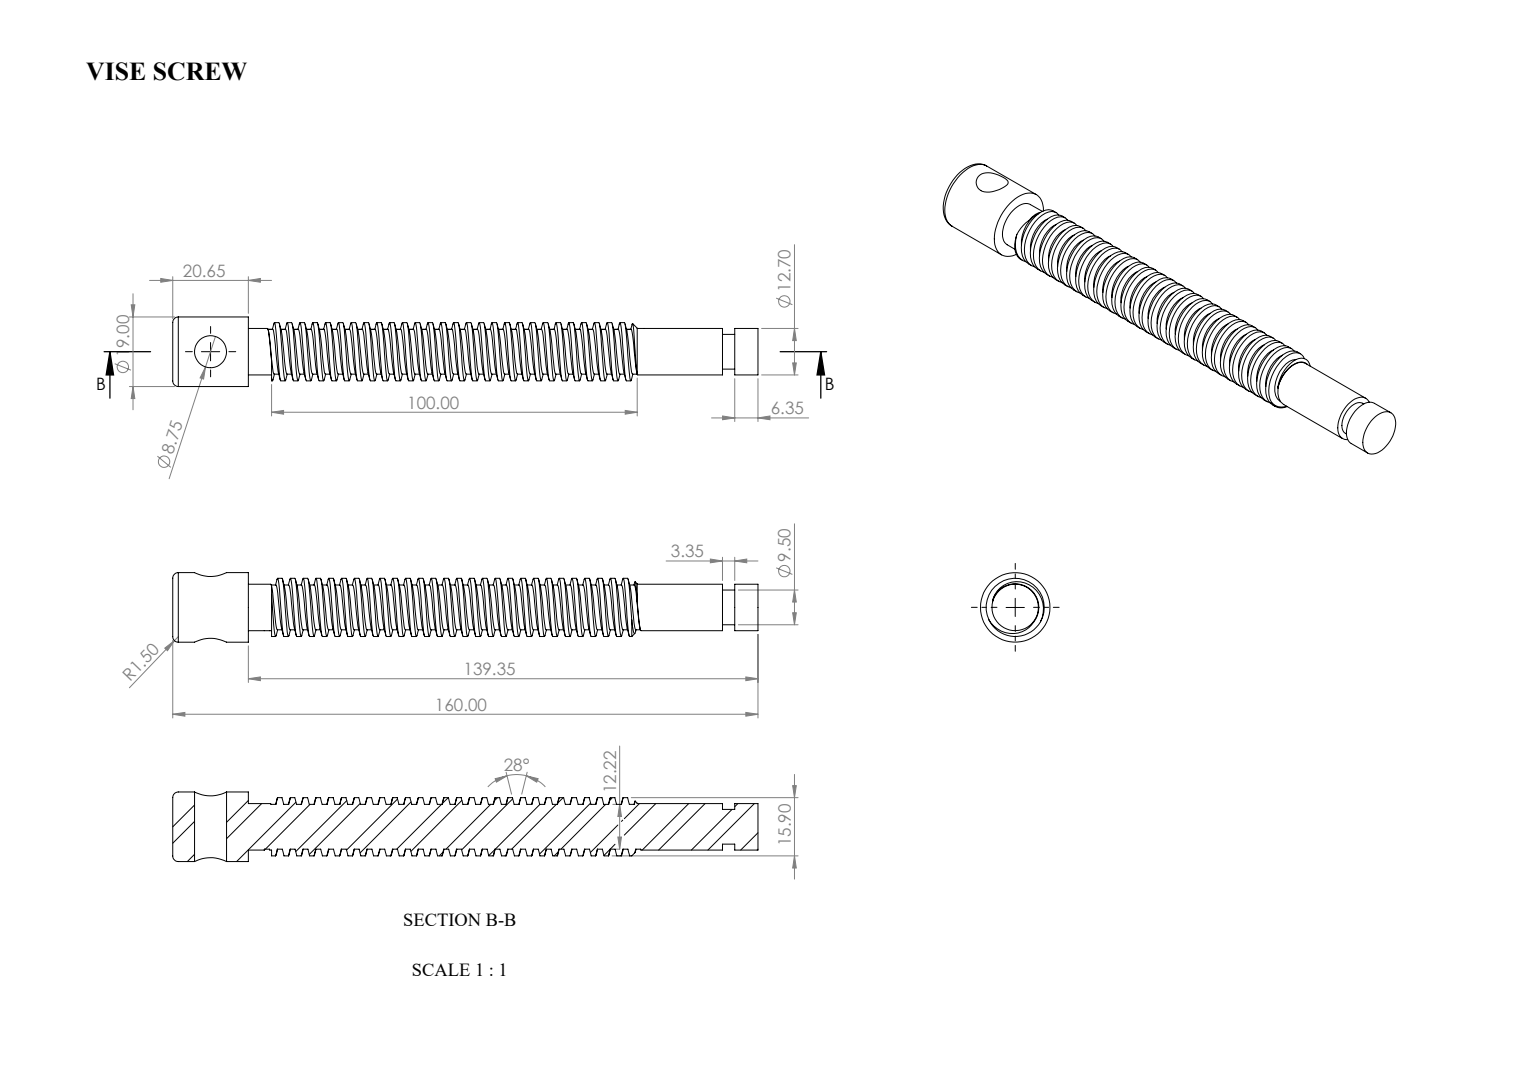
ISO-10303-21;
HEADER;
FILE_DESCRIPTION (('STEP AP214'),
    '1' );
FILE_NAME ('1.2 Vise Screw.step',
    '2026-10-06T08:51:13',
    ( '' ),
    ( '' ),
    'SwSTEP 2.0',
    'SolidWorks 2021',
    '' );
FILE_SCHEMA (( 'AUTOMOTIVE_DESIGN' ));
ENDSEC;

DATA;
#1=DIRECTION ( 'NONE',  ( 0.000000000000000000, 0.000000000000000000, 1.000000000000000000 ) ) ;
#6=CARTESIAN_POINT ( 'NONE',  ( 116.7245968585647660, -1.637169565754160949, 6.109999999999997655 ) ) ;
#17=CARTESIAN_POINT ( 'NONE',  ( 37.77126352523144703, 4.472830434245839371, 4.472830434245842035 ) ) ;
#23=CARTESIAN_POINT ( 'NONE',  ( 26.89126352523144092, -4.472830434245839371, -4.472830434245839371 ) ) ;
#50=ORIENTED_EDGE ( 'NONE', *, *, #36159, .F. ) ;
#52=ORIENTED_EDGE ( 'NONE', *, *, #60548, .T. ) ;
#55=CARTESIAN_POINT ( 'NONE',  ( 47.30793019189811588, -6.109999999999998543, 1.637169565754158507 ) ) ;
#68=DIRECTION ( 'NONE',  ( 0.000000000000000000, 0.000000000000000000, 1.000000000000000000 ) ) ;
#91=CARTESIAN_POINT ( 'NONE',  ( 109.2870968585647944, 3.054999999999997939, 5.291415217122920289 ) ) ;
#136=CARTESIAN_POINT ( 'NONE',  ( 29.66209685856477307, -5.291415217122919401, 3.054999999999998384 ) ) ;
#155=CARTESIAN_POINT ( 'NONE',  ( 124.5420968585647756, 5.291415217122923842, -3.054999999999996163 ) ) ;
#165=CARTESIAN_POINT ( 'NONE',  ( 54.62086038379622721, -6.884901960086286188, 3.974999999999997424 ) ) ;
#172=CARTESIAN_POINT ( 'NONE',  ( 48.25000000000000000, -9.735942053221458872E-16, 7.950000000000000178 ) ) ;
#180=CARTESIAN_POINT ( 'NONE',  ( 41.27126352523144703, 4.472830434245839371, 4.472830434245842035 ) ) ;
#194=CARTESIAN_POINT ( 'NONE',  ( 82.25043019189810423, 3.055000000000002824, -5.291415217122919401 ) ) ;
#203=CARTESIAN_POINT ( 'NONE',  ( 53.43293019189810167, 1.637169565754156508, 6.110000000000000320 ) ) ;
#229=AXIS2_PLACEMENT_3D ( 'NONE', #59966, #127341, #70166 ) ;
#238=CARTESIAN_POINT ( 'NONE',  ( 79.97459685856478018, 1.637169565754164280, -6.109999999999996767 ) ) ;
#269=CARTESIAN_POINT ( 'NONE',  ( 28.58376352523143993, -6.110000000000001208, -3.741295971395164515E-16 ) ) ;
#304=CARTESIAN_POINT ( 'NONE',  ( 97.49586038379624142, -3.974999999999998312, -6.884901960086286188 ) ) ;
#308=CARTESIAN_POINT ( 'NONE',  ( 0.000000000000000000, 0.000000000000000000, 7.950000000000000178 ) ) ;
#322=CARTESIAN_POINT ( 'NONE',  ( 56.34959685856478018, 6.109999999999997655, 1.637169565754163836 ) ) ;
#328=CARTESIAN_POINT ( 'NONE',  ( 32.30836038379622721, 7.949999999999996625, 2.130196079827431088 ) ) ;
#329=CARTESIAN_POINT ( 'NONE',  ( 83.68750000000000000, -5.819803920172573974, 5.819803920172573086 ) ) ;
#354=CARTESIAN_POINT ( 'NONE',  ( 81.45419371712955581, 6.884901960086283523, 3.975000000000002753 ) ) ;
#359=CARTESIAN_POINT ( 'NONE',  ( 73.62500000000000000, -7.950000000000000178, -4.867971026610729436E-16 ) ) ;
#371=CARTESIAN_POINT ( 'NONE',  ( 62.12543019189810423, 5.291415217122919401, 3.055000000000002824 ) ) ;
#390=CARTESIAN_POINT ( 'NONE',  ( 65.91709685856477563, 3.054999999999998828, 5.291415217122922066 ) ) ;
#419=CARTESIAN_POINT ( 'NONE',  ( 105.7870968585647802, 3.054999999999997495, 5.291415217122919401 ) ) ;
#439=CARTESIAN_POINT ( 'NONE',  ( 54.03752705046288440, -9.735942053221456900E-16, 7.949999999999998401 ) ) ;
#440=CARTESIAN_POINT ( 'NONE',  ( 59.14169371712955581, -2.130196079827424871, -7.949999999999998401 ) ) ;
#453=CARTESIAN_POINT ( 'NONE',  ( 53.81293019189810423, -1.637169565754159617, -6.110000000000001208 ) ) ;
#458=CARTESIAN_POINT ( 'NONE',  ( 93.47959685856476142, 6.109999999999999432, 1.637169565754164280 ) ) ;
#476=CARTESIAN_POINT ( 'NONE',  ( 121.2454301918981230, -5.291415217122918513, -3.055000000000000160 ) ) ;
#522=CARTESIAN_POINT ( 'NONE',  ( 111.0583603837961988, -7.949999999999997513, -2.130196079827425759 ) ) ;
#533=CARTESIAN_POINT ( 'NONE',  ( 0.000000000000000000, 0.000000000000000000, 7.950000000000000178 ) ) ;
#542=CARTESIAN_POINT ( 'NONE',  ( 106.7504301918981184, 3.055000000000002824, -5.291415217122919401 ) ) ;
#555=EDGE_CURVE ( 'NONE', #94937, #79882, #33614, .T. ) ;
#567=CARTESIAN_POINT ( 'NONE',  ( 94.50043019189810423, -3.055000000000002380, 5.291415217122920289 ) ) ;
#576=DIRECTION ( 'NONE',  ( -1.000000000000000000, 0.000000000000000000, -0.000000000000000000 ) ) ;
#578=CARTESIAN_POINT ( 'NONE',  ( 83.47459685856478018, 1.637169565754164058, -6.109999999999996767 ) ) ;
#631=CARTESIAN_POINT ( 'NONE',  ( 126.5837635252314612, -6.110000000000001208, -3.741295971395164515E-16 ) ) ;
#635=EDGE_CURVE ( 'NONE', #24706, #53682, #47379, .T. ) ;
#656=CARTESIAN_POINT ( 'NONE',  ( 108.1416937171295700, -2.130196079827424871, -7.949999999999998401 ) ) ;
#668=CARTESIAN_POINT ( 'NONE',  ( 87.12043019189812298, 3.055000000000002380, -5.291415217122917625 ) ) ;
#669=CARTESIAN_POINT ( 'NONE',  ( 8.372623110723612427, -8.651829453956585425, -3.925649932724890157 ) ) ;
#670=CARTESIAN_POINT ( 'NONE',  ( 99.10002705046288440, 5.819803920172570422, 5.819803920172575751 ) ) ;
#710=CARTESIAN_POINT ( 'NONE',  ( 99.29166666666667140, 3.975000000000003642, -6.884901960086285300 ) ) ;
#734=CARTESIAN_POINT ( 'NONE',  ( 120.8962635252314186, 4.472830434245840259, -4.472830434245839371 ) ) ;
#743=CARTESIAN_POINT ( 'NONE',  ( 113.9537635252314516, -6.109999999999998543, -3.741295971395162543E-16 ) ) ;
#750=CARTESIAN_POINT ( 'NONE',  ( 97.97916666666667140, -7.950000000000000178, 2.130196079827424427 ) ) ;
#753=CARTESIAN_POINT ( 'NONE',  ( 36.16709685856476852, -3.055000000000000160, -5.291415217122921177 ) ) ;
#759=CARTESIAN_POINT ( 'NONE',  ( 31.41209685856477662, 5.291415217122921177, -3.054999999999994831 ) ) ;
#762=LINE ( 'NONE', #89924, #117300 ) ;
#763=ORIENTED_EDGE ( 'NONE', *, *, #55111, .T. ) ;
#776=CARTESIAN_POINT ( 'NONE',  ( 82.03752705046288440, -9.735942053221456900E-16, 7.949999999999998401 ) ) ;
#792=CARTESIAN_POINT ( 'NONE',  ( 43.51626352523143737, -4.472830434245838482, 4.472830434245838482 ) ) ;
#800=CARTESIAN_POINT ( 'NONE',  ( 0.000000000000000000, 9.735942053221458872E-16, -7.950000000000000178 ) ) ;
#806=CARTESIAN_POINT ( 'NONE',  ( 0.000000000000000000, 0.000000000000000000, 0.000000000000000000 ) ) ;
#815=CARTESIAN_POINT ( 'NONE',  ( 36.24586038379622011, 3.974999999999996980, 6.884901960086287964 ) ) ;
#830=CARTESIAN_POINT ( 'NONE',  ( 108.1204301918981230, 3.055000000000002380, -5.291415217122917625 ) ) ;
#841=CARTESIAN_POINT ( 'NONE',  ( 121.4583333333333286, 3.974999999999997424, 6.884901960086288852 ) ) ;
#867=CARTESIAN_POINT ( 'NONE',  ( 28.78709685856477307, 3.054999999999997939, 5.291415217122920289 ) ) ;
#886=CARTESIAN_POINT ( 'NONE',  ( 121.9170968585647756, 3.054999999999998828, 5.291415217122922066 ) ) ;
#898=CARTESIAN_POINT ( 'NONE',  ( 46.16252705046289151, 7.949999999999998401, 1.460391307983218338E-15 ) ) ;
#905=CARTESIAN_POINT ( 'NONE',  ( 46.64583333333332860, 2.130196079827431976, -7.949999999999999289 ) ) ;
#914=CARTESIAN_POINT ( 'NONE',  ( 37.91709685856477563, 3.054999999999998828, 5.291415217122922066 ) ) ;
#937=CARTESIAN_POINT ( 'NONE',  ( 60.43293019189810877, 1.637169565754156508, 6.110000000000000320 ) ) ;
#942=VERTEX_POINT ( 'NONE', #42174 ) ;
#968=CARTESIAN_POINT ( 'NONE',  ( 78.22459685856478018, -1.637169565754160949, 6.109999999999997655 ) ) ;
#992=CARTESIAN_POINT ( 'NONE',  ( 29.02126352523143282, -4.472830434245838482, -4.472830434245840259 ) ) ;
#1018=CARTESIAN_POINT ( 'NONE',  ( 27.97916666666666430, -7.950000000000000178, 2.130196079827424427 ) ) ;
#1036=CARTESIAN_POINT ( 'NONE',  ( 112.4166666666666714, -6.884901960086287076, -3.975000000000000977 ) ) ;
#1039=CARTESIAN_POINT ( 'NONE',  ( 54.74543019189812298, -5.291415217122919401, -3.055000000000000604 ) ) ;
#1066=CARTESIAN_POINT ( 'NONE',  ( 71.82919371712957002, -3.975000000000001865, 6.884901960086284411 ) ) ;
#1072=CARTESIAN_POINT ( 'NONE',  ( 77.27083333333332860, -7.949999999999999289, -2.130196079827426203 ) ) ;
#1084=CARTESIAN_POINT ( 'NONE',  ( 66.79209685856477563, -5.291415217122921177, 3.054999999999999272 ) ) ;
#1091=CARTESIAN_POINT ( 'NONE',  ( 43.00000000000000000, 0.000000000000000000, -7.950000000000000178 ) ) ;
#1103=CARTESIAN_POINT ( 'NONE',  ( 68.54209685856477563, 5.291415217122923842, -3.054999999999996163 ) ) ;
#1119=DIRECTION ( 'NONE',  ( -0.000000000000000000, 1.000000000000000000, -0.000000000000000000 ) ) ;
#1129=CARTESIAN_POINT ( 'NONE',  ( 36.53752705046288440, -9.735942053221456900E-16, 7.949999999999998401 ) ) ;
#1135=CARTESIAN_POINT ( 'NONE',  ( 101.8495968585647802, 6.109999999999996767, 1.637169565754163836 ) ) ;
#1158=CARTESIAN_POINT ( 'NONE',  ( 51.18793019189810423, 6.110000000000002984, -1.637169565754156730 ) ) ;
#1164=CARTESIAN_POINT ( 'NONE',  ( 94.64626352523143282, -4.472830434245840259, 4.472830434245838482 ) ) ;
#1208=CARTESIAN_POINT ( 'NONE',  ( 7.036110477784782269, 9.049368983927246646, -2.898830007922127638 ) ) ;
#1231=CARTESIAN_POINT ( 'NONE',  ( 107.1208603837962272, -6.884901960086286188, 3.974999999999997424 ) ) ;
#1249=EDGE_LOOP ( 'NONE', ( #141134, #120202, #46022, #17961 ) ) ;
#1251=CARTESIAN_POINT ( 'NONE',  ( 93.33376352523144703, 6.110000000000001208, 1.122388791418549305E-15 ) ) ;
#1275=CARTESIAN_POINT ( 'NONE',  ( 87.93793019189809002, -6.110000000000001208, 1.637169565754158951 ) ) ;
#1287=CARTESIAN_POINT ( 'NONE',  ( 85.22459685856478018, -1.637169565754160949, 6.109999999999997655 ) ) ;
#1312=ORIENTED_EDGE ( 'NONE', *, *, #63406, .T. ) ;
#1316=CARTESIAN_POINT ( 'NONE',  ( 57.39169371712954160, 2.130196079827421762, 7.950000000000000178 ) ) ;
#1337=CARTESIAN_POINT ( 'NONE',  ( 121.0420968585647756, 5.291415217122923842, -3.054999999999996163 ) ) ;
#1338=DIRECTION ( 'NONE',  ( 0.000000000000000000, 0.000000000000000000, 1.000000000000000000 ) ) ;
#1365=CARTESIAN_POINT ( 'NONE',  ( 85.80793019189810877, -6.109999999999999432, 1.637169565754158507 ) ) ;
#1382=EDGE_LOOP ( 'NONE', ( #65288, #6857, #101636, #67565 ) ) ;
#1411=CARTESIAN_POINT ( 'NONE',  ( 109.7916666666666572, 3.975000000000003642, -6.884901960086285300 ) ) ;
#1416=CARTESIAN_POINT ( 'NONE',  ( 106.1458333333333144, 2.130196079827431976, -7.949999999999999289 ) ) ;
#1421=CARTESIAN_POINT ( 'NONE',  ( 14.47120107780393461, 9.396302691346770430, -1.425124364721372938 ) ) ;
#1430=CARTESIAN_POINT ( 'NONE',  ( 128.6829301918981230, -1.637169565754158951, -6.109999999999998543 ) ) ;
#1437=CARTESIAN_POINT ( 'NONE',  ( 87.14169371712955581, -2.130196079827424871, -7.949999999999998401 ) ) ;
#1442=CARTESIAN_POINT ( 'NONE',  ( 119.8754301918981184, -5.291415217122920289, -3.055000000000001492 ) ) ;
#1451=CARTESIAN_POINT ( 'NONE',  ( 113.2245968585647944, -1.637169565754160949, 6.109999999999997655 ) ) ;
#1459=CARTESIAN_POINT ( 'NONE',  ( 37.18793019189810423, 6.110000000000002984, -1.637169565754156730 ) ) ;
#1460=VERTEX_POINT ( 'NONE', #38433 ) ;
#1498=CARTESIAN_POINT ( 'NONE',  ( 50.07876352523145158, -7.482591942790325086E-16, 6.109999999999998543 ) ) ;
#1529=CARTESIAN_POINT ( 'NONE',  ( 108.2662635252314374, 4.472830434245839371, -4.472830434245839371 ) ) ;
#1540=CARTESIAN_POINT ( 'NONE',  ( 120.7291666666666572, 7.950000000000001954, -2.130196079827421762 ) ) ;
#1553=LINE ( 'NONE', #66865, #24099 ) ;
#1589=CARTESIAN_POINT ( 'NONE',  ( 118.7087635252314328, -7.482591942790329030E-16, 6.110000000000001208 ) ) ;
#1599=CARTESIAN_POINT ( 'NONE',  ( 47.62086038379622011, -6.884901960086286188, 3.974999999999997424 ) ) ;
#1605=CARTESIAN_POINT ( 'NONE',  ( 49.70833333333332860, -3.974999999999999201, -6.884901960086287964 ) ) ;
#1613=CARTESIAN_POINT ( 'NONE',  ( 34.41709685856476852, 3.054999999999998828, 5.291415217122922066 ) ) ;
#1619=CARTESIAN_POINT ( 'NONE',  ( 0.000000000000000000, 0.000000000000000000, 0.000000000000000000 ) ) ;
#1636=CARTESIAN_POINT ( 'NONE',  ( 61.89126352523144448, -4.472830434245839371, -4.472830434245839371 ) ) ;
#1661=CARTESIAN_POINT ( 'NONE',  ( 77.05793019189812298, 6.110000000000000320, -1.637169565754156064 ) ) ;
#1672=CARTESIAN_POINT ( 'NONE',  ( 28.99999999999999645, 0.000000000000000000, -7.950000000000000178 ) ) ;
#1680=ORIENTED_EDGE ( 'NONE', *, *, #101176, .T. ) ;
#1688=CARTESIAN_POINT ( 'NONE',  ( 43.39169371712955581, 2.130196079827421762, 7.950000000000000178 ) ) ;
#1703=ORIENTED_EDGE ( 'NONE', *, *, #44316, .T. ) ;
#1734=CARTESIAN_POINT ( 'NONE',  ( 57.37043019189810877, -3.055000000000001936, 5.291415217122918513 ) ) ;
#1744=CARTESIAN_POINT ( 'NONE',  ( 0.000000000000000000, 0.000000000000000000, 0.000000000000000000 ) ) ;
#1756=CARTESIAN_POINT ( 'NONE',  ( 79.41252705046289861, -7.949999999999998401, -4.867971026610728450E-16 ) ) ;
#1761=CARTESIAN_POINT ( 'NONE',  ( 71.58333333333332860, 6.884901960086290629, -3.974999999999994316 ) ) ;
#1763=FACE_OUTER_BOUND ( 'NONE', #86238, .T. ) ;
#1771=CARTESIAN_POINT ( 'NONE',  ( 69.41709685856477563, 3.054999999999998828, 5.291415217122922066 ) ) ;
#1791=CARTESIAN_POINT ( 'NONE',  ( 54.83376352523143282, 6.110000000000001208, 1.122388791418549305E-15 ) ) ;
#1805=CARTESIAN_POINT ( 'NONE',  ( 112.6625270504628986, 7.949999999999998401, 1.460391307983218338E-15 ) ) ;
#1818=CARTESIAN_POINT ( 'NONE',  ( 105.2037635252314516, 6.109999999999998543, 1.122388791418548911E-15 ) ) ;
#1831=CARTESIAN_POINT ( 'NONE',  ( 68.52083333333334281, 7.949999999999998401, 2.130196079827431532 ) ) ;
#1844=CARTESIAN_POINT ( 'NONE',  ( 50.60459685856477563, 1.637169565754164946, -6.109999999999999432 ) ) ;
#1851=CARTESIAN_POINT ( 'NONE',  ( 91.87543019189811844, -5.291415217122920289, -3.055000000000001492 ) ) ;
#1888=ORIENTED_EDGE ( 'NONE', *, *, #141103, .F. ) ;
#1920=EDGE_CURVE ( 'NONE', #135518, #143125, #124680, .T. ) ;
#1922=CARTESIAN_POINT ( 'NONE',  ( 101.1416937171295558, -2.130196079827424871, -7.949999999999999289 ) ) ;
#1939=CARTESIAN_POINT ( 'NONE',  ( 98.72959685856478984, -6.110000000000000320, -1.637169565754161393 ) ) ;
#1961=CARTESIAN_POINT ( 'NONE',  ( 86.33376352523144703, 6.110000000000001208, 1.122388791418549305E-15 ) ) ;
#1972=CARTESIAN_POINT ( 'NONE',  ( 87.70376352523146579, 6.109999999999998543, 1.122388791418548911E-15 ) ) ;
#1991=DIRECTION ( 'NONE',  ( 0.000000000000000000, -1.000000000000000000, 0.000000000000000000 ) ) ;
#2017=CARTESIAN_POINT ( 'NONE',  ( 116.6000270504628844, 5.819803920172570422, 5.819803920172575751 ) ) ;
#2028=CARTESIAN_POINT ( 'NONE',  ( 93.89583333333331439, -2.130196079827427091, 7.949999999999998401 ) ) ;
#2033=CARTESIAN_POINT ( 'NONE',  ( 122.0629301918980900, 1.637169565754157174, 6.110000000000002984 ) ) ;
#2064=ORIENTED_EDGE ( 'NONE', *, *, #98737, .F. ) ;
#2065=CARTESIAN_POINT ( 'NONE',  ( 80.99543019189810877, 5.291415217122917625, 3.055000000000002380 ) ) ;
#2098=CARTESIAN_POINT ( 'NONE',  ( 48.64169371712955581, -2.130196079827424871, -7.949999999999998401 ) ) ;
#2114=CARTESIAN_POINT ( 'NONE',  ( 96.81250000000000000, 5.819803920172571310, 5.819803920172575751 ) ) ;
#2116=ORIENTED_EDGE ( 'NONE', *, *, #54667, .F. ) ;
#2140=CARTESIAN_POINT ( 'NONE',  ( 26.51360224591381254, -6.350000000000003197, -3.888253587292850026E-16 ) ) ;
#2144=CARTESIAN_POINT ( 'NONE',  ( 121.1879301918980900, 6.110000000000002984, -1.637169565754156730 ) ) ;
#2154=CARTESIAN_POINT ( 'NONE',  ( 110.8912635252314658, -4.472830434245839371, -4.472830434245839371 ) ) ;
#2198=CARTESIAN_POINT ( 'NONE',  ( 45.70376352523145158, 6.109999999999998543, 1.122388791418548911E-15 ) ) ;
#2241=CARTESIAN_POINT ( 'NONE',  ( 113.5162635252314516, -4.472830434245839371, 4.472830434245839371 ) ) ;
#2275=ADVANCED_FACE ( 'NONE', ( #85148 ), #118488, .T. ) ;
#2284=CARTESIAN_POINT ( 'NONE',  ( 115.7708333333333428, -7.949999999999999289, -2.130196079827426203 ) ) ;
#2287=EDGE_LOOP ( 'NONE', ( #43419, #11730, #83774, #11348 ) ) ;
#2302=CARTESIAN_POINT ( 'NONE',  ( 121.4795968585647614, 6.109999999999999432, 1.637169565754164280 ) ) ;
#2311=( BOUNDED_CURVE ( )  B_SPLINE_CURVE ( 2, ( #39603, #115666, #105528, #93242, #94650, #136027, #27256, #59233, #25841, #92508, #83089, #81688, #71504 ),
 .UNSPECIFIED., .F., .T. ) 
 B_SPLINE_CURVE_WITH_KNOTS ( ( 3, 2, 2, 2, 2, 2, 3 ),
 ( 0.4333333333333334592, 0.4361111111111112271, 0.4388888888888889950, 0.4416666666666667629, 0.4444444444444445308, 0.4472222222222223542, 0.4500000000000001221 ),
 .UNSPECIFIED. ) 
 CURVE ( )  GEOMETRIC_REPRESENTATION_ITEM ( )  RATIONAL_B_SPLINE_CURVE ( ( 0.9999999999999986677, 0.9659258262890696445, 1.000000000000000000, 0.9659258262890683122, 1.000000000000000000, 0.9659258262890683122, 1.000000000000000000, 0.9659258262890683122, 1.000000000000000000, 0.9659258262890683122, 1.000000000000000000, 0.9659258262890669799, 1.000000000000001332 ) ) 
 REPRESENTATION_ITEM ( '' )  );
#2314=CARTESIAN_POINT ( 'NONE',  ( 49.51669371712955581, 7.950000000000001066, -2.130196079827421318 ) ) ;
#2319=CARTESIAN_POINT ( 'NONE',  ( 44.75000000000000000, -9.735942053221458872E-16, 7.950000000000000178 ) ) ;
#2320=ORIENTED_EDGE ( 'NONE', *, *, #17735, .T. ) ;
#2328=CARTESIAN_POINT ( 'NONE',  ( 39.37543019189809712, -5.291415217122920289, -3.055000000000001492 ) ) ;
#2352=CARTESIAN_POINT ( 'NONE',  ( 56.78709685856478728, 3.054999999999997495, 5.291415217122919401 ) ) ;
#2359=DIRECTION ( 'NONE',  ( 0.000000000000000000, 0.000000000000000000, 1.000000000000000000 ) ) ;
#2380=CARTESIAN_POINT ( 'NONE',  ( 75.16209685856478018, -5.291415217122919401, 3.054999999999997939 ) ) ;
#2381=ORIENTED_EDGE ( 'NONE', *, *, #99244, .F. ) ;
#2412=CARTESIAN_POINT ( 'NONE',  ( 29.45876352523143993, 0.000000000000000000, -6.110000000000001208 ) ) ;
#2421=CARTESIAN_POINT ( 'NONE',  ( 119.6625270504628986, 7.949999999999998401, 1.460391307983218338E-15 ) ) ;
#2426=EDGE_LOOP ( 'NONE', ( #135710, #51906, #114340, #8829, #67737 ) ) ;
#2465=CARTESIAN_POINT ( 'NONE',  ( 58.09959685856477307, -6.109999999999998543, -1.637169565754160727 ) ) ;
#2481=CARTESIAN_POINT ( 'NONE',  ( 26.90113084065429305, -4.940037651924031437, -4.143603795564325232 ) ) ;
#2486=CARTESIAN_POINT ( 'NONE',  ( 75.03752705046288440, -9.735942053221456900E-16, 7.949999999999998401 ) ) ;
#2490=CARTESIAN_POINT ( 'NONE',  ( 72.31250000000001421, 5.819803920172571310, 5.819803920172575751 ) ) ;
#2501=CARTESIAN_POINT ( 'NONE',  ( 70.29209685856477563, -5.291415217122921177, 3.054999999999999272 ) ) ;
#2514=CARTESIAN_POINT ( 'NONE',  ( 85.43750000000001421, 5.819803920172574863, -5.819803920172573086 ) ) ;
#2520=CIRCLE ( 'NONE', #229, 9.500000000000001776 ) ;
#2524=CARTESIAN_POINT ( 'NONE',  ( 53.22959685856475431, -6.110000000000000320, -1.637169565754161393 ) ) ;
#2544=CARTESIAN_POINT ( 'NONE',  ( 113.1000270504628986, 5.819803920172570422, 5.819803920172575751 ) ) ;
#2553=CARTESIAN_POINT ( 'NONE',  ( 37.99586038379622011, -3.974999999999998312, -6.884901960086286188 ) ) ;
#2560=CARTESIAN_POINT ( 'NONE',  ( 103.5995968585647802, -6.109999999999997655, -1.637169565754160283 ) ) ;
#2581=VERTEX_POINT ( 'NONE', #136876 ) ;
#2591=CARTESIAN_POINT ( 'NONE',  ( 57.75043019189809712, 3.055000000000002824, -5.291415217122919401 ) ) ;
#2595=CARTESIAN_POINT ( 'NONE',  ( 89.68793019189810423, 6.110000000000002984, -1.637169565754156730 ) ) ;
#2609=CARTESIAN_POINT ( 'NONE',  ( 126.0579301918981230, 6.110000000000001208, -1.637169565754156286 ) ) ;
#2613=VERTEX_POINT ( 'NONE', #63634 ) ;
#2642=CARTESIAN_POINT ( 'NONE',  ( 6.853232476907147763, 9.118190832583858096, -2.677290879925327882 ) ) ;
#2667=CARTESIAN_POINT ( 'NONE',  ( 101.5791937171295558, 3.975000000000002753, -6.884901960086283523 ) ) ;
#2684=CARTESIAN_POINT ( 'NONE',  ( 91.87543019189811844, -5.291415217122920289, -3.055000000000001492 ) ) ;
#2712=EDGE_LOOP ( 'NONE', ( #25102, #63841, #133635, #9677 ) ) ;
#2714=CARTESIAN_POINT ( 'NONE',  ( 79.04209685856477563, 5.291415217122923842, -3.054999999999996163 ) ) ;
#2730=CARTESIAN_POINT ( 'NONE',  ( 80.84959685856478018, 6.109999999999996767, 1.637169565754163836 ) ) ;
#2756=VERTEX_POINT ( 'NONE', #31688 ) ;
#2776=VECTOR ( 'NONE', #87300, 1000.000000000000000 ) ;
#2778=CARTESIAN_POINT ( 'NONE',  ( 93.75000000000000000, -9.735942053221458872E-16, 7.950000000000000178 ) ) ;
#2780=CARTESIAN_POINT ( 'NONE',  ( 120.0212635252314328, -4.472830434245838482, -4.472830434245840259 ) ) ;
#2806=VERTEX_POINT ( 'NONE', #65149 ) ;
#2840=CARTESIAN_POINT ( 'NONE',  ( 104.5416666666666714, -3.975000000000002753, 6.884901960086286188 ) ) ;
#2859=CARTESIAN_POINT ( 'NONE',  ( 88.79166666666665719, 3.975000000000003642, -6.884901960086285300 ) ) ;
#2869=CARTESIAN_POINT ( 'NONE',  ( 12.99795884586121630, 8.843280219809532383, 3.474951431101239052 ) ) ;
#2876=EDGE_CURVE ( 'NONE', #29769, #74867, #20924, .T. ) ;
#2888=CARTESIAN_POINT ( 'NONE',  ( 110.6879301918981184, 6.110000000000002984, -1.637169565754156730 ) ) ;
#2899=CARTESIAN_POINT ( 'NONE',  ( 100.2454301918981230, -5.291415217122918513, -3.055000000000000160 ) ) ;
#2903=CARTESIAN_POINT ( 'NONE',  ( 97.25000000000000000, -9.735942053221458872E-16, 7.950000000000000178 ) ) ;
#2912=CARTESIAN_POINT ( 'NONE',  ( 33.16209685856478018, -5.291415217122919401, 3.054999999999997939 ) ) ;
#2922=CYLINDRICAL_SURFACE ( 'NONE', #121136, 7.950000000000000178 ) ;
#2945=CARTESIAN_POINT ( 'NONE',  ( 39.28709685856478018, 3.054999999999997495, 5.291415217122919401 ) ) ;
#2957=ADVANCED_FACE ( 'NONE', ( #89724 ), #33255, .T. ) ;
#2964=AXIS2_PLACEMENT_3D ( 'NONE', #136803, #81749, #16423 ) ;
#2981=CARTESIAN_POINT ( 'NONE',  ( 107.9745968585647660, 1.637169565754164280, -6.109999999999997655 ) ) ;
#3024=CARTESIAN_POINT ( 'NONE',  ( 126.2740448710917320, -7.159498723440732348, 0.5736663686628497016 ) ) ;
#3031=CARTESIAN_POINT ( 'NONE',  ( 120.4374999999999858, 5.819803920172573974, -5.819803920172572198 ) ) ;
#3042=CARTESIAN_POINT ( 'NONE',  ( 108.9379301918981042, -6.110000000000001208, 1.637169565754158951 ) ) ;
#3053=CARTESIAN_POINT ( 'NONE',  ( 43.10002705046289861, 5.819803920172570422, 5.819803920172574863 ) ) ;
#3060=CARTESIAN_POINT ( 'NONE',  ( 37.60416666666666430, 2.130196079827422206, 7.950000000000001954 ) ) ;
#3072=CARTESIAN_POINT ( 'NONE',  ( 42.72959685856476142, -6.110000000000000320, -1.637169565754161393 ) ) ;
#3095=CARTESIAN_POINT ( 'NONE',  ( 59.99543019189810877, 5.291415217122916737, 3.055000000000001936 ) ) ;
#3118=CARTESIAN_POINT ( 'NONE',  ( 69.62043019189812298, 3.055000000000001936, -5.291415217122916737 ) ) ;
#3177=ORIENTED_EDGE ( 'NONE', *, *, #116429, .F. ) ;
#3196=CARTESIAN_POINT ( 'NONE',  ( 55.91209685856478018, 5.291415217122922066, -3.054999999999995275 ) ) ;
#3214=CARTESIAN_POINT ( 'NONE',  ( 117.9583333333333286, 3.974999999999997424, 6.884901960086288852 ) ) ;
#3215=CARTESIAN_POINT ( 'NONE',  ( 76.49586038379621300, -3.974999999999998312, -6.884901960086286188 ) ) ;
#3221=CARTESIAN_POINT ( 'NONE',  ( 63.27083333333332860, -7.949999999999999289, -2.130196079827426203 ) ) ;
#3223=EDGE_CURVE ( 'NONE', #134670, #143282, #108231, .T. ) ;
#3232=CARTESIAN_POINT ( 'NONE',  ( 64.60459685856477563, 1.637169565754164946, -6.109999999999999432 ) ) ;
#3284=CARTESIAN_POINT ( 'NONE',  ( 106.6620968585647802, -5.291415217122919401, 3.054999999999997939 ) ) ;
#3305=CARTESIAN_POINT ( 'NONE',  ( 50.31293019189809712, -1.637169565754159617, -6.110000000000001208 ) ) ;
#3320=CARTESIAN_POINT ( 'NONE',  ( 128.5370968585647802, -3.054999999999999272, -5.291415217122919401 ) ) ;
#3373=CARTESIAN_POINT ( 'NONE',  ( 106.6833603837962272, -2.130196079827426203, 7.949999999999997513 ) ) ;
#3384=CARTESIAN_POINT ( 'NONE',  ( 34.24999999999998579, -9.735942053221458872E-16, 7.950000000000000178 ) ) ;
#3392=CARTESIAN_POINT ( 'NONE',  ( 96.10459685856477563, 1.637169565754164946, -6.109999999999999432 ) ) ;
#3410=CYLINDRICAL_SURFACE ( 'NONE', #2964, 7.950000000000000178 ) ;
#3414=CARTESIAN_POINT ( 'NONE',  ( 81.52126352523141861, -4.472830434245839371, -4.472830434245840259 ) ) ;
#3428=CARTESIAN_POINT ( 'NONE',  ( 80.41209685856479439, 5.291415217122921177, -3.054999999999994831 ) ) ;
#3476=CARTESIAN_POINT ( 'NONE',  ( 114.6254301918981042, 5.291415217122919401, 3.055000000000002824 ) ) ;
#3526=CARTESIAN_POINT ( 'NONE',  ( 104.6875000000000000, -5.819803920172573974, 5.819803920172573086 ) ) ;
#3535=CARTESIAN_POINT ( 'NONE',  ( 30.82876352523145158, 0.000000000000000000, -6.109999999999999432 ) ) ;
#3551=EDGE_CURVE ( 'NONE', #5049, #29421, #95878, .T. ) ;
#3554=CARTESIAN_POINT ( 'NONE',  ( 90.68750000000001421, -5.819803920172573086, 5.819803920172572198 ) ) ;
#3560=CARTESIAN_POINT ( 'NONE',  ( 11.47410930353643188, 8.505905029784415206, -4.231274956823338762 ) ) ;
#3566=CARTESIAN_POINT ( 'NONE',  ( 126.3365831057324300, 6.972970002233967790, -1.493943918826199813 ) ) ;
#3580=CARTESIAN_POINT ( 'NONE',  ( 114.3337635252314470, 6.110000000000001208, 1.122388791418549305E-15 ) ) ;
#3590=CYLINDRICAL_SURFACE ( 'NONE', #51191, 7.950000000000000178 ) ;
#3591=CARTESIAN_POINT ( 'NONE',  ( 107.9745968585647660, 1.637169565754164058, -6.109999999999996767 ) ) ;
#3627=CARTESIAN_POINT ( 'NONE',  ( 36.37043019189811588, -3.055000000000001492, 5.291415217122917625 ) ) ;
#3664=CARTESIAN_POINT ( 'NONE',  ( 100.3912635252314516, -4.472830434245839371, -4.472830434245839371 ) ) ;
#3704=CARTESIAN_POINT ( 'NONE',  ( 125.6998834332835884, -5.108784383707307697, 5.835737331199903899 ) ) ;
#3705=CARTESIAN_POINT ( 'NONE',  ( 28.80836038379622011, 7.949999999999996625, 2.130196079827431088 ) ) ;
#3711=CARTESIAN_POINT ( 'NONE',  ( 124.3750000000000000, 7.950000000000000178, 1.460391307983218535E-15 ) ) ;
#3724=CARTESIAN_POINT ( 'NONE',  ( 111.2712635252314612, 4.472830434245839371, 4.472830434245842035 ) ) ;
#3734=CARTESIAN_POINT ( 'NONE',  ( 40.62086038379622721, -6.884901960086286188, 3.974999999999997424 ) ) ;
#3740=CARTESIAN_POINT ( 'NONE',  ( 33.66666666666666430, 6.884901960086285300, 3.975000000000003642 ) ) ;
#3751=CARTESIAN_POINT ( 'NONE',  ( 32.66709685856476852, -3.055000000000000160, -5.291415217122921177 ) ) ;
#3769=CARTESIAN_POINT ( 'NONE',  ( 46.28709685856477307, 3.054999999999997495, 5.291415217122919401 ) ) ;
#3794=CARTESIAN_POINT ( 'NONE',  ( 67.28709685856478018, 3.054999999999997495, 5.291415217122919401 ) ) ;
#3796=ORIENTED_EDGE ( 'NONE', *, *, #47475, .T. ) ;
#3801=( BOUNDED_CURVE ( )  B_SPLINE_CURVE ( 2, ( #73847, #139119, #84047, #128243, #39077, #118020, #38371, #83303, #127513, #18725, #116634, #107176, #52093 ),
 .UNSPECIFIED., .F., .F. ) 
 B_SPLINE_CURVE_WITH_KNOTS ( ( 3, 2, 2, 2, 2, 2, 3 ),
 ( 0.9333333333333333481, 0.9361111111111111160, 0.9388888888888888840, 0.9416666666666666519, 0.9444444444444444198, 0.9472222222222221877, 0.9499999999999999556 ),
 .UNSPECIFIED. ) 
 CURVE ( )  GEOMETRIC_REPRESENTATION_ITEM ( )  RATIONAL_B_SPLINE_CURVE ( ( 1.000000000000000000, 0.9659258262890683122, 1.000000000000000000, 0.9659258262890683122, 1.000000000000000000, 0.9659258262890683122, 1.000000000000000000, 0.9659258262890683122, 1.000000000000000000, 0.9659258262890683122, 1.000000000000000000, 0.9659258262890683122, 1.000000000000000000 ) ) 
 REPRESENTATION_ITEM ( '' )  );
#3875=CARTESIAN_POINT ( 'NONE',  ( 47.30793019189811588, -6.109999999999999432, 1.637169565754158507 ) ) ;
#3895=CARTESIAN_POINT ( 'NONE',  ( 118.2500000000000000, -9.735942053221458872E-16, 7.950000000000000178 ) ) ;
#3896=CARTESIAN_POINT ( 'NONE',  ( 78.97502705046288440, -5.819803920172572198, 5.819803920172572198 ) ) ;
#3901=CARTESIAN_POINT ( 'NONE',  ( 62.10416666666665719, 2.130196079827422206, 7.950000000000001954 ) ) ;
#3910=CARTESIAN_POINT ( 'NONE',  ( 20.65000000000000213, 0.000000000000000000, 0.000000000000000000 ) ) ;
#3911=CARTESIAN_POINT ( 'NONE',  ( 52.20876352523143282, -7.482591942790329030E-16, 6.110000000000001208 ) ) ;
#3958=CARTESIAN_POINT ( 'NONE',  ( 90.47459685856479439, 1.637169565754164280, -6.109999999999996767 ) ) ;
#3964=ORIENTED_EDGE ( 'NONE', *, *, #68959, .F. ) ;
#3967=CARTESIAN_POINT ( 'NONE',  ( 67.79166666666667140, 3.975000000000003642, -6.884901960086285300 ) ) ;
#3977=CARTESIAN_POINT ( 'NONE',  ( 42.58376352523143993, -6.110000000000001208, -3.741295971395164515E-16 ) ) ;
#3980=EDGE_CURVE ( 'NONE', #95449, #98838, #35803, .T. ) ;
#4053=CARTESIAN_POINT ( 'NONE',  ( 100.5583603837962272, -7.949999999999997513, -2.130196079827425759 ) ) ;
#4067=CARTESIAN_POINT ( 'NONE',  ( 95.66709685856477563, -3.055000000000000160, -5.291415217122921177 ) ) ;
#4089=CARTESIAN_POINT ( 'NONE',  ( 87.20876352523143282, -7.482591942790329030E-16, 6.110000000000001208 ) ) ;
#4098=CARTESIAN_POINT ( 'NONE',  ( 73.26626352523143737, 4.472830434245839371, -4.472830434245838482 ) ) ;
#4104=ORIENTED_EDGE ( 'NONE', *, *, #109273, .T. ) ;
#4122=CARTESIAN_POINT ( 'NONE',  ( 69.35002705046288440, -5.819803920172573086, -5.819803920172573086 ) ) ;
#4138=CARTESIAN_POINT ( 'NONE',  ( 77.58376352523144703, -6.110000000000001208, -3.741295971395164515E-16 ) ) ;
#4145=CARTESIAN_POINT ( 'NONE',  ( 122.6462635252314328, -4.472830434245840259, 4.472830434245838482 ) ) ;
#4182=DIRECTION ( 'NONE',  ( -1.000000000000000000, -0.000000000000000000, -0.000000000000000000 ) ) ;
#4212=CARTESIAN_POINT ( 'NONE',  ( 128.4125270504628986, -7.949999999999998401, -4.867971026610728450E-16 ) ) ;
#4214=CARTESIAN_POINT ( 'NONE',  ( 48.78752705046289151, 0.000000000000000000, -7.949999999999998401 ) ) ;
#4225=CARTESIAN_POINT ( 'NONE',  ( 95.20833333333334281, -3.974999999999999201, -6.884901960086287964 ) ) ;
#4230=CARTESIAN_POINT ( 'NONE',  ( 14.69272197276067438, 9.496641765041323069, -0.2911197889769509550 ) ) ;
#4239=CARTESIAN_POINT ( 'NONE',  ( 125.6139270598129229, -2.020146860515199094, -7.575422191809951578 ) ) ;
#4253=CARTESIAN_POINT ( 'NONE',  ( 115.3545968585647614, -1.637169565754161615, 6.110000000000000320 ) ) ;
#4263=CARTESIAN_POINT ( 'NONE',  ( 108.9954301918981088, 5.291415217122916737, 3.055000000000001936 ) ) ;
#4306=CARTESIAN_POINT ( 'NONE',  ( 35.20376352523143737, 6.109999999999998543, 1.122388791418548911E-15 ) ) ;
#4346=CARTESIAN_POINT ( 'NONE',  ( 99.95376352523145158, -6.109999999999999432, -3.741295971395163529E-16 ) ) ;
#4347=( BOUNDED_CURVE ( )  B_SPLINE_CURVE ( 2, ( #79809, #45732, #91370, #89902, #35579, #111675, #90650, #123986, #58776, #134147, #134884, #24648, #80489 ),
 .UNSPECIFIED., .F., .T. ) 
 B_SPLINE_CURVE_WITH_KNOTS ( ( 3, 2, 2, 2, 2, 2, 3 ),
 ( 0.2499999999999999445, 0.2527777777777777124, 0.2555555555555554803, 0.2583333333333333037, 0.2611111111111110716, 0.2638888888888888395, 0.2666666666666666075 ),
 .UNSPECIFIED. ) 
 CURVE ( )  GEOMETRIC_REPRESENTATION_ITEM ( )  RATIONAL_B_SPLINE_CURVE ( ( 1.000000000000000666, 0.9659258262890676461, 1.000000000000000000, 0.9659258262890683122, 1.000000000000000000, 0.9659258262890683122, 1.000000000000000000, 0.9659258262890683122, 1.000000000000000000, 0.9659258262890683122, 1.000000000000000000, 0.9659258262890689783, 0.9999999999999993339 ) ) 
 REPRESENTATION_ITEM ( '' )  );
#4397=CARTESIAN_POINT ( 'NONE',  ( 120.2916666666666714, 3.975000000000003642, -6.884901960086285300 ) ) ;
#4407=CARTESIAN_POINT ( 'NONE',  ( 115.3545968585647614, -1.637169565754161615, 6.110000000000000320 ) ) ;
#4415=CARTESIAN_POINT ( 'NONE',  ( 39.01669371712955581, 7.950000000000001066, -2.130196079827421318 ) ) ;
#4420=CARTESIAN_POINT ( 'NONE',  ( 35.12499999999999289, -7.950000000000000178, -4.867971026610729436E-16 ) ) ;
#4431=CARTESIAN_POINT ( 'NONE',  ( 29.16709685856476497, -3.055000000000000160, -5.291415217122921177 ) ) ;
#4446=ADVANCED_FACE ( 'NONE', ( #75744 ), #131544, .T. ) ;
#4454=CARTESIAN_POINT ( 'NONE',  ( 47.01626352523143026, -4.472830434245839371, 4.472830434245839371 ) ) ;
#4488=CARTESIAN_POINT ( 'NONE',  ( 64.51626352523145158, -4.472830434245838482, 4.472830434245838482 ) ) ;
#4500=DIRECTION ( 'NONE',  ( -1.000000000000000000, -0.000000000000000000, -0.000000000000000000 ) ) ;
#4565=CARTESIAN_POINT ( 'NONE',  ( 44.68293019189811588, -1.637169565754159173, -6.109999999999999432 ) ) ;
#4577=CARTESIAN_POINT ( 'NONE',  ( 0.000000000000000000, 9.735942053221458872E-16, -7.950000000000000178 ) ) ;
#4588=CARTESIAN_POINT ( 'NONE',  ( 117.8125000000000000, 5.819803920172571310, 5.819803920172576639 ) ) ;
#4589=CARTESIAN_POINT ( 'NONE',  ( 69.35002705046287019, -5.819803920172572198, -5.819803920172572198 ) ) ;
#4590=DIRECTION ( 'NONE',  ( 0.000000000000000000, 0.000000000000000000, 1.000000000000000000 ) ) ;
#4594=CARTESIAN_POINT ( 'NONE',  ( 68.52083333333334281, 7.949999999999999289, 2.130196079827431532 ) ) ;
#4602=CARTESIAN_POINT ( 'NONE',  ( 52.64626352523142572, -4.472830434245840259, 4.472830434245839371 ) ) ;
#4631=CARTESIAN_POINT ( 'NONE',  ( 124.1833603837965967, -2.130196079832207712, 7.949999999997237055 ) ) ;
#4652=( BOUNDED_CURVE ( )  B_SPLINE_CURVE ( 2, ( #38213, #28043, #96128, #82427, #41054, #73685, #104880, #115713, #117858, #115003, #50509, #126612, #27302 ),
 .UNSPECIFIED., .F., .T. ) 
 B_SPLINE_CURVE_WITH_KNOTS ( ( 3, 2, 2, 2, 2, 2, 3 ),
 ( 0.09999999999998596123, 0.1027777777777660745, 0.1055555555555461877, 0.1083333333333263149, 0.1111111111111064281, 0.1138888888888865414, 0.1166666666666666685 ),
 .UNSPECIFIED. ) 
 CURVE ( )  GEOMETRIC_REPRESENTATION_ITEM ( )  RATIONAL_B_SPLINE_CURVE ( ( 1.000000000000172307, 0.9659258262888960056, 1.000000000000000000, 0.9659258262890683122, 1.000000000000000000, 0.9659258262890683122, 1.000000000000000000, 0.9659258262890683122, 1.000000000000000000, 0.9659258262890683122, 1.000000000000000000, 0.9659258262890683122, 1.000000000000000000 ) ) 
 REPRESENTATION_ITEM ( '' )  );
#4659=CARTESIAN_POINT ( 'NONE',  ( 0.000000000000000000, 0.000000000000000000, 0.000000000000000000 ) ) ;
#4663=VERTEX_POINT ( 'NONE', #439 ) ;
#4665=CARTESIAN_POINT ( 'NONE',  ( 94.55793019189810877, 6.110000000000000320, -1.637169565754156064 ) ) ;
#4692=CARTESIAN_POINT ( 'NONE',  ( 46.95876352523143993, 0.000000000000000000, -6.110000000000001208 ) ) ;
#4728=EDGE_CURVE ( 'NONE', #32830, #113567, #80243, .T. ) ;
#4736=CARTESIAN_POINT ( 'NONE',  ( 96.03752705046289861, -9.735942053221456900E-16, 7.949999999999998401 ) ) ;
#4741=CARTESIAN_POINT ( 'NONE',  ( 70.78709685856478018, 3.054999999999997939, 5.291415217122920289 ) ) ;
#4772=CARTESIAN_POINT ( 'NONE',  ( 91.66252705046288440, 7.949999999999998401, 1.460391307983218338E-15 ) ) ;
#4788=CARTESIAN_POINT ( 'NONE',  ( 88.95876352523143282, 0.000000000000000000, -6.110000000000001208 ) ) ;
#4810=CARTESIAN_POINT ( 'NONE',  ( 86.18793019189811844, 6.110000000000002984, -1.637169565754156730 ) ) ;
#4816=EDGE_CURVE ( 'NONE', #92449, #102139, #93884, .T. ) ;
#4834=CARTESIAN_POINT ( 'NONE',  ( 65.02083333333332860, 7.949999999999998401, 2.130196079827431532 ) ) ;
#4835=ADVANCED_FACE ( 'NONE', ( #42928 ), #74853, .T. ) ;
#4874=CARTESIAN_POINT ( 'NONE',  ( 73.50043019189811844, -3.055000000000002380, 5.291415217122920289 ) ) ;
#4879=CARTESIAN_POINT ( 'NONE',  ( 106.0212635252314612, -4.472830434245838482, -4.472830434245840259 ) ) ;
#4948=CARTESIAN_POINT ( 'NONE',  ( 32.57876352523145158, -7.482591942790327058E-16, 6.109999999999999432 ) ) ;
#4965=CARTESIAN_POINT ( 'NONE',  ( 94.04166666666665719, -3.975000000000002753, 6.884901960086286188 ) ) ;
#4981=CARTESIAN_POINT ( 'NONE',  ( 126.5282371893278537, 6.759817336840661106, 1.509802715116372207 ) ) ;
#4992=CARTESIAN_POINT ( 'NONE',  ( 114.9170968585647756, 3.054999999999998828, 5.291415217122922066 ) ) ;
#5000=DIRECTION ( 'NONE',  ( 0.000000000000000000, 0.000000000000000000, 1.000000000000000000 ) ) ;
#5003=CARTESIAN_POINT ( 'NONE',  ( 107.6829301918981088, -1.637169565754158951, -6.109999999999998543 ) ) ;
#5013=VERTEX_POINT ( 'NONE', #56687 ) ;
#5025=EDGE_LOOP ( 'NONE', ( #10485, #114535, #24984, #19673 ) ) ;
#5049=VERTEX_POINT ( 'NONE', #66803 ) ;
#5058=CARTESIAN_POINT ( 'NONE',  ( 34.32876352523143737, 0.000000000000000000, -6.109999999999998543 ) ) ;
#5093=CARTESIAN_POINT ( 'NONE',  ( 100.5370968585647802, -3.054999999999999272, -5.291415217122919401 ) ) ;
#5146=CARTESIAN_POINT ( 'NONE',  ( 118.3958333333333286, -2.130196079827427091, 7.949999999999999289 ) ) ;
#5160=CARTESIAN_POINT ( 'NONE',  ( 115.5004301918981042, -3.055000000000002380, 5.291415217122920289 ) ) ;
#5163=CARTESIAN_POINT ( 'NONE',  ( 106.1000270504628986, 5.819803920172570422, 5.819803920172575751 ) ) ;
#5169=CARTESIAN_POINT ( 'NONE',  ( 34.20419371712955581, -6.884901960086285300, -3.975000000000000089 ) ) ;
#5173=EDGE_LOOP ( 'NONE', ( #99987, #77473 ) ) ;
#5174=CARTESIAN_POINT ( 'NONE',  ( 38.91666666666665719, -6.884901960086287076, -3.975000000000000977 ) ) ;
#5189=FACE_OUTER_BOUND ( 'NONE', #140682, .T. ) ;
#5192=CARTESIAN_POINT ( 'NONE',  ( 27.70876352523143993, -7.482591942790329030E-16, 6.110000000000001208 ) ) ;
#5193=B_SPLINE_CURVE_WITH_KNOTS ( 'NONE', 3,
 ( #47167, #70333, #57298, #3560, #125387, #12320, #124657, #102217, #134861, #69600, #114479, #48527, #58017, #1421, #90622, #102919, #47856, #4230, #134124, #24627, #80467, #92728, #136967, #113785, #35555, #122499, #46435, #25333, #2869, #91346, #26072, #23175, #14474, #113052, #135556, #13725 ),
 .UNSPECIFIED., .F., .F.,
 ( 4, 2, 2, 2, 2, 2, 2, 2, 2, 2, 2, 2, 2, 2, 2, 2, 2, 4 ),
 ( 0.01387570424127936193, 0.01474184239350130252, 0.01560798054572324310, 0.01647411869794518369, 0.01734025685016712254, 0.01820639500238906486, 0.01907253315461100718, 0.01993867130683294603, 0.02037174038294391545, 0.02080480945905488488, 0.02167094761127682373, 0.02253708576349876258, 0.02340322391572070490, 0.02426936206794264722, 0.02513550022016458607, 0.02600163837238652492, 0.02686777652460846724, 0.02773391467683040609 ),
 .UNSPECIFIED. ) ;
#5205=CARTESIAN_POINT ( 'NONE',  ( 51.18793019189810423, 6.110000000000002984, -1.637169565754156730 ) ) ;
#5207=EDGE_LOOP ( 'NONE', ( #68193, #57456, #33431, #64376 ) ) ;
#5216=CARTESIAN_POINT ( 'NONE',  ( 49.64126352523145158, 4.472830434245836706, 4.472830434245840259 ) ) ;
#5226=CARTESIAN_POINT ( 'NONE',  ( 60.16252705046289151, 7.949999999999998401, 1.460391307983218338E-15 ) ) ;
#5247=CARTESIAN_POINT ( 'NONE',  ( 64.66209685856478018, -5.291415217122919401, 3.054999999999997939 ) ) ;
#5249=( BOUNDED_CURVE ( )  B_SPLINE_CURVE ( 2, ( #85438, #105068, #60907, #49997, #94180, #17343, #97004, #128962, #18019, #19487, #73185, #84072, #129666 ),
 .UNSPECIFIED., .F., .T. ) 
 B_SPLINE_CURVE_WITH_KNOTS ( ( 3, 2, 2, 2, 2, 2, 3 ),
 ( 0.4833333333333333370, 0.4861111111111111049, 0.4888888888888888729, 0.4916666666666666408, 0.4944444444444444642, 0.4972222222222222321, 0.5000000000000000000 ),
 .UNSPECIFIED. ) 
 CURVE ( )  GEOMETRIC_REPRESENTATION_ITEM ( )  RATIONAL_B_SPLINE_CURVE ( ( 1.000000000000000000, 0.9659258262890683122, 1.000000000000000000, 0.9659258262890683122, 1.000000000000000000, 0.9659258262890683122, 1.000000000000000000, 0.9659258262890683122, 1.000000000000000000, 0.9659258262890683122, 1.000000000000000000, 0.9659258262890683122, 1.000000000000000000 ) ) 
 REPRESENTATION_ITEM ( '' )  );
#5326=CARTESIAN_POINT ( 'NONE',  ( 45.41209685856478728, 5.291415217122922066, -3.054999999999995275 ) ) ;
#5349=CARTESIAN_POINT ( 'NONE',  ( 62.49586038379623432, -3.974999999999998312, -6.884901960086286188 ) ) ;
#5354=CARTESIAN_POINT ( 'NONE',  ( 68.22916666666665719, 7.950000000000001954, -2.130196079827421762 ) ) ;
#5358=ADVANCED_FACE ( 'NONE', ( #38992 ), #48441, .F. ) ;
#5364=CARTESIAN_POINT ( 'NONE',  ( 57.75043019189809712, 3.055000000000002824, -5.291415217122919401 ) ) ;
#5387=CARTESIAN_POINT ( 'NONE',  ( 111.4958603837962272, -3.974999999999998312, -6.884901960086286188 ) ) ;
#5416=CARTESIAN_POINT ( 'NONE',  ( 90.91209685856478018, 5.291415217122921177, -3.054999999999994831 ) ) ;
#5428=CARTESIAN_POINT ( 'NONE',  ( 0.000000000000000000, 0.000000000000000000, 7.950000000000000178 ) ) ;
#5439=CARTESIAN_POINT ( 'NONE',  ( 44.33376352523143993, 6.110000000000001208, 1.122388791418549305E-15 ) ) ;
#5481=CARTESIAN_POINT ( 'NONE',  ( 96.08333333333332860, 6.884901960086290629, -3.974999999999994316 ) ) ;
#5494=CARTESIAN_POINT ( 'NONE',  ( 78.66209685856479439, -5.291415217122919401, 3.054999999999998384 ) ) ;
#5496=CARTESIAN_POINT ( 'NONE',  ( 75.03752705046288440, -9.735942053221456900E-16, 7.949999999999998401 ) ) ;
#5513=CARTESIAN_POINT ( 'NONE',  ( 122.1416937171300390, -2.130196079821051303, -7.950000000003678124 ) ) ;
#5518=CARTESIAN_POINT ( 'NONE',  ( 95.16252705046289861, 7.949999999999998401, 1.460391307983218338E-15 ) ) ;
#5519=CARTESIAN_POINT ( 'NONE',  ( 71.72916666666665719, 7.950000000000001954, -2.130196079827421762 ) ) ;
#5528=DIRECTION ( 'NONE',  ( -1.000000000000000000, -0.000000000000000000, -0.000000000000000000 ) ) ;
#5536=CARTESIAN_POINT ( 'NONE',  ( 85.60459685856478984, 1.637169565754164946, -6.109999999999999432 ) ) ;
#5554=CARTESIAN_POINT ( 'NONE',  ( 59.18749999999998579, -5.819803920172573974, 5.819803920172573086 ) ) ;
#5559=CARTESIAN_POINT ( 'NONE',  ( 70.14626352523143282, -4.472830434245840259, 4.472830434245839371 ) ) ;
#5574=CARTESIAN_POINT ( 'NONE',  ( 33.47502705046289151, -5.819803920172573086, 5.819803920172573086 ) ) ;
#5612=CARTESIAN_POINT ( 'NONE',  ( 69.56293019189810423, 1.637169565754157174, 6.110000000000002984 ) ) ;
#5618=CARTESIAN_POINT ( 'NONE',  ( 105.7295968585647898, -6.110000000000000320, -1.637169565754161393 ) ) ;
#5676=CARTESIAN_POINT ( 'NONE',  ( 153.6500000000000057, 5.817072295949924468E-16, -4.749999999999997335 ) ) ;
#5685=CARTESIAN_POINT ( 'NONE',  ( 118.6416937171295700, -2.130196079827424871, -7.949999999999999289 ) ) ;
#5699=CARTESIAN_POINT ( 'NONE',  ( 83.68750000000000000, -5.819803920172573086, 5.819803920172572198 ) ) ;
#5711=CARTESIAN_POINT ( 'NONE',  ( 126.6276089467980057, 6.187174973706484060, 2.918809472323000254 ) ) ;
#5723=CARTESIAN_POINT ( 'NONE',  ( 103.2504301918981184, 3.055000000000002824, -5.291415217122919401 ) ) ;
#5731=CARTESIAN_POINT ( 'NONE',  ( 105.4954301918981230, 5.291415217122916737, 3.055000000000001936 ) ) ;
#5735=CARTESIAN_POINT ( 'NONE',  ( 122.2875270504628844, 0.000000000000000000, -7.949999999999998401 ) ) ;
#5759=CARTESIAN_POINT ( 'NONE',  ( 109.4329301918981088, 1.637169565754156508, 6.110000000000000320 ) ) ;
#5781=CARTESIAN_POINT ( 'NONE',  ( 35.34959685856478728, 6.109999999999996767, 1.637169565754163836 ) ) ;
#5810=CARTESIAN_POINT ( 'NONE',  ( 101.9954301918981230, 5.291415217122917625, 3.055000000000002380 ) ) ;
#5815=CARTESIAN_POINT ( 'NONE',  ( 0.000000000000000000, 0.000000000000000000, 7.950000000000000178 ) ) ;
#5865=CARTESIAN_POINT ( 'NONE',  ( 110.6666666666666572, 6.884901960086285300, 3.975000000000003642 ) ) ;
#5876=CARTESIAN_POINT ( 'NONE',  ( 111.8545968585647756, -1.637169565754161615, 6.110000000000000320 ) ) ;
#5878=DIRECTION ( 'NONE',  ( -1.000000000000000000, -0.000000000000000000, -0.000000000000000000 ) ) ;
#5884=CARTESIAN_POINT ( 'NONE',  ( 42.22502705046289861, 5.819803920172573086, -5.819803920172572198 ) ) ;
#5890=CARTESIAN_POINT ( 'NONE',  ( 37.89583333333332860, -2.130196079827427091, 7.949999999999999289 ) ) ;
#5898=CARTESIAN_POINT ( 'NONE',  ( 30.62543019189810423, 5.291415217122919401, 3.055000000000002824 ) ) ;
#5908=CARTESIAN_POINT ( 'NONE',  ( 58.77126352523142572, 4.472830434245839371, 4.472830434245842035 ) ) ;
#5916=CARTESIAN_POINT ( 'NONE',  ( 52.12043019189811588, 3.055000000000001936, -5.291415217122916737 ) ) ;
#5927=CARTESIAN_POINT ( 'NONE',  ( 59.72502705046289861, 5.819803920172573974, -5.819803920172573086 ) ) ;
#5948=CARTESIAN_POINT ( 'NONE',  ( 68.01626352523145158, -4.472830434245838482, 4.472830434245838482 ) ) ;
#6013=EDGE_CURVE ( 'NONE', #123729, #4663, #15151, .T. ) ;
#6021=CARTESIAN_POINT ( 'NONE',  ( 50.51626352523143737, -4.472830434245839371, 4.472830434245839371 ) ) ;
#6046=CARTESIAN_POINT ( 'NONE',  ( 69.64169371712952739, -2.130196079827424871, -7.949999999999999289 ) ) ;
#6052=CARTESIAN_POINT ( 'NONE',  ( 66.18749999999997158, -5.819803920172573086, 5.819803920172572198 ) ) ;
#6060=CARTESIAN_POINT ( 'NONE',  ( 57.89626352523144703, 4.472830434245840259, -4.472830434245839371 ) ) ;
#6084=CARTESIAN_POINT ( 'NONE',  ( 110.7666937171295558, -7.949999999999998401, 2.130196079827423983 ) ) ;
#6105=AXIS2_PLACEMENT_3D ( 'NONE', #94586, #114888, #27192 ) ;
#6108=CARTESIAN_POINT ( 'NONE',  ( 92.37043019189810877, -3.055000000000001492, 5.291415217122917625 ) ) ;
#6136=CARTESIAN_POINT ( 'NONE',  ( 41.12543019189809712, 5.291415217122919401, 3.055000000000002824 ) ) ;
#6171=CARTESIAN_POINT ( 'NONE',  ( 65.75000000000000000, -9.735942053221458872E-16, 7.950000000000000178 ) ) ;
#6177=CARTESIAN_POINT ( 'NONE',  ( 97.10416666666665719, 2.130196079827422206, 7.950000000000001954 ) ) ;
#6189=CARTESIAN_POINT ( 'NONE',  ( 72.82876352523145158, 0.000000000000000000, -6.109999999999999432 ) ) ;
#6211=CARTESIAN_POINT ( 'NONE',  ( 96.18336038379621300, -2.130196079827426203, 7.949999999999997513 ) ) ;
#6225=CARTESIAN_POINT ( 'NONE',  ( 88.52126352523143282, -4.472830434245839371, -4.472830434245840259 ) ) ;
#6243=CARTESIAN_POINT ( 'NONE',  ( 76.41709685856476142, 3.054999999999998828, 5.291415217122922066 ) ) ;
#6265=CARTESIAN_POINT ( 'NONE',  ( 53.74586038379622011, 3.974999999999996980, 6.884901960086287964 ) ) ;
#6294=CARTESIAN_POINT ( 'NONE',  ( 76.56293019189810423, 1.637169565754157174, 6.110000000000002984 ) ) ;
#6300=CARTESIAN_POINT ( 'NONE',  ( 106.3129301918981042, -1.637169565754159617, -6.110000000000001208 ) ) ;
#6306=CARTESIAN_POINT ( 'NONE',  ( 35.51669371712954870, 7.950000000000000178, -2.130196079827421318 ) ) ;
#6337=CARTESIAN_POINT ( 'NONE',  ( 14.47113640696344028, -9.396276906557130104, 1.425181317190020058 ) ) ;
#6338=EDGE_LOOP ( 'NONE', ( #110820, #8572 ) ) ;
#6352=CARTESIAN_POINT ( 'NONE',  ( 73.62500000000000000, -7.950000000000000178, -4.867971026610729436E-16 ) ) ;
#6367=CARTESIAN_POINT ( 'NONE',  ( 123.3083603837962130, 7.949999999999997513, 2.130196079827431088 ) ) ;
#6382=CARTESIAN_POINT ( 'NONE',  ( 82.66666666666667140, 6.884901960086285300, 3.975000000000003642 ) ) ;
#6406=CARTESIAN_POINT ( 'NONE',  ( 99.60459685856476142, 1.637169565754164946, -6.109999999999999432 ) ) ;
#6415=CARTESIAN_POINT ( 'NONE',  ( 91.20376352523145158, 6.109999999999998543, 1.122388791418548911E-15 ) ) ;
#6446=CARTESIAN_POINT ( 'NONE',  ( 112.9329301918981230, 1.637169565754156508, 6.110000000000000320 ) ) ;
#6451=CARTESIAN_POINT ( 'NONE',  ( 56.99999999999999289, 0.000000000000000000, -7.950000000000000178 ) ) ;
#6505=CARTESIAN_POINT ( 'NONE',  ( 99.80793019189812298, -6.109999999999999432, 1.637169565754158507 ) ) ;
#6523=VECTOR ( 'NONE', #94747, 1000.000000000000000 ) ;
#6557=CARTESIAN_POINT ( 'NONE',  ( 113.1458333333333144, 2.130196079827431976, -7.949999999999999289 ) ) ;
#6573=CARTESIAN_POINT ( 'NONE',  ( 103.8337635252314328, 6.110000000000001208, 1.122388791418549305E-15 ) ) ;
#6579=CARTESIAN_POINT ( 'NONE',  ( 83.78752705046288440, 0.000000000000000000, -7.949999999999998401 ) ) ;
#6583=CARTESIAN_POINT ( 'NONE',  ( 36.39169371712955581, 2.130196079827421762, 7.950000000000001066 ) ) ;
#6588=CARTESIAN_POINT ( 'NONE',  ( 26.08333333333333215, 6.884901960086290629, -3.974999999999994316 ) ) ;
#6596=CARTESIAN_POINT ( 'NONE',  ( 29.89626352523142927, 4.472830434245840259, -4.472830434245839371 ) ) ;
#6605=CARTESIAN_POINT ( 'NONE',  ( 55.41709685856477563, 3.054999999999998828, 5.291415217122922066 ) ) ;
#6607=CYLINDRICAL_SURFACE ( 'NONE', #107239, 7.950000000000000178 ) ;
#6612=CARTESIAN_POINT ( 'NONE',  ( 45.26626352523144448, 4.472830434245839371, -4.472830434245838482 ) ) ;
#6649=CARTESIAN_POINT ( 'NONE',  ( 52.84959685856478728, 6.109999999999996767, 1.637169565754163836 ) ) ;
#6657=CARTESIAN_POINT ( 'NONE',  ( 35.85416666666665719, -2.130196079827501698, -7.949999999999956657 ) ) ;
#6671=AXIS2_PLACEMENT_3D ( 'NONE', #142632, #32447, #86113 ) ;
#6674=CARTESIAN_POINT ( 'NONE',  ( 54.32919371712956291, -3.975000000000001865, 6.884901960086284411 ) ) ;
#6708=EDGE_LOOP ( 'NONE', ( #64672, #10605, #105317, #142378 ) ) ;
#6722=CARTESIAN_POINT ( 'NONE',  ( 47.89126352523143737, -4.472830434245839371, -4.472830434245839371 ) ) ;
#6749=CARTESIAN_POINT ( 'NONE',  ( 61.32919371712955581, -3.975000000000001865, 6.884901960086284411 ) ) ;
#6753=CARTESIAN_POINT ( 'NONE',  ( 54.37499999999999289, 7.950000000000000178, 1.460391307983218535E-15 ) ) ;
#6764=CARTESIAN_POINT ( 'NONE',  ( 53.95876352523143282, 0.000000000000000000, -6.110000000000001208 ) ) ;
#6768=EDGE_LOOP ( 'NONE', ( #133406, #49375, #138591, #88145 ) ) ;
#6778=ORIENTED_EDGE ( 'NONE', *, *, #65610, .T. ) ;
#6791=CARTESIAN_POINT ( 'NONE',  ( 74.43293019189810877, 1.637169565754156508, 6.110000000000000320 ) ) ;
#6808=CARTESIAN_POINT ( 'NONE',  ( 62.20419371712955581, -6.884901960086285300, -3.975000000000000089 ) ) ;
#6821=CARTESIAN_POINT ( 'NONE',  ( 92.51626352523145158, -4.472830434245838482, 4.472830434245838482 ) ) ;
#6825=CARTESIAN_POINT ( 'NONE',  ( 0.000000000000000000, 9.735942053221458872E-16, -7.950000000000000178 ) ) ;
#6849=CARTESIAN_POINT ( 'NONE',  ( 46.66709685856476852, -3.055000000000000160, -5.291415217122921177 ) ) ;
#6857=ORIENTED_EDGE ( 'NONE', *, *, #48779, .T. ) ;
#6900=CARTESIAN_POINT ( 'NONE',  ( 74.43293019189810877, 1.637169565754156730, 6.110000000000001208 ) ) ;
#6924=CARTESIAN_POINT ( 'NONE',  ( 94.72502705046289861, 5.819803920172573086, -5.819803920172572198 ) ) ;
#6931=CYLINDRICAL_SURFACE ( 'NONE', #14364, 7.950000000000000178 ) ;
#6937=CARTESIAN_POINT ( 'NONE',  ( 80.64626352523141861, -4.472830434245840259, 4.472830434245839371 ) ) ;
#6939=VECTOR ( 'NONE', #112574, 1000.000000000000000 ) ;
#6954=( BOUNDED_CURVE ( )  B_SPLINE_CURVE ( 2, ( #5496, #60666, #15632, #125891, #26563, #72260, #49773, #93953, #70806, #38868, #7644, #63512, #8337 ),
 .UNSPECIFIED., .F., .T. ) 
 B_SPLINE_CURVE_WITH_KNOTS ( ( 3, 2, 2, 2, 2, 2, 3 ),
 ( 0.5166666666666667185, 0.5194444444444444864, 0.5222222222222222543, 0.5250000000000000222, 0.5277777777777777901, 0.5305555555555555580, 0.5333333333333333259 ),
 .UNSPECIFIED. ) 
 CURVE ( )  GEOMETRIC_REPRESENTATION_ITEM ( )  RATIONAL_B_SPLINE_CURVE ( ( 1.000000000000000000, 0.9659258262890683122, 1.000000000000000000, 0.9659258262890683122, 1.000000000000000000, 0.9659258262890683122, 1.000000000000000000, 0.9659258262890683122, 1.000000000000000000, 0.9659258262890683122, 1.000000000000000000, 0.9659258262890683122, 1.000000000000000000 ) ) 
 REPRESENTATION_ITEM ( '' )  );
#6958=CARTESIAN_POINT ( 'NONE',  ( 71.75043019189811844, 3.055000000000002824, -5.291415217122919401 ) ) ;
#6973=CARTESIAN_POINT ( 'NONE',  ( 34.49586038379622011, -3.974999999999998312, -6.884901960086286188 ) ) ;
#7014=CARTESIAN_POINT ( 'NONE',  ( 74.66709685856476142, -3.055000000000000160, -5.291415217122921177 ) ) ;
#7023=CARTESIAN_POINT ( 'NONE',  ( 109.6670968585647756, -3.055000000000000160, -5.291415217122921177 ) ) ;
#7080=ADVANCED_FACE ( 'NONE', ( #20998 ), #10129, .T. ) ;
#7095=CARTESIAN_POINT ( 'NONE',  ( 121.5583603837962130, -7.949999999999997513, -2.130196079827425759 ) ) ;
#7109=CARTESIAN_POINT ( 'NONE',  ( 85.87500000000000000, 7.950000000000000178, 1.460391307983218535E-15 ) ) ;
#7133=CARTESIAN_POINT ( 'NONE',  ( 100.7712635252314328, 4.472830434245839371, 4.472830434245842035 ) ) ;
#7145=CARTESIAN_POINT ( 'NONE',  ( 92.66209685856479439, -5.291415217122919401, 3.054999999999997939 ) ) ;
#7153=DIRECTION ( 'NONE',  ( 0.2419218955996628451, 0.000000000000000000, 0.9702957262759975832 ) ) ;
#7169=CIRCLE ( 'NONE', #88245, 6.450000000000025047 ) ;
#7223=VERTEX_POINT ( 'NONE', #31827 ) ;
#7224=( BOUNDED_CURVE ( )  B_SPLINE_CURVE ( 2, ( #104630, #27067, #48129 ),
 .UNSPECIFIED., .F., .F. ) 
 B_SPLINE_CURVE_WITH_KNOTS ( ( 3, 3 ),
 ( 0.01429413858638482922, 0.01666666666666668031 ),
 .UNSPECIFIED. ) 
 CURVE ( )  GEOMETRIC_REPRESENTATION_ITEM ( )  RATIONAL_B_SPLINE_CURVE ( ( 0.9915083049239679092, 0.9708969037810285529, 1.000000000000000222 ) ) 
 REPRESENTATION_ITEM ( '' )  );
#7239=CARTESIAN_POINT ( 'NONE',  ( 93.09959685856479439, -6.109999999999998543, -1.637169565754160727 ) ) ;
#7244=VERTEX_POINT ( 'NONE', #75349 ) ;
#7256=B_SPLINE_CURVE_WITH_KNOTS ( 'NONE', 1,
 ( #2140, #46450 ),
 .UNSPECIFIED., .F., .F.,
 ( 2, 2 ),
 ( 0.8695652173913019922, 1.000000000000000000 ),
 .UNSPECIFIED. ) ;
#7297=CARTESIAN_POINT ( 'NONE',  ( 114.1666666666666714, 6.884901960086285300, 3.975000000000003642 ) ) ;
#7305=CARTESIAN_POINT ( 'NONE',  ( 89.81249999999998579, 5.819803920172571310, 5.819803920172576639 ) ) ;
#7313=CARTESIAN_POINT ( 'NONE',  ( 98.87543019189810423, -5.291415217122920289, -3.055000000000001492 ) ) ;
#7323=CARTESIAN_POINT ( 'NONE',  ( 28.37086038379622721, 6.884901960086289741, -3.974999999999993427 ) ) ;
#7327=CARTESIAN_POINT ( 'NONE',  ( 125.4170968585647756, 3.054999999999998828, 5.291415217122922066 ) ) ;
#7338=CARTESIAN_POINT ( 'NONE',  ( 126.0579301918981230, 6.110000000000000320, -1.637169565754156064 ) ) ;
#7351=CARTESIAN_POINT ( 'NONE',  ( 45.50043019189810423, -3.055000000000002380, 5.291415217122920289 ) ) ;
#7359=CARTESIAN_POINT ( 'NONE',  ( 36.37043019189811588, -3.055000000000001492, 5.291415217122917625 ) ) ;
#7371=CARTESIAN_POINT ( 'NONE',  ( 43.97502705046288440, -5.819803920172573086, 5.819803920172573086 ) ) ;
#7389=CARTESIAN_POINT ( 'NONE',  ( 53.43293019189810167, 1.637169565754156508, 6.110000000000000320 ) ) ;
#7423=CARTESIAN_POINT ( 'NONE',  ( 128.6829301918981230, -1.637169565754159173, -6.109999999999999432 ) ) ;
#7464=VECTOR ( 'NONE', #76490, 1000.000000000000227 ) ;
#7468=CARTESIAN_POINT ( 'NONE',  ( 38.99543019189812298, 5.291415217122917625, 3.055000000000002380 ) ) ;
#7496=CARTESIAN_POINT ( 'NONE',  ( 103.6208603837962272, -6.884901960086286188, 3.974999999999997424 ) ) ;
#7497=CARTESIAN_POINT ( 'NONE',  ( 63.80836038379621300, 7.949999999999997513, 2.130196079827431088 ) ) ;
#7501=CARTESIAN_POINT ( 'NONE',  ( 53.93750000000000000, 5.819803920172573974, -5.819803920172572198 ) ) ;
#7508=CARTESIAN_POINT ( 'NONE',  ( 45.93793019189810423, -6.110000000000001208, 1.637169565754158951 ) ) ;
#7509=AXIS2_PLACEMENT_3D ( 'NONE', #140453, #141159, #119394 ) ;
#7522=CARTESIAN_POINT ( 'NONE',  ( 0.000000000000000000, 9.735942053221458872E-16, -7.950000000000000178 ) ) ;
#7531=CARTESIAN_POINT ( 'NONE',  ( 79.97459685856479439, 1.637169565754164058, -6.109999999999996767 ) ) ;
#7562=CARTESIAN_POINT ( 'NONE',  ( 85.51626352523145158, -4.472830434245838482, 4.472830434245838482 ) ) ;
#7568=AXIS2_PLACEMENT_3D ( 'NONE', #129958, #64704, #100886 ) ;
#7589=CARTESIAN_POINT ( 'NONE',  ( 31.50043019189810423, -3.055000000000002380, 5.291415217122920289 ) ) ;
#7641=CARTESIAN_POINT ( 'NONE',  ( 73.26626352523143737, 4.472830434245839371, -4.472830434245839371 ) ) ;
#7644=CARTESIAN_POINT ( 'NONE',  ( 73.57919371712957002, 3.975000000000002753, -6.884901960086283523 ) ) ;
#7665=ORIENTED_EDGE ( 'NONE', *, *, #113714, .F. ) ;
#7670=CARTESIAN_POINT ( 'NONE',  ( 93.41252705046289861, -7.949999999999998401, -4.867971026610728450E-16 ) ) ;
#7683=CARTESIAN_POINT ( 'NONE',  ( 82.97959685856476142, 6.109999999999999432, 1.637169565754164280 ) ) ;
#7699=CARTESIAN_POINT ( 'NONE',  ( 60.50000000000000000, 0.000000000000000000, -7.950000000000000178 ) ) ;
#7703=CARTESIAN_POINT ( 'NONE',  ( 69.27126352523144703, 4.472830434245839371, 4.472830434245842035 ) ) ;
#7746=CARTESIAN_POINT ( 'NONE',  ( 27.00000000000001421, -7.661656307529537635, -1.660001620851698112 ) ) ;
#7758=CARTESIAN_POINT ( 'NONE',  ( 64.16709685856476142, -3.055000000000000160, -5.291415217122921177 ) ) ;
#7765=CARTESIAN_POINT ( 'NONE',  ( 103.6879301918981042, 6.110000000000002984, -1.637169565754156730 ) ) ;
#7811=CARTESIAN_POINT ( 'NONE',  ( 25.95876352523143638, 0.000000000000000000, -6.110000000000001208 ) ) ;
#7830=( BOUNDED_CURVE ( )  B_SPLINE_CURVE ( 2, ( #118274, #18981, #63246, #8075, #52317, #75513, #119683, #64627, #53775, #97976, #135604, #44331, #113113 ),
 .UNSPECIFIED., .F., .T. ) 
 B_SPLINE_CURVE_WITH_KNOTS ( ( 3, 2, 2, 2, 2, 2, 3 ),
 ( 0.4666666666666666741, 0.4694444444444444420, 0.4722222222222222099, 0.4749999999999999778, 0.4777777777777778012, 0.4805555555555555691, 0.4833333333333333370 ),
 .UNSPECIFIED. ) 
 CURVE ( )  GEOMETRIC_REPRESENTATION_ITEM ( )  RATIONAL_B_SPLINE_CURVE ( ( 1.000000000000000000, 0.9659258262890683122, 1.000000000000000000, 0.9659258262890683122, 1.000000000000000000, 0.9659258262890683122, 1.000000000000000000, 0.9659258262890683122, 1.000000000000000000, 0.9659258262890683122, 1.000000000000000000, 0.9659258262890683122, 1.000000000000000000 ) ) 
 REPRESENTATION_ITEM ( '' )  );
#7833=CARTESIAN_POINT ( 'NONE',  ( 121.1208603837962272, -6.884901960086286188, 3.974999999999997424 ) ) ;
#7872=CARTESIAN_POINT ( 'NONE',  ( 97.27126352523143282, 4.472830434245839371, 4.472830434245842035 ) ) ;
#7882=CARTESIAN_POINT ( 'NONE',  ( 96.59959685856476597, -6.109999999999997655, -1.637169565754160283 ) ) ;
#7898=VERTEX_POINT ( 'NONE', #71432 ) ;
#7958=EDGE_CURVE ( 'NONE', #82847, #49011, #65588, .T. ) ;
#7964=CARTESIAN_POINT ( 'NONE',  ( 87.84959685856476597, 6.109999999999997655, 1.637169565754163836 ) ) ;
#8015=CARTESIAN_POINT ( 'NONE',  ( 109.5000000000000000, 0.000000000000000000, -7.950000000000000178 ) ) ;
#8026=CARTESIAN_POINT ( 'NONE',  ( 100.9170968585647756, 3.054999999999998828, 5.291415217122922066 ) ) ;
#8035=CARTESIAN_POINT ( 'NONE',  ( 32.01669371712954160, 7.950000000000001066, -2.130196079827421318 ) ) ;
#8043=CARTESIAN_POINT ( 'NONE',  ( 29.43749999999998579, 5.819803920172573974, -5.819803920172572198 ) ) ;
#8047=FACE_OUTER_BOUND ( 'NONE', #96688, .T. ) ;
#8052=CARTESIAN_POINT ( 'NONE',  ( 124.4537635252314516, -6.109999999999998543, -3.741295971395162543E-16 ) ) ;
#8061=CARTESIAN_POINT ( 'NONE',  ( 45.79209685856476852, -5.291415217122921177, 3.054999999999999272 ) ) ;
#8067=CARTESIAN_POINT ( 'NONE',  ( 37.68293019189810167, -1.637169565754158951, -6.109999999999998543 ) ) ;
#8075=CARTESIAN_POINT ( 'NONE',  ( 79.85002705046289861, -5.819803920172573086, -5.819803920172573086 ) ) ;
#8080=EDGE_CURVE ( 'NONE', #24706, #128126, #40442, .T. ) ;
#8096=CARTESIAN_POINT ( 'NONE',  ( 60.14126352523143737, 4.472830434245835818, 4.472830434245840259 ) ) ;
#8131=CARTESIAN_POINT ( 'NONE',  ( 116.8704301918981230, -3.055000000000001936, 5.291415217122918513 ) ) ;
#8141=CARTESIAN_POINT ( 'NONE',  ( 75.62086038379622721, -6.884901960086286188, 3.974999999999997424 ) ) ;
#8171=CARTESIAN_POINT ( 'NONE',  ( 39.43293019189811588, 1.637169565754156730, 6.110000000000001208 ) ) ;
#8184=CARTESIAN_POINT ( 'NONE',  ( 82.81250000000000000, 5.819803920172571310, 5.819803920172576639 ) ) ;
#8192=CARTESIAN_POINT ( 'NONE',  ( 60.16252705046289151, 7.949999999999998401, 1.460391307983218338E-15 ) ) ;
#8198=CARTESIAN_POINT ( 'NONE',  ( 50.87499999999999289, 7.950000000000000178, 1.460391307983218535E-15 ) ) ;
#8208=CARTESIAN_POINT ( 'NONE',  ( 47.10459685856477563, 1.637169565754164946, -6.109999999999999432 ) ) ;
#8231=CARTESIAN_POINT ( 'NONE',  ( 70.05793019189812298, 6.110000000000000320, -1.637169565754156064 ) ) ;
#8244=CARTESIAN_POINT ( 'NONE',  ( 64.29166666666665719, 3.975000000000003642, -6.884901960086285300 ) ) ;
#8260=CARTESIAN_POINT ( 'NONE',  ( 85.95376352523145158, -6.109999999999998543, -3.741295971395162543E-16 ) ) ;
#8285=CARTESIAN_POINT ( 'NONE',  ( 40.10459685856476852, 1.637169565754164946, -6.109999999999999432 ) ) ;
#8304=CARTESIAN_POINT ( 'NONE',  ( 109.1625270504628986, 7.949999999999998401, 1.460391307983218338E-15 ) ) ;
#8336=CARTESIAN_POINT ( 'NONE',  ( 69.18293019189809456, -1.637169565754159173, -6.109999999999999432 ) ) ;
#8337=CARTESIAN_POINT ( 'NONE',  ( 73.28752705046288440, 0.000000000000000000, -7.949999999999998401 ) ) ;
#8342=ORIENTED_EDGE ( 'NONE', *, *, #67563, .T. ) ;
#8359=CARTESIAN_POINT ( 'NONE',  ( 86.70419371712955581, -6.884901960086285300, -3.975000000000000089 ) ) ;
#8373=CARTESIAN_POINT ( 'NONE',  ( 78.60459685856477563, 1.637169565754164946, -6.109999999999999432 ) ) ;
#8392=CARTESIAN_POINT ( 'NONE',  ( 73.79209685856477563, -5.291415217122921177, 3.054999999999999272 ) ) ;
#8407=ORIENTED_EDGE ( 'NONE', *, *, #95323, .T. ) ;
#8411=CARTESIAN_POINT ( 'NONE',  ( 128.1594355792471163, -6.349999999999998757, -1.701477371937630378 ) ) ;
#8414=AXIS2_PLACEMENT_3D ( 'NONE', #103982, #135929, #36607 ) ;
#8445=CARTESIAN_POINT ( 'NONE',  ( 67.52126352523144703, -4.472830434245838482, -4.472830434245840259 ) ) ;
#8452=CARTESIAN_POINT ( 'NONE',  ( 97.27126352523143282, 4.472830434245838482, 4.472830434245842035 ) ) ;
#8468=CARTESIAN_POINT ( 'NONE',  ( 126.4954301918981230, 5.291415217122916737, 3.055000000000001936 ) ) ;
#8483=CARTESIAN_POINT ( 'NONE',  ( 38.47916666666665719, -7.950000000000000178, 2.130196079827424427 ) ) ;
#8484=VERTEX_POINT ( 'NONE', #114402 ) ;
#8495=CARTESIAN_POINT ( 'NONE',  ( 32.95876352523143282, 0.000000000000000000, -6.110000000000001208 ) ) ;
#8516=CARTESIAN_POINT ( 'NONE',  ( 119.5166937171295558, 7.950000000000001066, -2.130196079827421318 ) ) ;
#8517=CARTESIAN_POINT ( 'NONE',  ( 27.00000000000000355, -4.083527258847093222, -4.862849486279972488 ) ) ;
#8519=PLANE ( 'NONE',  #60700 ) ;
#8538=CARTESIAN_POINT ( 'NONE',  ( 93.02083333333331439, 7.949999999999998401, 2.130196079827431532 ) ) ;
#8553=CARTESIAN_POINT ( 'NONE',  ( 105.4379301918981042, -6.110000000000001208, 1.637169565754158951 ) ) ;
#8563=CARTESIAN_POINT ( 'NONE',  ( 96.74543019189810877, -5.291415217122918513, -3.055000000000000160 ) ) ;
#8572=ORIENTED_EDGE ( 'NONE', *, *, #15620, .F. ) ;
#8614=CARTESIAN_POINT ( 'NONE',  ( 29.51626352523143737, -4.472830434245838482, 4.472830434245838482 ) ) ;
#8617=CARTESIAN_POINT ( 'NONE',  ( 124.3962635252314470, 4.472830434245840259, -4.472830434245838482 ) ) ;
#8652=CARTESIAN_POINT ( 'NONE',  ( 89.16209685856478018, -5.291415217122919401, 3.054999999999998384 ) ) ;
#8672=CARTESIAN_POINT ( 'NONE',  ( 0.000000000000000000, 0.000000000000000000, 7.950000000000000178 ) ) ;
#8686=DIRECTION ( 'NONE',  ( 0.000000000000000000, 0.000000000000000000, 1.000000000000000000 ) ) ;
#8695=CARTESIAN_POINT ( 'NONE',  ( 106.7291666666666430, 7.950000000000001954, -2.130196079827421762 ) ) ;
#8710=CARTESIAN_POINT ( 'NONE',  ( 106.0212635252314470, -4.472830434245839371, -4.472830434245840259 ) ) ;
#8720=CARTESIAN_POINT ( 'NONE',  ( 33.03752705046289151, -9.735942053221456900E-16, 7.949999999999998401 ) ) ;
#8724=CARTESIAN_POINT ( 'NONE',  ( 27.10416666666666785, 2.130196079827422206, 7.950000000000001954 ) ) ;
#8734=CARTESIAN_POINT ( 'NONE',  ( 120.9537635252314658, -6.109999999999998543, -3.741295971395162543E-16 ) ) ;
#8744=CARTESIAN_POINT ( 'NONE',  ( 44.77126352523143282, 4.472830434245839371, 4.472830434245842035 ) ) ;
#8751=CARTESIAN_POINT ( 'NONE',  ( 40.59959685856476597, -6.109999999999997655, -1.637169565754160283 ) ) ;
#8780=CARTESIAN_POINT ( 'NONE',  ( 56.49543019189812298, 5.291415217122916737, 3.055000000000001936 ) ) ;
#8816=CARTESIAN_POINT ( 'NONE',  ( 122.5579301918981088, 6.110000000000001208, -1.637169565754156286 ) ) ;
#8820=AXIS2_PLACEMENT_3D ( 'NONE', #31378, #20471, #98750 ) ;
#8823=CARTESIAN_POINT ( 'NONE',  ( 75.18336038379622721, -2.130196079827426203, 7.949999999999996625 ) ) ;
#8829=ORIENTED_EDGE ( 'NONE', *, *, #61521, .F. ) ;
#8832=DIRECTION ( 'NONE',  ( -1.000000000000000000, -0.000000000000000000, -0.000000000000000000 ) ) ;
#8851=CARTESIAN_POINT ( 'NONE',  ( 37.09959685856476597, -6.109999999999998543, -1.637169565754160727 ) ) ;
#8870=CARTESIAN_POINT ( 'NONE',  ( 79.74999999999998579, -9.735942053221458872E-16, 7.950000000000000178 ) ) ;
#8876=CARTESIAN_POINT ( 'NONE',  ( 56.22502705046289151, 5.819803920172573086, -5.819803920172572198 ) ) ;
#8881=CARTESIAN_POINT ( 'NONE',  ( 53.49999999999999289, 0.000000000000000000, -7.950000000000000178 ) ) ;
#8890=CARTESIAN_POINT ( 'NONE',  ( 47.25043019189810423, 3.055000000000002824, -5.291415217122919401 ) ) ;
#8908=CARTESIAN_POINT ( 'NONE',  ( 79.62543019189810423, 5.291415217122919401, 3.055000000000002824 ) ) ;
#8916=CARTESIAN_POINT ( 'NONE',  ( 64.66209685856478018, -5.291415217122919401, 3.054999999999997939 ) ) ;
#8925=CARTESIAN_POINT ( 'NONE',  ( 0.000000000000000000, 0.000000000000000000, 0.000000000000000000 ) ) ;
#8943=CARTESIAN_POINT ( 'NONE',  ( 40.18336038379621300, -2.130196079827426203, 7.949999999999996625 ) ) ;
#8953=CARTESIAN_POINT ( 'NONE',  ( 85.22459685856479439, -1.637169565754160949, 6.109999999999997655 ) ) ;
#8970=ORIENTED_EDGE ( 'NONE', *, *, #8080, .F. ) ;
#8979=CARTESIAN_POINT ( 'NONE',  ( 35.14626352523143993, -4.472830434245840259, 4.472830434245838482 ) ) ;
#8997=CARTESIAN_POINT ( 'NONE',  ( 109.4541937171295558, 6.884901960086283523, 3.975000000000002753 ) ) ;
#9021=( BOUNDED_CURVE ( )  B_SPLINE_CURVE ( 2, ( #64394, #28917, #86156, #73156, #117321, #40519, #106425, #130382, #9248, #51393, #95587, #97734, #139847 ),
 .UNSPECIFIED., .F., .T. ) 
 B_SPLINE_CURVE_WITH_KNOTS ( ( 3, 2, 2, 2, 2, 2, 3 ),
 ( 0.3499999999999999778, 0.3527777777777778012, 0.3555555555555555691, 0.3583333333333333370, 0.3611111111111111049, 0.3638888888888888729, 0.3666666666666666408 ),
 .UNSPECIFIED. ) 
 CURVE ( )  GEOMETRIC_REPRESENTATION_ITEM ( )  RATIONAL_B_SPLINE_CURVE ( ( 1.000000000000000000, 0.9659258262890683122, 1.000000000000000000, 0.9659258262890683122, 1.000000000000000000, 0.9659258262890683122, 1.000000000000000000, 0.9659258262890683122, 1.000000000000000000, 0.9659258262890683122, 1.000000000000000000, 0.9659258262890683122, 1.000000000000000000 ) ) 
 REPRESENTATION_ITEM ( '' )  );
#9023=ORIENTED_EDGE ( 'NONE', *, *, #555, .F. ) ;
#9031=CARTESIAN_POINT ( 'NONE',  ( 64.66209685856478018, -5.291415217122919401, 3.054999999999998384 ) ) ;
#9063=CARTESIAN_POINT ( 'NONE',  ( 79.99586038379621300, -3.974999999999998312, -6.884901960086286188 ) ) ;
#9079=CARTESIAN_POINT ( 'NONE',  ( 77.00043019189811844, -3.055000000000002380, 5.291415217122920289 ) ) ;
#9096=CARTESIAN_POINT ( 'NONE',  ( 62.85459685856477563, -1.637169565754161615, 6.110000000000000320 ) ) ;
#9126=CARTESIAN_POINT ( 'NONE',  ( 111.9120968585647944, 5.291415217122921177, -3.054999999999994831 ) ) ;
#9156=CARTESIAN_POINT ( 'NONE',  ( 60.22959685856476142, -6.110000000000000320, -1.637169565754161393 ) ) ;
#9163=CARTESIAN_POINT ( 'NONE',  ( 98.43793019189811844, -6.110000000000001208, 1.637169565754158951 ) ) ;
#9180=CARTESIAN_POINT ( 'NONE',  ( 120.3704301918981230, -3.055000000000001492, 5.291415217122917625 ) ) ;
#9197=FACE_OUTER_BOUND ( 'NONE', #1382, .T. ) ;
#9204=CARTESIAN_POINT ( 'NONE',  ( 26.39626352523143282, 4.472830434245840259, -4.472830434245839371 ) ) ;
#9226=CARTESIAN_POINT ( 'NONE',  ( 108.7250270504628844, 5.819803920172573086, -5.819803920172572198 ) ) ;
#9248=CARTESIAN_POINT ( 'NONE',  ( 91.37086038379622721, 6.884901960086289741, -3.974999999999993427 ) ) ;
#9257=CARTESIAN_POINT ( 'NONE',  ( 93.75000000000000000, -9.735942053221458872E-16, 7.950000000000000178 ) ) ;
#9272=CARTESIAN_POINT ( 'NONE',  ( 95.08376352523144703, -6.110000000000001208, -3.741295971395164515E-16 ) ) ;
#9281=CARTESIAN_POINT ( 'NONE',  ( 93.53709685856479439, -3.054999999999998828, -5.291415217122919401 ) ) ;
#9304=( BOUNDED_CURVE ( )  B_SPLINE_CURVE ( 2, ( #25773, #78749, #46887, #112786, #134570, #57723, #122962 ),
 .UNSPECIFIED., .F., .F. ) 
 B_SPLINE_CURVE_WITH_KNOTS ( ( 3, 2, 2, 3 ),
 ( 0.9666666666666666741, 0.9694444444444444420, 0.9722222222222222099, 0.9741589280471857348 ),
 .UNSPECIFIED. ) 
 CURVE ( )  GEOMETRIC_REPRESENTATION_ITEM ( )  RATIONAL_B_SPLINE_CURVE ( ( 1.000000000000000000, 0.9659258262890683122, 1.000000000000000000, 0.9659258262890683122, 1.000000000000000000, 0.9762430057455590005, 0.9856134340835827068 ) ) 
 REPRESENTATION_ITEM ( '' )  );
#9316=AXIS2_PLACEMENT_3D ( 'NONE', #1619, #55343, #56082 ) ;
#9334=CARTESIAN_POINT ( 'NONE',  ( 27.03709685856478373, -3.054999999999998828, -5.291415217122919401 ) ) ;
#9337=CARTESIAN_POINT ( 'NONE',  ( 126.8754301918981184, -5.291415217122920289, -3.055000000000001492 ) ) ;
#9353=ORIENTED_EDGE ( 'NONE', *, *, #122732, .F. ) ;
#9374=CARTESIAN_POINT ( 'NONE',  ( 91.34959685856478018, 6.109999999999997655, 1.637169565754163836 ) ) ;
#9375=CARTESIAN_POINT ( 'NONE',  ( 5.980202007725322844, -9.485991381305455050, 0.5885017396600767947 ) ) ;
#9426=CARTESIAN_POINT ( 'NONE',  ( 103.2291666666666714, 7.950000000000001954, -2.130196079827421762 ) ) ;
#9451=CARTESIAN_POINT ( 'NONE',  ( 30.99586038379621655, -3.974999999999998312, -6.884901960086286188 ) ) ;
#9456=CARTESIAN_POINT ( 'NONE',  ( 30.75000000000000000, -9.735942053221458872E-16, 7.950000000000000178 ) ) ;
#9457=EDGE_LOOP ( 'NONE', ( #130653, #98634, #123307, #56251 ) ) ;
#9469=CARTESIAN_POINT ( 'NONE',  ( 121.8287635252314516, 0.000000000000000000, -6.109999999999998543 ) ) ;
#9480=CARTESIAN_POINT ( 'NONE',  ( 45.35459685856476852, -1.637169565754161615, 6.110000000000000320 ) ) ;
#9489=CARTESIAN_POINT ( 'NONE',  ( 43.66209685856478728, -5.291415217122919401, 3.054999999999997939 ) ) ;
#9519=CARTESIAN_POINT ( 'NONE',  ( 59.84959685856476597, 6.109999999999996767, 1.637169565754163836 ) ) ;
#9559=CARTESIAN_POINT ( 'NONE',  ( 120.2245968585648086, -1.637169565754161171, 6.109999999999998543 ) ) ;
#9572=EDGE_LOOP ( 'NONE', ( #99934, #105720, #135150, #75962 ) ) ;
#9583=VERTEX_POINT ( 'NONE', #124963 ) ;
#9601=CARTESIAN_POINT ( 'NONE',  ( 40.59959685856476597, -6.109999999999998543, -1.637169565754160727 ) ) ;
#9625=CARTESIAN_POINT ( 'NONE',  ( 79.16666666666665719, 6.884901960086285300, 3.975000000000003642 ) ) ;
#9631=CARTESIAN_POINT ( 'NONE',  ( 57.53752705046289151, -9.735942053221456900E-16, 7.949999999999998401 ) ) ;
#9636=CARTESIAN_POINT ( 'NONE',  ( 58.45833333333333570, 3.974999999999997424, 6.884901960086288852 ) ) ;
#9649=CARTESIAN_POINT ( 'NONE',  ( 48.85459685856476142, -1.637169565754161615, 6.110000000000000320 ) ) ;
#9668=CARTESIAN_POINT ( 'NONE',  ( 81.81293019189810423, -1.637169565754159617, -6.110000000000001208 ) ) ;
#9677=ORIENTED_EDGE ( 'NONE', *, *, #105221, .F. ) ;
#9679=CARTESIAN_POINT ( 'NONE',  ( 63.64126352523144448, 4.472830434245836706, 4.472830434245840259 ) ) ;
#9709=CARTESIAN_POINT ( 'NONE',  ( 80.55793019189810877, 6.110000000000000320, -1.637169565754156064 ) ) ;
#9734=CARTESIAN_POINT ( 'NONE',  ( 36.75043019189811133, 3.055000000000002824, -5.291415217122919401 ) ) ;
#9739=CARTESIAN_POINT ( 'NONE',  ( 89.47502705046288440, -5.819803920172573086, 5.819803920172573086 ) ) ;
#9761=CARTESIAN_POINT ( 'NONE',  ( 108.2875270504628986, 0.000000000000000000, -7.949999999999998401 ) ) ;
#9776=CARTESIAN_POINT ( 'NONE',  ( 96.91252705046289861, -7.949999999999998401, -4.867971026610728450E-16 ) ) ;
#9791=CARTESIAN_POINT ( 'NONE',  ( 66.70376352523143737, 6.109999999999999432, 1.122388791418549108E-15 ) ) ;
#9821=CARTESIAN_POINT ( 'NONE',  ( 87.72502705046291283, 5.819803920172573086, -5.819803920172572198 ) ) ;
#9825=CARTESIAN_POINT ( 'NONE',  ( 81.93749999999998579, 5.819803920172573974, -5.819803920172572198 ) ) ;
#9836=CARTESIAN_POINT ( 'NONE',  ( 76.12543019189810423, 5.291415217122919401, 3.055000000000002824 ) ) ;
#9852=ORIENTED_EDGE ( 'NONE', *, *, #136460, .F. ) ;
#9855=CARTESIAN_POINT ( 'NONE',  ( 67.37543019189810423, -5.291415217122920289, -3.055000000000001492 ) ) ;
#9879=CARTESIAN_POINT ( 'NONE',  ( 61.52083333333332149, 7.949999999999998401, 2.130196079827431532 ) ) ;
#9885=CARTESIAN_POINT ( 'NONE',  ( 116.8704301918981230, -3.055000000000001492, 5.291415217122917625 ) ) ;
#9911=CARTESIAN_POINT ( 'NONE',  ( 66.79209685856477563, -5.291415217122921177, 3.054999999999999272 ) ) ;
#9917=CARTESIAN_POINT ( 'NONE',  ( 103.1045968585647614, 1.637169565754164946, -6.109999999999999432 ) ) ;
#9918=( BOUNDED_CURVE ( )  B_SPLINE_CURVE ( 2, ( #122836, #100379, #112667, #14782, #35867, #13331, #68486 ),
 .UNSPECIFIED., .F., .T. ) 
 B_SPLINE_CURVE_WITH_KNOTS ( ( 3, 2, 2, 3 ),
 ( 0.000000000000000000, 0.002777777777777780052, 0.005555555555555560104, 0.008333333333333340157 ),
 .UNSPECIFIED. ) 
 CURVE ( )  GEOMETRIC_REPRESENTATION_ITEM ( )  RATIONAL_B_SPLINE_CURVE ( ( 1.000000000000000000, 0.9659258262890683122, 1.000000000000000000, 0.9659258262890683122, 1.000000000000000000, 0.9659258262890678681, 1.000000000000000444 ) ) 
 REPRESENTATION_ITEM ( '' )  );
#9934=CARTESIAN_POINT ( 'NONE',  ( 121.0995968585647802, -6.109999999999997655, -1.637169565754160283 ) ) ;
#9948=CARTESIAN_POINT ( 'NONE',  ( 11.74750898584326464, -8.547897970587566618, -4.147060425997655564 ) ) ;
#9962=CARTESIAN_POINT ( 'NONE',  ( 31.20876352523144348, -7.482591942790329030E-16, 6.110000000000001208 ) ) ;
#9987=( BOUNDED_CURVE ( )  B_SPLINE_CURVE ( 2, ( #83232, #27393, #115814, #36170, #36856, #39012, #60066, #28138, #92657, #91952, #80398, #16520, #26705 ),
 .UNSPECIFIED., .F., .T. ) 
 B_SPLINE_CURVE_WITH_KNOTS ( ( 3, 2, 2, 2, 2, 2, 3 ),
 ( 0.1166666666666666408, 0.1194444444444444225, 0.1222222222222221905, 0.1249999999999999722, 0.1277777777777777402, 0.1305555555555555358, 0.1333333333333333037 ),
 .UNSPECIFIED. ) 
 CURVE ( )  GEOMETRIC_REPRESENTATION_ITEM ( )  RATIONAL_B_SPLINE_CURVE ( ( 1.000000000000000444, 0.9659258262890679791, 1.000000000000000000, 0.9659258262890683122, 1.000000000000000000, 0.9659258262890683122, 1.000000000000000000, 0.9659258262890683122, 1.000000000000000000, 0.9659258262890683122, 1.000000000000000000, 0.9659258262890686453, 0.9999999999999996669 ) ) 
 REPRESENTATION_ITEM ( '' )  );
#9988=CARTESIAN_POINT ( 'NONE',  ( 115.2875270504628986, 0.000000000000000000, -7.949999999999998401 ) ) ;
#9989=CARTESIAN_POINT ( 'NONE',  ( 50.10002705046289151, 5.819803920172570422, 5.819803920172575751 ) ) ;
#10004=VERTEX_POINT ( 'NONE', #117374 ) ;
#10029=CARTESIAN_POINT ( 'NONE',  ( 94.64626352523143282, -4.472830434245840259, 4.472830434245839371 ) ) ;
#10039=CARTESIAN_POINT ( 'NONE',  ( 88.14126352523143737, 4.472830434245836706, 4.472830434245840259 ) ) ;
#10044=ORIENTED_EDGE ( 'NONE', *, *, #135848, .F. ) ;
#10052=DIRECTION ( 'NONE',  ( -1.000000000000000000, -0.000000000000000000, -0.000000000000000000 ) ) ;
#10064=CARTESIAN_POINT ( 'NONE',  ( 26.79783616915502975, -7.489999999999998437, -4.586302262806838083E-16 ) ) ;
#10090=CARTESIAN_POINT ( 'NONE',  ( 124.2504301918981184, 3.055000000000002824, -5.291415217122919401 ) ) ;
#10124=CARTESIAN_POINT ( 'NONE',  ( 93.53709685856479439, -3.054999999999999272, -5.291415217122919401 ) ) ;
#10125=CARTESIAN_POINT ( 'NONE',  ( 6.540342856384453896, -9.242792321178736614, -2.199412111314436036 ) ) ;
#10128=VERTEX_POINT ( 'NONE', #61202 ) ;
#10129=CYLINDRICAL_SURFACE ( 'NONE', #56749, 7.950000000000000178 ) ;
#10170=CARTESIAN_POINT ( 'NONE',  ( 97.54166666666667140, -3.975000000000002753, 6.884901960086286188 ) ) ;
#10190=CARTESIAN_POINT ( 'NONE',  ( 27.93336038379622011, 2.130196079827431532, -7.949999999999997513 ) ) ;
#10195=CARTESIAN_POINT ( 'NONE',  ( 117.1045968585647898, 1.637169565754164946, -6.109999999999999432 ) ) ;
#10203=CARTESIAN_POINT ( 'NONE',  ( 123.5787635252314516, -7.482591942790325086E-16, 6.109999999999998543 ) ) ;
#10214=CARTESIAN_POINT ( 'NONE',  ( 37.04209685856476852, 5.291415217122923842, -3.054999999999996163 ) ) ;
#10223=CARTESIAN_POINT ( 'NONE',  ( 36.51626352523145158, -4.472830434245839371, 4.472830434245839371 ) ) ;
#10239=ORIENTED_EDGE ( 'NONE', *, *, #102832, .T. ) ;
#10250=CARTESIAN_POINT ( 'NONE',  ( 51.68293019189810877, -1.637169565754158951, -6.109999999999998543 ) ) ;
#10263=CYLINDRICAL_SURFACE ( 'NONE', #122369, 6.349999999999997868 ) ;
#10287=CARTESIAN_POINT ( 'NONE',  ( 122.9954301918981230, 5.291415217122917625, 3.055000000000002380 ) ) ;
#10299=ORIENTED_EDGE ( 'NONE', *, *, #22679, .F. ) ;
#10307=EDGE_LOOP ( 'NONE', ( #56637, #18371 ) ) ;
#10327=CARTESIAN_POINT ( 'NONE',  ( 36.80793019189810167, -6.109999999999999432, 1.637169565754158507 ) ) ;
#10343=CARTESIAN_POINT ( 'NONE',  ( 117.9795968585647898, 6.109999999999999432, 1.637169565754164280 ) ) ;
#10353=CARTESIAN_POINT ( 'NONE',  ( 53.45419371712956291, 6.884901960086283523, 3.975000000000002753 ) ) ;
#10354=DIRECTION ( 'NONE',  ( -1.000000000000000000, -0.000000000000000000, -0.000000000000000000 ) ) ;
#10358=CARTESIAN_POINT ( 'NONE',  ( 41.97916666666665719, -7.950000000000001066, 2.130196079827424427 ) ) ;
#10365=CARTESIAN_POINT ( 'NONE',  ( 43.45876352523143993, 0.000000000000000000, -6.110000000000001208 ) ) ;
#10375=EDGE_LOOP ( 'NONE', ( #24516, #40006, #62879, #59263 ) ) ;
#10376=EDGE_CURVE ( 'NONE', #72906, #90062, #1553, .T. ) ;
#10381=CARTESIAN_POINT ( 'NONE',  ( 81.95876352523143282, 0.000000000000000000, -6.110000000000001208 ) ) ;
#10390=CARTESIAN_POINT ( 'NONE',  ( 67.87043019189812298, -3.055000000000001492, 5.291415217122917625 ) ) ;
#10409=CARTESIAN_POINT ( 'NONE',  ( 41.35002705046289151, -5.819803920172573086, -5.819803920172573086 ) ) ;
#10420=CARTESIAN_POINT ( 'NONE',  ( 70.78709685856478018, 3.054999999999997495, 5.291415217122919401 ) ) ;
#10445=CARTESIAN_POINT ( 'NONE',  ( 35.72959685856474721, -6.110000000000000320, -1.637169565754161393 ) ) ;
#10473=DIRECTION ( 'NONE',  ( 0.000000000000000000, 0.000000000000000000, -1.000000000000000000 ) ) ;
#10485=ORIENTED_EDGE ( 'NONE', *, *, #132062, .F. ) ;
#10495=CARTESIAN_POINT ( 'NONE',  ( 51.74999999999999289, -9.735942053221458872E-16, 7.950000000000000178 ) ) ;
#10498=CARTESIAN_POINT ( 'NONE',  ( 66.99543019189812298, 5.291415217122917625, 3.055000000000002380 ) ) ;
#10502=CARTESIAN_POINT ( 'NONE',  ( 84.12500000000000000, -7.950000000000000178, -4.867971026610729436E-16 ) ) ;
#10520=CARTESIAN_POINT ( 'NONE',  ( 88.16252705046289861, 7.949999999999998401, 1.460391307983218338E-15 ) ) ;
#10524=CARTESIAN_POINT ( 'NONE',  ( 86.02083333333330017, 7.949999999999999289, 2.130196079827431532 ) ) ;
#10534=CARTESIAN_POINT ( 'NONE',  ( 74.52126352523141861, -4.472830434245839371, -4.472830434245840259 ) ) ;
#10544=ORIENTED_EDGE ( 'NONE', *, *, #3551, .T. ) ;
#10553=CARTESIAN_POINT ( 'NONE',  ( 61.83376352523143993, 6.110000000000001208, 1.122388791418549305E-15 ) ) ;
#10581=CARTESIAN_POINT ( 'NONE',  ( 114.0995968585647518, -6.109999999999997655, -1.637169565754160283 ) ) ;
#10595=CARTESIAN_POINT ( 'NONE',  ( 36.72916666666665719, 7.950000000000001954, -2.130196079827421762 ) ) ;
#10605=ORIENTED_EDGE ( 'NONE', *, *, #39758, .T. ) ;
#10608=EDGE_CURVE ( 'NONE', #108642, #13817, #119603, .T. ) ;
#10610=CARTESIAN_POINT ( 'NONE',  ( 65.77126352523143282, 4.472830434245838482, 4.472830434245842035 ) ) ;
#10616=CARTESIAN_POINT ( 'NONE',  ( 103.8337635252314328, 6.110000000000001208, 1.122388791418549305E-15 ) ) ;
#10633=CARTESIAN_POINT ( 'NONE',  ( 125.4745968585647944, 1.637169565754164280, -6.109999999999996767 ) ) ;
#10634=ORIENTED_EDGE ( 'NONE', *, *, #4816, .F. ) ;
#10655=CARTESIAN_POINT ( 'NONE',  ( 31.93793019189809712, -6.110000000000001208, 1.637169565754158951 ) ) ;
#10674=CARTESIAN_POINT ( 'NONE',  ( 109.8916937171295416, 2.130196079827421762, 7.950000000000001066 ) ) ;
#10675=CARTESIAN_POINT ( 'NONE',  ( 50.39169371712954870, 2.130196079827421762, 7.950000000000000178 ) ) ;
#10719=CARTESIAN_POINT ( 'NONE',  ( 90.41709685856477563, 3.054999999999998828, 5.291415217122922066 ) ) ;
#10727=CARTESIAN_POINT ( 'NONE',  ( 48.97916666666665009, -7.950000000000000178, 2.130196079827424427 ) ) ;
#10729=CARTESIAN_POINT ( 'NONE',  ( 83.76626352523145158, 4.472830434245839371, -4.472830434245838482 ) ) ;
#10732=CARTESIAN_POINT ( 'NONE',  ( 116.0625000000000000, -5.819803920172573086, -5.819803920172573974 ) ) ;
#10762=CARTESIAN_POINT ( 'NONE',  ( 119.8541666666666572, -2.130196079827463507, -7.949999999999979750 ) ) ;
#10770=CARTESIAN_POINT ( 'NONE',  ( 116.4541937171295558, 6.884901960086283523, 3.975000000000002753 ) ) ;
#10798=FACE_OUTER_BOUND ( 'NONE', #24250, .T. ) ;
#10815=CARTESIAN_POINT ( 'NONE',  ( 86.53709685856478018, -3.054999999999999272, -5.291415217122919401 ) ) ;
#10816=CARTESIAN_POINT ( 'NONE',  ( 6.176602844086411359, -9.397266779063615516, -1.419141200614698395 ) ) ;
#10848=CARTESIAN_POINT ( 'NONE',  ( 31.47916666666665364, -7.950000000000000178, 2.130196079827424427 ) ) ;
#10859=CARTESIAN_POINT ( 'NONE',  ( 101.9166666666666714, -6.884901960086287076, -3.975000000000000977 ) ) ;
#10885=CARTESIAN_POINT ( 'NONE',  ( 118.2712635252314470, 4.472830434245839371, 4.472830434245842035 ) ) ;
#10897=CARTESIAN_POINT ( 'NONE',  ( 115.8495968585647802, 6.109999999999996767, 1.637169565754163836 ) ) ;
#10906=VECTOR ( 'NONE', #122739, 1000.000000000000000 ) ;
#10907=CARTESIAN_POINT ( 'NONE',  ( 40.83376352523143993, 6.110000000000001208, 1.122388791418549305E-15 ) ) ;
#10908=VERTEX_POINT ( 'NONE', #15813 ) ;
#10916=CARTESIAN_POINT ( 'NONE',  ( 30.09959685856478018, -6.109999999999997655, -1.637169565754160283 ) ) ;
#10943=CARTESIAN_POINT ( 'NONE',  ( 43.95376352523145158, -6.109999999999998543, -3.741295971395162543E-16 ) ) ;
#10964=EDGE_LOOP ( 'NONE', ( #31577, #91235, #21833, #49192 ) ) ;
#10978=CARTESIAN_POINT ( 'NONE',  ( 123.2870968585647944, 3.054999999999997939, 5.291415217122920289 ) ) ;
#11020=CARTESIAN_POINT ( 'NONE',  ( 27.62043019189810877, 3.055000000000002380, -5.291415217122917625 ) ) ;
#11024=CARTESIAN_POINT ( 'NONE',  ( 125.3958333333333428, -2.130196079827427091, 7.949999999999999289 ) ) ;
#11035=CARTESIAN_POINT ( 'NONE',  ( 122.7920968585647756, -5.291415217122921177, 3.054999999999999272 ) ) ;
#11039=VECTOR ( 'NONE', #86428, 1000.000000000000000 ) ;
#11045=CARTESIAN_POINT ( 'NONE',  ( 56.95419371712956291, 6.884901960086283523, 3.975000000000002753 ) ) ;
#11051=CARTESIAN_POINT ( 'NONE',  ( 41.83333333333333570, -6.884901960086287964, 3.974999999999998312 ) ) ;
#11061=CARTESIAN_POINT ( 'NONE',  ( 40.83376352523143993, 6.110000000000001208, 1.122388791418549305E-15 ) ) ;
#11062=ORIENTED_EDGE ( 'NONE', *, *, #138528, .T. ) ;
#11076=ORIENTED_EDGE ( 'NONE', *, *, #22679, .T. ) ;
#11077=CARTESIAN_POINT ( 'NONE',  ( 79.18793019189810423, 6.110000000000002984, -1.637169565754156730 ) ) ;
#11086=CARTESIAN_POINT ( 'NONE',  ( 67.43293019189812298, 1.637169565754156508, 6.110000000000000320 ) ) ;
#11114=CARTESIAN_POINT ( 'NONE',  ( 71.95376352523145158, -6.109999999999998543, -3.741295971395162543E-16 ) ) ;
#11122=LINE ( 'NONE', #99571, #124754 ) ;
#11135=CARTESIAN_POINT ( 'NONE',  ( 26.97959685856476497, 6.109999999999999432, 1.637169565754164280 ) ) ;
#11159=CARTESIAN_POINT ( 'NONE',  ( 27.24999999999999645, -9.735942053221458872E-16, 7.950000000000000178 ) ) ;
#11185=CARTESIAN_POINT ( 'NONE',  ( 69.47459685856475176, 1.637169565754164280, -6.109999999999997655 ) ) ;
#11189=CARTESIAN_POINT ( 'NONE',  ( 32.89169371712954870, 2.130196079827421762, 7.950000000000000178 ) ) ;
#11201=CARTESIAN_POINT ( 'NONE',  ( 104.7875270504628986, 0.000000000000000000, -7.949999999999998401 ) ) ;
#11214=CARTESIAN_POINT ( 'NONE',  ( 81.74586038379622721, 3.974999999999996980, 6.884901960086287964 ) ) ;
#11219=CARTESIAN_POINT ( 'NONE',  ( 69.54166666666667140, -3.975000000000002753, 6.884901960086286188 ) ) ;
#11232=CARTESIAN_POINT ( 'NONE',  ( 77.58376352523144703, -6.110000000000001208, -3.741295971395164515E-16 ) ) ;
#11256=CARTESIAN_POINT ( 'NONE',  ( 60.08376352523143993, -6.110000000000001208, -3.741295971395164515E-16 ) ) ;
#11261=CARTESIAN_POINT ( 'NONE',  ( 124.4750270504628844, -5.819803920172573086, 5.819803920172573086 ) ) ;
#11270=CARTESIAN_POINT ( 'NONE',  ( 112.3708603837962272, 6.884901960086289741, -3.974999999999993427 ) ) ;
#11277=CARTESIAN_POINT ( 'NONE',  ( 128.8886022459138019, 0.000000000000000000, -6.349999999999997868 ) ) ;
#11278=CARTESIAN_POINT ( 'NONE',  ( 61.81249999999998579, 5.819803920172571310, 5.819803920172576639 ) ) ;
#11286=CARTESIAN_POINT ( 'NONE',  ( 106.9537635252314516, -6.109999999999998543, -3.741295971395162543E-16 ) ) ;
#11305=ORIENTED_EDGE ( 'NONE', *, *, #25557, .F. ) ;
#11308=CARTESIAN_POINT ( 'NONE',  ( 54.68793019189810423, 6.110000000000002984, -1.637169565754156730 ) ) ;
#11313=CARTESIAN_POINT ( 'NONE',  ( 91.14626352523144703, -4.472830434245840259, 4.472830434245838482 ) ) ;
#11329=CARTESIAN_POINT ( 'NONE',  ( 124.5995968585647802, -6.109999999999997655, -1.637169565754160283 ) ) ;
#11333=AXIS2_PLACEMENT_3D ( 'NONE', #49048, #114953, #81690 ) ;
#11348=ORIENTED_EDGE ( 'NONE', *, *, #130896, .F. ) ;
#11377=CARTESIAN_POINT ( 'NONE',  ( 114.1208603837962414, -6.884901960086286188, 3.974999999999997424 ) ) ;
#11395=CARTESIAN_POINT ( 'NONE',  ( 106.6045968585647472, 1.637169565754164946, -6.109999999999999432 ) ) ;
#11422=CARTESIAN_POINT ( 'NONE',  ( 94.20876352523144703, -7.482591942790329030E-16, 6.110000000000001208 ) ) ;
#11438=CARTESIAN_POINT ( 'NONE',  ( 86.82876352523145158, 0.000000000000000000, -6.109999999999998543 ) ) ;
#11471=CARTESIAN_POINT ( 'NONE',  ( 67.50000000000000000, 0.000000000000000000, -7.950000000000000178 ) ) ;
#11477=ORIENTED_EDGE ( 'NONE', *, *, #57378, .T. ) ;
#11521=CARTESIAN_POINT ( 'NONE',  ( 79.97459685856479439, 1.637169565754164280, -6.109999999999997655 ) ) ;
#11573=CARTESIAN_POINT ( 'NONE',  ( 103.9583333333333286, 3.974999999999997424, 6.884901960086288852 ) ) ;
#11594=CARTESIAN_POINT ( 'NONE',  ( 86.26669371712955581, -7.949999999999998401, 2.130196079827423983 ) ) ;
#11598=CARTESIAN_POINT ( 'NONE',  ( 124.8337635252314470, 6.110000000000001208, 1.122388791418549305E-15 ) ) ;
#11606=CARTESIAN_POINT ( 'NONE',  ( 118.3287635252314658, 0.000000000000000000, -6.109999999999998543 ) ) ;
#11618=CARTESIAN_POINT ( 'NONE',  ( 37.62543019189811133, 5.291415217122919401, 3.055000000000002824 ) ) ;
#11624=( BOUNDED_CURVE ( )  B_SPLINE_CURVE ( 2, ( #65493, #128572, #75630, #8184, #73490, #117654, #63357, #41547, #51020, #18340, #40852, #97334, #130001 ),
 .UNSPECIFIED., .F., .F. ) 
 B_SPLINE_CURVE_WITH_KNOTS ( ( 3, 2, 2, 2, 2, 2, 3 ),
 ( 0.4166666666666667962, 0.4194444444444445641, 0.4222222222222223320, 0.4250000000000000999, 0.4277777777777778678, 0.4305555555555556912, 0.4333333333333334592 ),
 .UNSPECIFIED. ) 
 CURVE ( )  GEOMETRIC_REPRESENTATION_ITEM ( )  RATIONAL_B_SPLINE_CURVE ( ( 0.9999999999999986677, 0.9659258262890696445, 1.000000000000000000, 0.9659258262890683122, 1.000000000000000000, 0.9659258262890683122, 1.000000000000000000, 0.9659258262890683122, 1.000000000000000000, 0.9659258262890683122, 1.000000000000000000, 0.9659258262890669799, 1.000000000000001332 ) ) 
 REPRESENTATION_ITEM ( '' )  );
#11626=CARTESIAN_POINT ( 'NONE',  ( 33.74543019189811588, -5.291415217122918513, -3.055000000000000160 ) ) ;
#11655=CARTESIAN_POINT ( 'NONE',  ( 43.80793019189810877, -6.109999999999998543, 1.637169565754158507 ) ) ;
#11662=LINE ( 'NONE', #800, #100076 ) ;
#11694=CARTESIAN_POINT ( 'NONE',  ( 106.9537635252314516, -6.109999999999999432, -3.741295971395163529E-16 ) ) ;
#11706=ORIENTED_EDGE ( 'NONE', *, *, #135782, .T. ) ;
#11724=ORIENTED_EDGE ( 'NONE', *, *, #23886, .T. ) ;
#11730=ORIENTED_EDGE ( 'NONE', *, *, #118281, .T. ) ;
#11741=CARTESIAN_POINT ( 'NONE',  ( 129.2875270504628986, 0.000000000000000000, -7.949999999999998401 ) ) ;
#11744=ORIENTED_EDGE ( 'NONE', *, *, #54990, .F. ) ;
#11762=CARTESIAN_POINT ( 'NONE',  ( 126.1462635252314328, -4.472830434245840259, 4.472830434245839371 ) ) ;
#11772=CARTESIAN_POINT ( 'NONE',  ( 47.32919371712955581, -3.975000000000001865, 6.884901960086284411 ) ) ;
#11778=CARTESIAN_POINT ( 'NONE',  ( 46.50000000000000000, 0.000000000000000000, -7.950000000000000178 ) ) ;
#11787=CARTESIAN_POINT ( 'NONE',  ( 37.47959685856476852, 6.109999999999999432, 1.637169565754164280 ) ) ;
#11801=CARTESIAN_POINT ( 'NONE',  ( 86.18793019189810423, 6.110000000000002984, -1.637169565754156730 ) ) ;
#11809=CARTESIAN_POINT ( 'NONE',  ( 60.72459685856477307, -1.637169565754160949, 6.109999999999997655 ) ) ;
#11841=CARTESIAN_POINT ( 'NONE',  ( 73.99543019189810877, 5.291415217122916737, 3.055000000000001936 ) ) ;
#11868=CARTESIAN_POINT ( 'NONE',  ( 27.41709685856476142, 3.054999999999998828, 5.291415217122922066 ) ) ;
#11901=( BOUNDED_CURVE ( )  B_SPLINE_CURVE ( 2, ( #67805, #54068, #143175, #11931, #64918, #56217, #10502, #53302, #98257, #329, #109834, #132338, #66352 ),
 .UNSPECIFIED., .F., .F. ) 
 B_SPLINE_CURVE_WITH_KNOTS ( ( 3, 2, 2, 2, 2, 2, 3 ),
 ( 0.4000000000000000777, 0.4027777777777778456, 0.4055555555555556135, 0.4083333333333334370, 0.4111111111111112049, 0.4138888888888889728, 0.4166666666666667962 ),
 .UNSPECIFIED. ) 
 CURVE ( )  GEOMETRIC_REPRESENTATION_ITEM ( )  RATIONAL_B_SPLINE_CURVE ( ( 0.9999999999999993339, 0.9659258262890689783, 1.000000000000000000, 0.9659258262890683122, 1.000000000000000000, 0.9659258262890683122, 1.000000000000000000, 0.9659258262890683122, 1.000000000000000000, 0.9659258262890683122, 1.000000000000000000, 0.9659258262890669799, 1.000000000000001332 ) ) 
 REPRESENTATION_ITEM ( '' )  );
#11925=CARTESIAN_POINT ( 'NONE',  ( 55.32876352523144448, 0.000000000000000000, -6.109999999999999432 ) ) ;
#11931=CARTESIAN_POINT ( 'NONE',  ( 84.56250000000000000, -5.819803920172573086, -5.819803920172573974 ) ) ;
#11954=CARTESIAN_POINT ( 'NONE',  ( 72.12086038379622721, -6.884901960086286188, 3.974999999999997424 ) ) ;
#11958=CARTESIAN_POINT ( 'NONE',  ( 75.81250000000000000, 5.819803920172571310, 5.819803920172575751 ) ) ;
#11971=CARTESIAN_POINT ( 'NONE',  ( 66.35459685856476142, -1.637169565754161615, 6.110000000000000320 ) ) ;
#11988=CARTESIAN_POINT ( 'NONE',  ( 68.25043019189810423, 3.055000000000002824, -5.291415217122919401 ) ) ;
#12019=CARTESIAN_POINT ( 'NONE',  ( 101.7037635252314374, 6.109999999999998543, 1.122388791418548911E-15 ) ) ;
#12041=( GEOMETRIC_REPRESENTATION_CONTEXT ( 3 ) GLOBAL_UNCERTAINTY_ASSIGNED_CONTEXT ( ( #57787 ) ) GLOBAL_UNIT_ASSIGNED_CONTEXT ( ( #133637, #66245, #48573 ) ) REPRESENTATION_CONTEXT ( 'NONE', 'WORKASPACE' ) );
#12049=CARTESIAN_POINT ( 'NONE',  ( 54.97959685856476852, 6.109999999999999432, 1.637169565754164280 ) ) ;
#12054=CARTESIAN_POINT ( 'NONE',  ( 87.20876352523143282, -7.482591942790329030E-16, 6.110000000000001208 ) ) ;
#12079=ORIENTED_EDGE ( 'NONE', *, *, #108955, .F. ) ;
#12122=CARTESIAN_POINT ( 'NONE',  ( 112.9541937171295558, 6.884901960086283523, 3.975000000000002753 ) ) ;
#12142=CARTESIAN_POINT ( 'NONE',  ( 89.68793019189810423, 6.110000000000002984, -1.637169565754156730 ) ) ;
#12159=CARTESIAN_POINT ( 'NONE',  ( 102.6000270504628844, 5.819803920172570422, 5.819803920172575751 ) ) ;
#12166=CARTESIAN_POINT ( 'NONE',  ( 88.22959685856474721, -6.110000000000000320, -1.637169565754161393 ) ) ;
#12178=CARTESIAN_POINT ( 'NONE',  ( 86.24543019189812298, -5.291415217122918513, -3.055000000000000160 ) ) ;
#12225=CARTESIAN_POINT ( 'NONE',  ( 119.4379301918980900, -6.110000000000001208, 1.637169565754158951 ) ) ;
#12226=DIRECTION ( 'NONE',  ( -1.000000000000000000, -0.000000000000000000, -0.000000000000000000 ) ) ;
#12262=CARTESIAN_POINT ( 'NONE',  ( 83.62043019189812298, 3.055000000000002380, -5.291415217122917625 ) ) ;
#12308=CARTESIAN_POINT ( 'NONE',  ( 110.0833333333333428, 6.884901960086290629, -3.974999999999994316 ) ) ;
#12313=CARTESIAN_POINT ( 'NONE',  ( 99.72916666666665719, 7.950000000000001954, -2.130196079827421762 ) ) ;
#12318=DIRECTION ( 'NONE',  ( -1.000000000000000000, -0.000000000000000000, -0.000000000000000000 ) ) ;
#12320=CARTESIAN_POINT ( 'NONE',  ( 12.27820156798389561, 8.651982939446476450, -3.925326872160782798 ) ) ;
#12322=DIRECTION ( 'NONE',  ( -1.000000000000000000, -0.000000000000000000, -0.000000000000000000 ) ) ;
#12338=CARTESIAN_POINT ( 'NONE',  ( 115.9379301918980900, -6.110000000000001208, 1.637169565754158951 ) ) ;
#12340=EDGE_CURVE ( 'NONE', #26730, #83228, #9021, .T. ) ;
#12347=CARTESIAN_POINT ( 'NONE',  ( 114.3912635252314232, -4.472830434245839371, -4.472830434245839371 ) ) ;
#12356=CARTESIAN_POINT ( 'NONE',  ( 38.50043019189809712, -3.055000000000002380, 5.291415217122920289 ) ) ;
#12365=CARTESIAN_POINT ( 'NONE',  ( 30.53709685856477307, -3.054999999999998828, -5.291415217122919401 ) ) ;
#12374=CARTESIAN_POINT ( 'NONE',  ( 0.000000000000000000, 9.735942053221458872E-16, -7.950000000000000178 ) ) ;
#12395=CARTESIAN_POINT ( 'NONE',  ( 42.93293019189810877, 1.637169565754156508, 6.110000000000000320 ) ) ;
#12430=CARTESIAN_POINT ( 'NONE',  ( 109.4329301918981088, 1.637169565754156730, 6.110000000000001208 ) ) ;
#12471=CARTESIAN_POINT ( 'NONE',  ( 125.5000000000000000, -3.441786896390352624, 7.166352137582667758 ) ) ;
#12472=CARTESIAN_POINT ( 'NONE',  ( 30.68293019189811943, -1.637169565754159173, -6.109999999999999432 ) ) ;
#12491=CARTESIAN_POINT ( 'NONE',  ( 119.1462635252314470, -4.472830434245840259, 4.472830434245839371 ) ) ;
#12498=( BOUNDED_CURVE ( )  B_SPLINE_CURVE ( 2, ( #37473, #5513, #81709, #71527, #15652, #26580, #126585, #36732, #94671, #17134, #70136, #38887, #70825 ),
 .UNSPECIFIED., .F., .T. ) 
 B_SPLINE_CURVE_WITH_KNOTS ( ( 3, 2, 2, 2, 2, 2, 3 ),
 ( 0.06666666666665739538, 0.06944444444443478859, 0.07222222222221218180, 0.07499999999998957501, 0.07777777777776696821, 0.08055555555554437530, 0.08333333333332175463 ),
 .UNSPECIFIED. ) 
 CURVE ( )  GEOMETRIC_REPRESENTATION_ITEM ( )  RATIONAL_B_SPLINE_CURVE ( ( 1.000000000000113687, 0.9659258262889546254, 1.000000000000000000, 0.9659258262890683122, 1.000000000000000000, 0.9659258262890683122, 1.000000000000000000, 0.9659258262890683122, 1.000000000000000000, 0.9659258262890683122, 1.000000000000000000, 0.9659258262892103097, 0.9999999999998580025 ) ) 
 REPRESENTATION_ITEM ( '' )  );
#12502=CARTESIAN_POINT ( 'NONE',  ( 50.10002705046289151, 5.819803920172570422, 5.819803920172574863 ) ) ;
#12508=CARTESIAN_POINT ( 'NONE',  ( 49.56249999999999289, -5.819803920172572198, -5.819803920172573086 ) ) ;
#12516=CARTESIAN_POINT ( 'NONE',  ( 40.25043019189809712, 3.055000000000002824, -5.291415217122919401 ) ) ;
#12540=CARTESIAN_POINT ( 'NONE',  ( 57.37043019189810877, -3.055000000000001492, 5.291415217122917625 ) ) ;
#12568=CARTESIAN_POINT ( 'NONE',  ( 78.07876352523145158, -7.482591942790325086E-16, 6.109999999999998543 ) ) ;
#12592=ORIENTED_EDGE ( 'NONE', *, *, #69124, .T. ) ;
#12594=CARTESIAN_POINT ( 'NONE',  ( 27.12543019189810067, 5.291415217122919401, 3.055000000000002824 ) ) ;
#12599=CARTESIAN_POINT ( 'NONE',  ( 89.76669371712954160, -7.949999999999998401, 2.130196079827423983 ) ) ;
#12644=CARTESIAN_POINT ( 'NONE',  ( 52.99543019189811588, 5.291415217122917625, 3.055000000000002380 ) ) ;
#12663=CARTESIAN_POINT ( 'NONE',  ( 26.51360224591381254, -6.350000000000003197, -3.888253587292850026E-16 ) ) ;
#12667=CARTESIAN_POINT ( 'NONE',  ( 70.95419371712955581, 6.884901960086283523, 3.975000000000002753 ) ) ;
#12672=CARTESIAN_POINT ( 'NONE',  ( 72.75000000000000000, -9.735942053221458872E-16, 7.950000000000000178 ) ) ;
#12681=CARTESIAN_POINT ( 'NONE',  ( 66.93793019189809002, -6.110000000000001208, 1.637169565754158951 ) ) ;
#12700=CARTESIAN_POINT ( 'NONE',  ( 56.72959685856476142, -6.110000000000000320, -1.637169565754161393 ) ) ;
#12733=CARTESIAN_POINT ( 'NONE',  ( 107.9745968585647660, 1.637169565754164280, -6.109999999999996767 ) ) ;
#12744=CARTESIAN_POINT ( 'NONE',  ( 68.22916666666665719, 7.950000000000001954, -2.130196079827421762 ) ) ;
#12750=CARTESIAN_POINT ( 'NONE',  ( 87.18749999999998579, -5.819803920172573974, 5.819803920172573086 ) ) ;
#12756=CARTESIAN_POINT ( 'NONE',  ( 52.06293019189810423, 1.637169565754157174, 6.110000000000002984 ) ) ;
#12762=CARTESIAN_POINT ( 'NONE',  ( 90.85459685856478984, -1.637169565754161615, 6.110000000000000320 ) ) ;
#12781=CYLINDRICAL_SURFACE ( 'NONE', #86299, 4.375000000000001776 ) ;
#12807=CARTESIAN_POINT ( 'NONE',  ( 5.979278404433885363, 9.486416045811226994, -0.5818371488247532364 ) ) ;
#12828=CARTESIAN_POINT ( 'NONE',  ( 103.1833603837962130, -2.130196079827426203, 7.949999999999997513 ) ) ;
#12843=CARTESIAN_POINT ( 'NONE',  ( 92.75043019189810423, 3.055000000000002824, -5.291415217122919401 ) ) ;
#12867=CARTESIAN_POINT ( 'NONE',  ( 86.04209685856477563, 5.291415217122923842, -3.054999999999996163 ) ) ;
#12883=CARTESIAN_POINT ( 'NONE',  ( 83.32876352523143737, 0.000000000000000000, -6.109999999999998543 ) ) ;
#12912=DIRECTION ( 'NONE',  ( -1.000000000000000000, -0.000000000000000000, -0.000000000000000000 ) ) ;
#12922=LINE ( 'NONE', #123869, #120902 ) ;
#12933=CARTESIAN_POINT ( 'NONE',  ( 113.8962635252314186, 4.472830434245840259, -4.472830434245838482 ) ) ;
#12963=CARTESIAN_POINT ( 'NONE',  ( 80.70376352523145158, 6.109999999999999432, 1.122388791418549108E-15 ) ) ;
#12979=FACE_OUTER_BOUND ( 'NONE', #2426, .T. ) ;
#12988=EDGE_CURVE ( 'NONE', #98697, #20563, #119616, .T. ) ;
#13001=CARTESIAN_POINT ( 'NONE',  ( 47.32919371712955581, -3.975000000000001865, 6.884901960086284411 ) ) ;
#13009=CYLINDRICAL_SURFACE ( 'NONE', #119997, 7.950000000000000178 ) ;
#13015=VERTEX_POINT ( 'NONE', #83513 ) ;
#13016=CARTESIAN_POINT ( 'NONE',  ( 89.52083333333332860, 7.949999999999999289, 2.130196079827431532 ) ) ;
#13024=CARTESIAN_POINT ( 'NONE',  ( 27.00000000000000355, 0.000000000000000000, 0.000000000000000000 ) ) ;
#13032=CARTESIAN_POINT ( 'NONE',  ( 27.00000000000004974, 3.781023723404877579, 6.868722978355127573 ) ) ;
#13041=CARTESIAN_POINT ( 'NONE',  ( 124.2504301918981184, 3.055000000000002824, -5.291415217122919401 ) ) ;
#13051=CARTESIAN_POINT ( 'NONE',  ( 114.9745968585647660, 1.637169565754164058, -6.109999999999996767 ) ) ;
#13074=DIRECTION ( 'NONE',  ( -1.000000000000000000, -0.000000000000000000, -0.000000000000000000 ) ) ;
#13097=ADVANCED_FACE ( 'NONE', ( #8047 ), #107378, .T. ) ;
#13099=CARTESIAN_POINT ( 'NONE',  ( 51.39126352523145158, -4.472830434245838482, -4.472830434245838482 ) ) ;
#13128=CARTESIAN_POINT ( 'NONE',  ( 114.5370968585647802, -3.054999999999999272, -5.291415217122919401 ) ) ;
#13142=( BOUNDED_CURVE ( )  B_SPLINE_CURVE ( 2, ( #51075, #92404, #62667, #105426, #48940, #116319, #93143, #95273, #28619, #72872, #61965, #136631, #93850 ),
 .UNSPECIFIED., .F., .F. ) 
 B_SPLINE_CURVE_WITH_KNOTS ( ( 3, 2, 2, 2, 2, 2, 3 ),
 ( 0.5333333333333333259, 0.5361111111111110938, 0.5388888888888888618, 0.5416666666666666297, 0.5444444444444443976, 0.5472222222222222765, 0.5500000000000000444 ),
 .UNSPECIFIED. ) 
 CURVE ( )  GEOMETRIC_REPRESENTATION_ITEM ( )  RATIONAL_B_SPLINE_CURVE ( ( 1.000000000000000000, 0.9659258262890683122, 1.000000000000000000, 0.9659258262890683122, 1.000000000000000000, 0.9659258262890683122, 1.000000000000000000, 0.9659258262890683122, 1.000000000000000000, 0.9659258262890683122, 1.000000000000000000, 0.9659258262890683122, 1.000000000000000000 ) ) 
 REPRESENTATION_ITEM ( '' )  );
#13188=CARTESIAN_POINT ( 'NONE',  ( 122.3545968585647472, -1.637169565754161615, 6.110000000000000320 ) ) ;
#13191=CARTESIAN_POINT ( 'NONE',  ( 105.6625270504628844, 7.949999999999998401, 1.460391307983218338E-15 ) ) ;
#13200=CARTESIAN_POINT ( 'NONE',  ( 46.30836038379622721, 7.949999999999997513, 2.130196079827431088 ) ) ;
#13204=ORIENTED_EDGE ( 'NONE', *, *, #109435, .T. ) ;
#13206=CARTESIAN_POINT ( 'NONE',  ( 42.85416666666666430, -2.130196079827425315, -7.950000000000001066 ) ) ;
#13217=CARTESIAN_POINT ( 'NONE',  ( 38.20876352523143282, -7.482591942790329030E-16, 6.110000000000001208 ) ) ;
#13240=CARTESIAN_POINT ( 'NONE',  ( 60.28709685856478728, 3.054999999999997495, 5.291415217122919401 ) ) ;
#13248=EDGE_CURVE ( 'NONE', #141150, #142079, #4347, .T. ) ;
#13268=CARTESIAN_POINT ( 'NONE',  ( 77.20376352523145158, 6.109999999999998543, 1.122388791418548911E-15 ) ) ;
#13279=FACE_OUTER_BOUND ( 'NONE', #130437, .T. ) ;
#13281=CARTESIAN_POINT ( 'NONE',  ( 97.25000000000000000, -9.735942053221458872E-16, 7.950000000000000178 ) ) ;
#13298=CARTESIAN_POINT ( 'NONE',  ( 43.24586038379622721, 3.974999999999996980, 6.884901960086287964 ) ) ;
#13304=CARTESIAN_POINT ( 'NONE',  ( 120.5375270504628844, -9.735942053221456900E-16, 7.949999999999998401 ) ) ;
#13318=CARTESIAN_POINT ( 'NONE',  ( 28.85416666666666075, -2.130196079827425759, -7.950000000000000178 ) ) ;
#13331=CARTESIAN_POINT ( 'NONE',  ( 25.75309147121574327, -1.701477371937609728, -6.350000000000015632 ) ) ;
#13348=CARTESIAN_POINT ( 'NONE',  ( 51.97459685856478728, 1.637169565754164280, -6.109999999999997655 ) ) ;
#13360=CARTESIAN_POINT ( 'NONE',  ( 0.000000000000000000, 0.000000000000000000, 0.000000000000000000 ) ) ;
#13369=CARTESIAN_POINT ( 'NONE',  ( 71.68336038379621300, -2.130196079827426203, 7.949999999999997513 ) ) ;
#13374=CARTESIAN_POINT ( 'NONE',  ( 77.56250000000000000, -5.819803920172572198, -5.819803920172573086 ) ) ;
#13384=CARTESIAN_POINT ( 'NONE',  ( 61.54209685856476852, 5.291415217122923842, -3.054999999999996163 ) ) ;
#13386=FACE_BOUND ( 'NONE', #79579, .T. ) ;
#13394=CARTESIAN_POINT ( 'NONE',  ( 85.58333333333332860, 6.884901960086290629, -3.974999999999994316 ) ) ;
#13403=CARTESIAN_POINT ( 'NONE',  ( 58.18793019189811133, 6.110000000000002984, -1.637169565754156730 ) ) ;
#13432=CARTESIAN_POINT ( 'NONE',  ( 99.37043019189812298, -3.055000000000001492, 5.291415217122917625 ) ) ;
#13433=ORIENTED_EDGE ( 'NONE', *, *, #79927, .F. ) ;
#13436=DIRECTION ( 'NONE',  ( 0.000000000000000000, 0.000000000000000000, 1.000000000000000000 ) ) ;
#13445=DIRECTION ( 'NONE',  ( -1.000000000000000000, -0.000000000000000000, -0.000000000000000000 ) ) ;
#13458=CARTESIAN_POINT ( 'NONE',  ( 58.47959685856477563, 6.109999999999999432, 1.637169565754164280 ) ) ;
#13461=CARTESIAN_POINT ( 'NONE',  ( 92.16709685856477563, -3.055000000000000160, -5.291415217122921177 ) ) ;
#13471=CARTESIAN_POINT ( 'NONE',  ( 125.9120968585647802, 5.291415217122922066, -3.054999999999995275 ) ) ;
#13472=ORIENTED_EDGE ( 'NONE', *, *, #43024, .T. ) ;
#13504=CARTESIAN_POINT ( 'NONE',  ( 58.16666666666665719, 6.884901960086285300, 3.975000000000003642 ) ) ;
#13509=CARTESIAN_POINT ( 'NONE',  ( 6.399664195087332530, 9.300955700193000553, 1.952836266634600415 ) ) ;
#13535=CARTESIAN_POINT ( 'NONE',  ( 107.4125270504628986, -7.949999999999998401, -4.867971026610728450E-16 ) ) ;
#13552=CARTESIAN_POINT ( 'NONE',  ( 98.00043019189810423, -3.055000000000002380, 5.291415217122920289 ) ) ;
#13575=CARTESIAN_POINT ( 'NONE',  ( 82.54209685856478984, 5.291415217122923842, -3.054999999999996163 ) ) ;
#13586=CARTESIAN_POINT ( 'NONE',  ( 80.55793019189812298, 6.110000000000000320, -1.637169565754156064 ) ) ;
#13640=ORIENTED_EDGE ( 'NONE', *, *, #106487, .T. ) ;
#13642=CARTESIAN_POINT ( 'NONE',  ( 94.47916666666665719, -7.950000000000000178, 2.130196079827424427 ) ) ;
#13644=CARTESIAN_POINT ( 'NONE',  ( 116.9587635252314470, 0.000000000000000000, -6.110000000000001208 ) ) ;
#13648=FACE_OUTER_BOUND ( 'NONE', #17279, .T. ) ;
#13676=EDGE_CURVE ( 'NONE', #83993, #46474, #9918, .T. ) ;
#13700=EDGE_CURVE ( 'NONE', #32075, #79314, #108125, .T. ) ;
#13718=CARTESIAN_POINT ( 'NONE',  ( 93.60416666666665719, 2.130196079827422206, 7.950000000000001954 ) ) ;
#13725=CARTESIAN_POINT ( 'NONE',  ( 10.32500000000000107, 8.432637487761466488, 4.375000000000001776 ) ) ;
#13747=CARTESIAN_POINT ( 'NONE',  ( 108.2087635252314470, -7.482591942790329030E-16, 6.110000000000001208 ) ) ;
#13755=CARTESIAN_POINT ( 'NONE',  ( 114.2454301918981230, -5.291415217122918513, -3.055000000000000160 ) ) ;
#13760=CARTESIAN_POINT ( 'NONE',  ( 97.68750000000000000, -5.819803920172573974, 5.819803920172573086 ) ) ;
#13768=CARTESIAN_POINT ( 'NONE',  ( 30.68293019189811943, -1.637169565754158951, -6.109999999999998543 ) ) ;
#13790=ORIENTED_EDGE ( 'NONE', *, *, #52154, .F. ) ;
#13791=CARTESIAN_POINT ( 'NONE',  ( 63.80836038379621300, 7.949999999999996625, 2.130196079827431088 ) ) ;
#13801=CARTESIAN_POINT ( 'NONE',  ( 42.64126352523145158, 4.472830434245835818, 4.472830434245840259 ) ) ;
#13809=AXIS2_PLACEMENT_3D ( 'NONE', #35554, #12318, #44268 ) ;
#13817=VERTEX_POINT ( 'NONE', #119322 ) ;
#13839=CARTESIAN_POINT ( 'NONE',  ( 112.2037635252314516, 6.109999999999999432, 1.122388791418549108E-15 ) ) ;
#13886=CARTESIAN_POINT ( 'NONE',  ( 120.7291666666666572, 7.950000000000001954, -2.130196079827421762 ) ) ;
#13904=CARTESIAN_POINT ( 'NONE',  ( 110.3962635252314328, 4.472830434245840259, -4.472830434245839371 ) ) ;
#13915=CARTESIAN_POINT ( 'NONE',  ( 47.91252705046289151, -7.949999999999998401, -4.867971026610728450E-16 ) ) ;
#13921=CARTESIAN_POINT ( 'NONE',  ( 35.70833333333332860, -3.974999999999999201, -6.884901960086287964 ) ) ;
#13930=CARTESIAN_POINT ( 'NONE',  ( 36.02126352523142572, -4.472830434245839371, -4.472830434245840259 ) ) ;
#13945=CARTESIAN_POINT ( 'NONE',  ( 38.43336038379621300, 2.130196079827431532, -7.949999999999996625 ) ) ;
#13952=CARTESIAN_POINT ( 'NONE',  ( 54.45376352523144448, -6.109999999999998543, -3.741295971395162543E-16 ) ) ;
#13982=CARTESIAN_POINT ( 'NONE',  ( 68.30793019189810877, -6.109999999999998543, 1.637169565754158507 ) ) ;
#13990=( BOUNDED_CURVE ( )  B_SPLINE_CURVE ( 2, ( #60755, #107057, #6265, #73718, #49854, #94031, #83924, #138270, #38954, #83177, #85288, #117196, #139725 ),
 .UNSPECIFIED., .F., .F. ) 
 B_SPLINE_CURVE_WITH_KNOTS ( ( 3, 2, 2, 2, 2, 2, 3 ),
 ( 0.7166666666666666741, 0.7194444444444444420, 0.7222222222222222099, 0.7249999999999999778, 0.7277777777777777457, 0.7305555555555555136, 0.7333333333333332815 ),
 .UNSPECIFIED. ) 
 CURVE ( )  GEOMETRIC_REPRESENTATION_ITEM ( )  RATIONAL_B_SPLINE_CURVE ( ( 1.000000000000000000, 0.9659258262890683122, 1.000000000000000000, 0.9659258262890683122, 1.000000000000000000, 0.9659258262890683122, 1.000000000000000000, 0.9659258262890683122, 1.000000000000000000, 0.9659258262890683122, 1.000000000000000000, 0.9659258262890683122, 1.000000000000000000 ) ) 
 REPRESENTATION_ITEM ( '' )  );
#14009=CARTESIAN_POINT ( 'NONE',  ( 29.31293019189811133, -1.637169565754159617, -6.110000000000001208 ) ) ;
#14053=CARTESIAN_POINT ( 'NONE',  ( 127.0000000000000000, 0.000000000000000000, 0.000000000000000000 ) ) ;
#14069=CARTESIAN_POINT ( 'NONE',  ( 55.18293019189810877, -1.637169565754159173, -6.109999999999999432 ) ) ;
#14091=CARTESIAN_POINT ( 'NONE',  ( 75.18336038379624142, -2.130196079827426203, 7.949999999999997513 ) ) ;
#14096=CARTESIAN_POINT ( 'NONE',  ( 74.06249999999998579, -5.819803920172572198, -5.819803920172573086 ) ) ;
#14107=CARTESIAN_POINT ( 'NONE',  ( 67.08376352523143282, -6.110000000000001208, -3.741295971395164515E-16 ) ) ;
#14129=CARTESIAN_POINT ( 'NONE',  ( 58.04209685856477563, 5.291415217122923842, -3.054999999999996163 ) ) ;
#14137=CARTESIAN_POINT ( 'NONE',  ( 54.37499999999999289, 7.950000000000000178, 1.460391307983218535E-15 ) ) ;
#14158=CARTESIAN_POINT ( 'NONE',  ( 37.55836038379621300, -7.949999999999996625, -2.130196079827426203 ) ) ;
#14167=CARTESIAN_POINT ( 'NONE',  ( 104.4745968585647802, 1.637169565754164280, -6.109999999999996767 ) ) ;
#14192=CARTESIAN_POINT ( 'NONE',  ( 51.33376352523143282, 6.110000000000001208, 1.122388791418549305E-15 ) ) ;
#14198=CARTESIAN_POINT ( 'NONE',  ( 93.18793019189809002, 6.110000000000002984, -1.637169565754156730 ) ) ;
#14250=CARTESIAN_POINT ( 'NONE',  ( 6.093169818762517842, 9.434785192573073687, 1.147133048873354211 ) ) ;
#14274=CARTESIAN_POINT ( 'NONE',  ( 106.1000270504628986, 5.819803920172570422, 5.819803920172574863 ) ) ;
#14289=ORIENTED_EDGE ( 'NONE', *, *, #48765, .F. ) ;
#14290=CARTESIAN_POINT ( 'NONE',  ( 94.79209685856476142, -5.291415217122921177, 3.054999999999999272 ) ) ;
#14312=CARTESIAN_POINT ( 'NONE',  ( 82.97959685856476142, 6.109999999999999432, 1.637169565754164280 ) ) ;
#14326=CARTESIAN_POINT ( 'NONE',  ( 74.87043019189812298, -3.055000000000001492, 5.291415217122917625 ) ) ;
#14356=VECTOR ( 'NONE', #64092, 1000.000000000000000 ) ;
#14364=AXIS2_PLACEMENT_3D ( 'NONE', #128072, #10354, #126598 ) ;
#14365=DIRECTION ( 'NONE',  ( -1.000000000000000000, -0.000000000000000000, -0.000000000000000000 ) ) ;
#14382=CARTESIAN_POINT ( 'NONE',  ( 118.8545968585647756, -1.637169565754161615, 6.110000000000000320 ) ) ;
#14445=VERTEX_POINT ( 'NONE', #100287 ) ;
#14466=CARTESIAN_POINT ( 'NONE',  ( 92.58333333333332860, 6.884901960086290629, -3.974999999999994316 ) ) ;
#14474=CARTESIAN_POINT ( 'NONE',  ( 11.47583603616349102, 8.506184923238587103, 4.230711047486125587 ) ) ;
#14479=CARTESIAN_POINT ( 'NONE',  ( 125.7014274047528488, -0.5088013136202494957, -7.748369483595296536 ) ) ;
#14490=CARTESIAN_POINT ( 'NONE',  ( 112.8754301918981042, -5.291415217122920289, -3.055000000000001492 ) ) ;
#14499=CARTESIAN_POINT ( 'NONE',  ( 107.5370968585647944, -3.054999999999998828, -5.291415217122919401 ) ) ;
#14540=EDGE_CURVE ( 'NONE', #74280, #24706, #98831, .T. ) ;
#14550=CARTESIAN_POINT ( 'NONE',  ( 37.39126352523144448, -4.472830434245838482, -4.472830434245838482 ) ) ;
#14575=DIRECTION ( 'NONE',  ( 0.000000000000000000, 0.000000000000000000, 1.000000000000000000 ) ) ;
#14583=CARTESIAN_POINT ( 'NONE',  ( 102.2870968585647802, 3.054999999999997939, 5.291415217122920289 ) ) ;
#14617=CARTESIAN_POINT ( 'NONE',  ( 52.33333333333332860, -6.884901960086287964, 3.974999999999998312 ) ) ;
#14635=CARTESIAN_POINT ( 'NONE',  ( 120.5833333333333286, 6.884901960086290629, -3.974999999999994316 ) ) ;
#14649=CARTESIAN_POINT ( 'NONE',  ( 112.1462635252314328, -4.472830434245840259, 4.472830434245839371 ) ) ;
#14658=PRODUCT_DEFINITION ( 'UNKNOWN', '', #47199, #50204 ) ;
#14659=CARTESIAN_POINT ( 'NONE',  ( 49.37086038379622011, 6.884901960086289741, -3.974999999999993427 ) ) ;
#14665=CARTESIAN_POINT ( 'NONE',  ( 40.52083333333332860, 7.949999999999999289, 2.130196079827431532 ) ) ;
#14672=CARTESIAN_POINT ( 'NONE',  ( 0.000000000000000000, 0.000000000000000000, 0.000000000000000000 ) ) ;
#14676=CARTESIAN_POINT ( 'NONE',  ( 31.64626352523143638, -4.472830434245840259, 4.472830434245839371 ) ) ;
#14685=CARTESIAN_POINT ( 'NONE',  ( 62.25000000000000000, -9.735942053221458872E-16, 7.950000000000000178 ) ) ;
#14694=CARTESIAN_POINT ( 'NONE',  ( 53.87043019189811588, -3.055000000000001492, 5.291415217122917625 ) ) ;
#14696=CARTESIAN_POINT ( 'NONE',  ( 124.0833333333333428, 6.884901960086290629, -3.974999999999994316 ) ) ;
#14723=CARTESIAN_POINT ( 'NONE',  ( 66.12043019189812298, 3.055000000000001936, -5.291415217122916737 ) ) ;
#14733=CARTESIAN_POINT ( 'NONE',  ( 102.3541666666666714, -2.130196079827387567, -7.950000000000023270 ) ) ;
#14749=ADVANCED_FACE ( 'NONE', ( #59314, #35423 ), #134732, .F. ) ;
#14782=CARTESIAN_POINT ( 'NONE',  ( 25.46142480454906121, -4.648522628062372597, -4.648522628062373485 ) ) ;
#14784=LINE ( 'NONE', #308, #135083 ) ;
#14787=CARTESIAN_POINT ( 'NONE',  ( 65.70419371712955581, -6.884901960086285300, -3.975000000000000089 ) ) ;
#14796=CARTESIAN_POINT ( 'NONE',  ( 60.72459685856477307, -1.637169565754161171, 6.109999999999998543 ) ) ;
#14813=ORIENTED_EDGE ( 'NONE', *, *, #6013, .T. ) ;
#14818=CARTESIAN_POINT ( 'NONE',  ( 78.10002705046289861, 5.819803920172570422, 5.819803920172574863 ) ) ;
#14822=CARTESIAN_POINT ( 'NONE',  ( 65.75000000000000000, -9.735942053221458872E-16, 7.950000000000000178 ) ) ;
#14826=EDGE_LOOP ( 'NONE', ( #31792, #113385, #126374, #19664, #139919, #3177 ) ) ;
#14831=CARTESIAN_POINT ( 'NONE',  ( 53.81293019189810423, -1.637169565754159617, -6.110000000000001208 ) ) ;
#14883=CARTESIAN_POINT ( 'NONE',  ( 91.49543019189812298, 5.291415217122916737, 3.055000000000001936 ) ) ;
#14905=CARTESIAN_POINT ( 'NONE',  ( 45.64626352523142572, -4.472830434245840259, 4.472830434245838482 ) ) ;
#14921=CARTESIAN_POINT ( 'NONE',  ( 124.8912635252314516, -4.472830434245839371, -4.472830434245839371 ) ) ;
#14974=CARTESIAN_POINT ( 'NONE',  ( 102.4541937171295700, 6.884901960086283523, 3.975000000000002753 ) ) ;
#14993=CARTESIAN_POINT ( 'NONE',  ( 96.54209685856477563, 5.291415217122923842, -3.054999999999996163 ) ) ;
#15014=CARTESIAN_POINT ( 'NONE',  ( 85.45876352523143282, 0.000000000000000000, -6.110000000000001208 ) ) ;
#15026=CARTESIAN_POINT ( 'NONE',  ( 75.59959685856478018, -6.109999999999997655, -1.637169565754160283 ) ) ;
#15031=EDGE_CURVE ( 'NONE', #133316, #83142, #68399, .T. ) ;
#15076=CARTESIAN_POINT ( 'NONE',  ( 120.4587635252314328, 0.000000000000000000, -6.110000000000001208 ) ) ;
#15077=CYLINDRICAL_SURFACE ( 'NONE', #81934, 7.950000000000000178 ) ;
#15102=CARTESIAN_POINT ( 'NONE',  ( 14.55624338558763853, -9.434519525233701742, 1.149922814568643981 ) ) ;
#15136=CARTESIAN_POINT ( 'NONE',  ( 29.22459685856478018, -1.637169565754161171, 6.109999999999998543 ) ) ;
#15151=( BOUNDED_CURVE ( )  B_SPLINE_CURVE ( 2, ( #63290, #29185, #16134, #106726, #127812, #74129, #61844, #27042, #129199, #116908, #6674, #29886, #118323 ),
 .UNSPECIFIED., .F., .T. ) 
 B_SPLINE_CURVE_WITH_KNOTS ( ( 3, 2, 2, 2, 2, 2, 3 ),
 ( 0.6999999999999999556, 0.7027777777777777235, 0.7055555555555556024, 0.7083333333333333703, 0.7111111111111111382, 0.7138888888888889062, 0.7166666666666666741 ),
 .UNSPECIFIED. ) 
 CURVE ( )  GEOMETRIC_REPRESENTATION_ITEM ( )  RATIONAL_B_SPLINE_CURVE ( ( 1.000000000000000000, 0.9659258262890683122, 1.000000000000000000, 0.9659258262890683122, 1.000000000000000000, 0.9659258262890683122, 1.000000000000000000, 0.9659258262890683122, 1.000000000000000000, 0.9659258262890683122, 1.000000000000000000, 0.9659258262890683122, 1.000000000000000000 ) ) 
 REPRESENTATION_ITEM ( '' )  );
#15152=CARTESIAN_POINT ( 'NONE',  ( 87.91666666666667140, -6.884901960086287076, -3.975000000000000977 ) ) ;
#15179=CARTESIAN_POINT ( 'NONE',  ( 109.8129301918981042, -1.637169565754159617, -6.110000000000001208 ) ) ;
#15190=CARTESIAN_POINT ( 'NONE',  ( 108.1204301918981230, 3.055000000000001936, -5.291415217122916737 ) ) ;
#15222=ORIENTED_EDGE ( 'NONE', *, *, #130896, .T. ) ;
#15229=CARTESIAN_POINT ( 'NONE',  ( 39.87043019189810877, -3.055000000000001492, 5.291415217122917625 ) ) ;
#15260=CARTESIAN_POINT ( 'NONE',  ( 97.47459685856478018, 1.637169565754164280, -6.109999999999997655 ) ) ;
#15310=CARTESIAN_POINT ( 'NONE',  ( 121.6041666666666430, 2.130196079827422206, 7.950000000000001954 ) ) ;
#15323=CARTESIAN_POINT ( 'NONE',  ( 110.8337635252314470, 6.110000000000001208, 1.122388791418549305E-15 ) ) ;
#15332=CARTESIAN_POINT ( 'NONE',  ( 41.05836038379621300, -7.949999999999997513, -2.130196079827425759 ) ) ;
#15338=CARTESIAN_POINT ( 'NONE',  ( 37.31250000000000000, 5.819803920172571310, 5.819803920172575751 ) ) ;
#15348=CARTESIAN_POINT ( 'NONE',  ( 33.39626352523143993, 4.472830434245840259, -4.472830434245839371 ) ) ;
#15367=CARTESIAN_POINT ( 'NONE',  ( 44.53709685856478728, -3.054999999999998828, -5.291415217122919401 ) ) ;
#15396=CARTESIAN_POINT ( 'NONE',  ( 70.20376352523143737, 6.109999999999998543, 1.122388791418548911E-15 ) ) ;
#15429=CARTESIAN_POINT ( 'NONE',  ( 119.9541937171295700, 6.884901960086283523, 3.975000000000002753 ) ) ;
#15439=B_SPLINE_CURVE_WITH_KNOTS ( 'NONE', 3,
 ( #21258, #32880, #134319, #123465 ),
 .UNSPECIFIED., .F., .F.,
 ( 4, 4 ),
 ( 0.001975484284630000132, 0.002273591611137678378 ),
 .UNSPECIFIED. ) ;
#15450=CYLINDRICAL_SURFACE ( 'NONE', #57579, 6.349999999999999645 ) ;
#15474=CARTESIAN_POINT ( 'NONE',  ( 45.99543019189810877, 5.291415217122917625, 3.055000000000002380 ) ) ;
#15485=EDGE_CURVE ( 'NONE', #93941, #13015, #38728, .T. ) ;
#15496=CARTESIAN_POINT ( 'NONE',  ( 65.99586038379622721, -3.974999999999998312, -6.884901960086286188 ) ) ;
#15501=CARTESIAN_POINT ( 'NONE',  ( 59.91666666666665719, -6.884901960086287076, -3.975000000000000977 ) ) ;
#15509=CARTESIAN_POINT ( 'NONE',  ( 56.29209685856477563, -5.291415217122921177, 3.054999999999999272 ) ) ;
#15533=CARTESIAN_POINT ( 'NONE',  ( 110.0375270504628986, -9.735942053221456900E-16, 7.949999999999998401 ) ) ;
#15536=ORIENTED_EDGE ( 'NONE', *, *, #38363, .F. ) ;
#15543=CARTESIAN_POINT ( 'NONE',  ( 62.05836038379622011, -7.949999999999996625, -2.130196079827426203 ) ) ;
#15558=CARTESIAN_POINT ( 'NONE',  ( 94.70376352523145158, 6.109999999999998543, 1.122388791418548911E-15 ) ) ;
#15582=CARTESIAN_POINT ( 'NONE',  ( 44.62543019189810423, 5.291415217122919401, 3.055000000000002824 ) ) ;
#15620=EDGE_CURVE ( 'NONE', #25494, #82607, #137055, .T. ) ;
#15630=CARTESIAN_POINT ( 'NONE',  ( 77.34959685856478018, 6.109999999999997655, 1.637169565754163836 ) ) ;
#15632=CARTESIAN_POINT ( 'NONE',  ( 74.74586038379622721, 3.974999999999996980, 6.884901960086287964 ) ) ;
#15652=CARTESIAN_POINT ( 'NONE',  ( 121.7041937171295700, -6.884901960086285300, -3.975000000000000089 ) ) ;
#15658=CARTESIAN_POINT ( 'NONE',  ( 103.0375270504628986, -9.735942053221456900E-16, 7.949999999999998401 ) ) ;
#15672=CARTESIAN_POINT ( 'NONE',  ( 81.37543019189810423, -5.291415217122920289, -3.055000000000001492 ) ) ;
#15679=( BOUNDED_CURVE ( )  B_SPLINE_CURVE ( 2, ( #38668, #139443, #61185, #93042, #17598, #137272, #50973, #37970, #60448, #59726, #18298, #105335, #103886 ),
 .UNSPECIFIED., .F., .T. ) 
 B_SPLINE_CURVE_WITH_KNOTS ( ( 3, 2, 2, 2, 2, 2, 3 ),
 ( 0.1666666666666666574, 0.1694444444444444531, 0.1722222222222222210, 0.1749999999999999889, 0.1777777777777778123, 0.1805555555555555802, 0.1833333333333333481 ),
 .UNSPECIFIED. ) 
 CURVE ( )  GEOMETRIC_REPRESENTATION_ITEM ( )  RATIONAL_B_SPLINE_CURVE ( ( 1.000000000000000000, 0.9659258262890683122, 1.000000000000000000, 0.9659258262890683122, 1.000000000000000000, 0.9659258262890683122, 1.000000000000000000, 0.9659258262890683122, 1.000000000000000000, 0.9659258262890683122, 1.000000000000000000, 0.9659258262890679791, 1.000000000000000444 ) ) 
 REPRESENTATION_ITEM ( '' )  );
#15695=CARTESIAN_POINT ( 'NONE',  ( 80.64626352523141861, -4.472830434245840259, 4.472830434245839371 ) ) ;
#15704=CARTESIAN_POINT ( 'NONE',  ( 75.16209685856478018, -5.291415217122919401, 3.054999999999997939 ) ) ;
#15711=CARTESIAN_POINT ( 'NONE',  ( 64.87499999999998579, 7.950000000000000178, 1.460391307983218535E-15 ) ) ;
#15744=CARTESIAN_POINT ( 'NONE',  ( 74.52126352523143282, -4.472830434245838482, -4.472830434245840259 ) ) ;
#15750=CARTESIAN_POINT ( 'NONE',  ( 110.2504301918981042, 3.055000000000002824, -5.291415217122919401 ) ) ;
#15751=CARTESIAN_POINT ( 'NONE',  ( 127.0000000000000000, 1.864289179696898779, 6.174700466780991270 ) ) ;
#15783=CARTESIAN_POINT ( 'NONE',  ( 13.21415715735881058, -8.911859315205598264, -3.297485585150703002 ) ) ;
#15813=CARTESIAN_POINT ( 'NONE',  ( 97.78752705046289861, 0.000000000000000000, -7.949999999999998401 ) ) ;
#15819=CARTESIAN_POINT ( 'NONE',  ( 106.2916666666666714, 3.975000000000003642, -6.884901960086285300 ) ) ;
#15820=CARTESIAN_POINT ( 'NONE',  ( 27.32876352523144803, 0.000000000000000000, -6.109999999999999432 ) ) ;
#15836=CARTESIAN_POINT ( 'NONE',  ( 94.18749999999998579, -5.819803920172573086, 5.819803920172572198 ) ) ;
#15850=CARTESIAN_POINT ( 'NONE',  ( 126.7599512408517057, 4.946259330407210442, 4.511684350628299534 ) ) ;
#15857=CARTESIAN_POINT ( 'NONE',  ( 160.0000000000000000, 0.000000000000000000, 6.349999999999997868 ) ) ;
#15866=CARTESIAN_POINT ( 'NONE',  ( 114.6254301918981042, 5.291415217122919401, 3.055000000000002824 ) ) ;
#15876=CARTESIAN_POINT ( 'NONE',  ( 100.0995968585647944, -6.109999999999997655, -1.637169565754160283 ) ) ;
#15887=ORIENTED_EDGE ( 'NONE', *, *, #128931, .T. ) ;
#15925=CARTESIAN_POINT ( 'NONE',  ( 36.51626352523145158, -4.472830434245838482, 4.472830434245838482 ) ) ;
#15943=ORIENTED_EDGE ( 'NONE', *, *, #84424, .F. ) ;
#15964=CARTESIAN_POINT ( 'NONE',  ( 100.6829301918981230, -1.637169565754159173, -6.109999999999999432 ) ) ;
#16007=EDGE_CURVE ( 'NONE', #141150, #76474, #58089, .T. ) ;
#16021=CARTESIAN_POINT ( 'NONE',  ( 123.6458333333333286, 2.130196079827431976, -7.949999999999999289 ) ) ;
#16030=CARTESIAN_POINT ( 'NONE',  ( 117.3962635252314470, 4.472830434245840259, -4.472830434245839371 ) ) ;
#16038=CARTESIAN_POINT ( 'NONE',  ( 38.72502705046289151, 5.819803920172573086, -5.819803920172572198 ) ) ;
#16044=CARTESIAN_POINT ( 'NONE',  ( 38.47916666666665009, -7.950000000000001066, 2.130196079827424427 ) ) ;
#16053=CARTESIAN_POINT ( 'NONE',  ( 33.25043019189810423, 3.055000000000002824, -5.291415217122919401 ) ) ;
#16073=CARTESIAN_POINT ( 'NONE',  ( 52.70376352523144448, 6.109999999999998543, 1.122388791418548911E-15 ) ) ;
#16075=CARTESIAN_POINT ( 'NONE',  ( 124.9583333333333428, 3.974999999999997424, 6.884901960086288852 ) ) ;
#16110=CARTESIAN_POINT ( 'NONE',  ( 68.45376352523143737, -6.109999999999998543, -3.741295971395162543E-16 ) ) ;
#16134=CARTESIAN_POINT ( 'NONE',  ( 55.49586038379622721, -3.974999999999998312, -6.884901960086286188 ) ) ;
#16189=CARTESIAN_POINT ( 'NONE',  ( 47.45376352523145158, -6.109999999999999432, -3.741295971395163529E-16 ) ) ;
#16211=CARTESIAN_POINT ( 'NONE',  ( 116.7916666666666714, 3.975000000000003642, -6.884901960086285300 ) ) ;
#16212=CARTESIAN_POINT ( 'NONE',  ( 63.07919371712955581, 3.975000000000002753, -6.884901960086283523 ) ) ;
#16217=CARTESIAN_POINT ( 'NONE',  ( 65.02083333333334281, 7.949999999999999289, 2.130196079827431532 ) ) ;
#16220=AXIS2_PLACEMENT_3D ( 'NONE', #111826, #121251, #44451 ) ;
#16225=CARTESIAN_POINT ( 'NONE',  ( 59.06293019189809712, 1.637169565754157174, 6.110000000000002984 ) ) ;
#16236=CARTESIAN_POINT ( 'NONE',  ( 100.8500270504628986, -5.819803920172573086, -5.819803920172573086 ) ) ;
#16275=( BOUNDED_CURVE ( )  B_SPLINE_CURVE ( 2, ( #40063, #61805, #95106, #127016, #16853, #18230, #84281, #96507, #105278, #7371, #52319, #128476, #29148 ),
 .UNSPECIFIED., .F., .T. ) 
 B_SPLINE_CURVE_WITH_KNOTS ( ( 3, 2, 2, 2, 2, 2, 3 ),
 ( 0.8000000000000000444, 0.8027777777777778123, 0.8055555555555555802, 0.8083333333333333481, 0.8111111111111111160, 0.8138888888888888840, 0.8166666666666666519 ),
 .UNSPECIFIED. ) 
 CURVE ( )  GEOMETRIC_REPRESENTATION_ITEM ( )  RATIONAL_B_SPLINE_CURVE ( ( 1.000000000000000000, 0.9659258262890683122, 1.000000000000000000, 0.9659258262890683122, 1.000000000000000000, 0.9659258262890683122, 1.000000000000000000, 0.9659258262890683122, 1.000000000000000000, 0.9659258262890683122, 1.000000000000000000, 0.9659258262890683122, 1.000000000000000000 ) ) 
 REPRESENTATION_ITEM ( '' )  );
#16282=CARTESIAN_POINT ( 'NONE',  ( 91.93293019189812298, 1.637169565754156508, 6.110000000000000320 ) ) ;
#16286=EDGE_CURVE ( 'NONE', #79882, #83402, #34931, .T. ) ;
#16296=EDGE_CURVE ( 'NONE', #29769, #13015, #12922, .T. ) ;
#16313=CARTESIAN_POINT ( 'NONE',  ( 47.68793019189809712, 6.110000000000002984, -1.637169565754156730 ) ) ;
#16360=CARTESIAN_POINT ( 'NONE',  ( 74.57876352523145158, -7.482591942790327058E-16, 6.109999999999999432 ) ) ;
#16389=CARTESIAN_POINT ( 'NONE',  ( 93.26669371712957002, -7.949999999999999289, 2.130196079827424427 ) ) ;
#16390=CARTESIAN_POINT ( 'NONE',  ( 72.16666666666665719, 6.884901960086285300, 3.975000000000003642 ) ) ;
#16398=CARTESIAN_POINT ( 'NONE',  ( 0.000000000000000000, 0.000000000000000000, 6.350000000000004086 ) ) ;
#16405=CARTESIAN_POINT ( 'NONE',  ( 81.81293019189810423, -1.637169565754159617, -6.110000000000001208 ) ) ;
#16423=DIRECTION ( 'NONE',  ( 0.000000000000000000, 0.000000000000000000, 1.000000000000000000 ) ) ;
#16427=CARTESIAN_POINT ( 'NONE',  ( 73.20876352523143282, -7.482591942790329030E-16, 6.110000000000001208 ) ) ;
#16453=CARTESIAN_POINT ( 'NONE',  ( 25.22959685856476142, -6.110000000000000320, -1.637169565754161393 ) ) ;
#16491=CARTESIAN_POINT ( 'NONE',  ( 69.85459685856476142, -1.637169565754161615, 6.110000000000000320 ) ) ;
#16497=CARTESIAN_POINT ( 'NONE',  ( 112.7295968585647756, -6.110000000000000320, -1.637169565754161393 ) ) ;
#16516=CARTESIAN_POINT ( 'NONE',  ( 114.1208603837962414, -6.884901960086286188, 3.974999999999997424 ) ) ;
#16520=CARTESIAN_POINT ( 'NONE',  ( 113.1458333333333428, 2.130196079827451516, -7.949999999999988631 ) ) ;
#16566=CARTESIAN_POINT ( 'NONE',  ( 119.6625270504628986, 7.949999999999998401, 1.460391307983218338E-15 ) ) ;
#16583=CARTESIAN_POINT ( 'NONE',  ( 79.45833333333332860, 3.974999999999997424, 6.884901960086288852 ) ) ;
#16585=CARTESIAN_POINT ( 'NONE',  ( 96.03752705046289861, -9.735942053221456900E-16, 7.949999999999998401 ) ) ;
#16615=CARTESIAN_POINT ( 'NONE',  ( 111.1254301918981042, 5.291415217122919401, 3.055000000000002824 ) ) ;
#16625=CARTESIAN_POINT ( 'NONE',  ( 108.2662635252314374, 4.472830434245839371, -4.472830434245838482 ) ) ;
#16656=CARTESIAN_POINT ( 'NONE',  ( 113.3704301918981230, -3.055000000000001492, 5.291415217122917625 ) ) ;
#16678=CARTESIAN_POINT ( 'NONE',  ( 33.59959685856478018, -6.109999999999997655, -1.637169565754160283 ) ) ;
#16720=CARTESIAN_POINT ( 'NONE',  ( 103.3079301918981088, -6.109999999999999432, 1.637169565754158507 ) ) ;
#16751=VERTEX_POINT ( 'NONE', #13281 ) ;
#16771=CARTESIAN_POINT ( 'NONE',  ( 115.9166666666666714, -6.884901960086287076, -3.975000000000000977 ) ) ;
#16783=CARTESIAN_POINT ( 'NONE',  ( 115.9379301918980900, -6.110000000000001208, 1.637169565754158951 ) ) ;
#16796=CARTESIAN_POINT ( 'NONE',  ( 37.12086038379622011, -6.884901960086286188, 3.974999999999997424 ) ) ;
#16800=CARTESIAN_POINT ( 'NONE',  ( 32.35416666666665009, -2.130196079827425315, -7.950000000000001066 ) ) ;
#16816=CARTESIAN_POINT ( 'NONE',  ( 28.72959685856476497, -6.110000000000000320, -1.637169565754161393 ) ) ;
#16817=ORIENTED_EDGE ( 'NONE', *, *, #13676, .T. ) ;
#16819=ORIENTED_EDGE ( 'NONE', *, *, #96974, .F. ) ;
#16828=CARTESIAN_POINT ( 'NONE',  ( 51.77126352523143993, 4.472830434245839371, 4.472830434245842035 ) ) ;
#16837=CARTESIAN_POINT ( 'NONE',  ( 50.22459685856477307, -1.637169565754160949, 6.109999999999997655 ) ) ;
#16839=CARTESIAN_POINT ( 'NONE',  ( 124.2291666666666714, 7.950000000000001954, -2.130196079827421762 ) ) ;
#16853=CARTESIAN_POINT ( 'NONE',  ( 44.70419371712955581, -6.884901960086285300, -3.975000000000000089 ) ) ;
#16859=EDGE_CURVE ( 'NONE', #142079, #10908, #16883, .T. ) ;
#16870=CARTESIAN_POINT ( 'NONE',  ( 69.47459685856476597, 1.637169565754164280, -6.109999999999996767 ) ) ;
#16883=LINE ( 'NONE', #103850, #67873 ) ;
#16894=CARTESIAN_POINT ( 'NONE',  ( 29.43749999999998934, 5.819803920172574863, -5.819803920172573086 ) ) ;
#16944=CARTESIAN_POINT ( 'NONE',  ( 49.34959685856478728, 6.109999999999997655, 1.637169565754163836 ) ) ;
#16967=DIRECTION ( 'NONE',  ( -1.000000000000000000, -0.000000000000000000, -0.000000000000000000 ) ) ;
#16971=CARTESIAN_POINT ( 'NONE',  ( 65.41252705046289861, -7.949999999999998401, -4.867971026610728450E-16 ) ) ;
#16976=CARTESIAN_POINT ( 'NONE',  ( 67.64583333333330017, 2.130196079827431976, -7.949999999999999289 ) ) ;
#16983=CARTESIAN_POINT ( 'NONE',  ( 33.52083333333333570, 7.949999999999998401, 2.130196079827431532 ) ) ;
#16986=CARTESIAN_POINT ( 'NONE',  ( 52.93793019189809002, -6.110000000000001208, 1.637169565754158951 ) ) ;
#17026=CARTESIAN_POINT ( 'NONE',  ( 123.3754301918981184, -5.291415217122920289, -3.055000000000001492 ) ) ;
#17031=CYLINDRICAL_SURFACE ( 'NONE', #66721, 6.349999999999999645 ) ;
#17040=CARTESIAN_POINT ( 'NONE',  ( 93.53709685856479439, -3.054999999999998828, -5.291415217122919401 ) ) ;
#17052=CARTESIAN_POINT ( 'NONE',  ( 102.5000000000000142, 0.000000000000000000, -7.950000000000000178 ) ) ;
#17056=DIRECTION ( 'NONE',  ( -1.000000000000000000, -0.000000000000000000, -0.000000000000000000 ) ) ;
#17065=CARTESIAN_POINT ( 'NONE',  ( 44.04209685856477563, 5.291415217122923842, -3.054999999999996163 ) ) ;
#17110=CARTESIAN_POINT ( 'NONE',  ( 94.87086038379621300, 6.884901960086289741, -3.974999999999993427 ) ) ;
#17114=CARTESIAN_POINT ( 'NONE',  ( 73.84959685856480860, 6.109999999999997655, 1.637169565754163836 ) ) ;
#17134=CARTESIAN_POINT ( 'NONE',  ( 120.9750270504628986, -5.819803920172573086, 5.819803920172573086 ) ) ;
#17138=CARTESIAN_POINT ( 'NONE',  ( 89.76669371712954160, -7.949999999999999289, 2.130196079827424427 ) ) ;
#17140=CARTESIAN_POINT ( 'NONE',  ( 71.14583333333332860, 2.130196079827356037, -7.950000000000043698 ) ) ;
#17145=CARTESIAN_POINT ( 'NONE',  ( 0.000000000000000000, 0.000000000000000000, 7.950000000000000178 ) ) ;
#17157=CARTESIAN_POINT ( 'NONE',  ( 84.72959685856476142, -6.110000000000000320, -1.637169565754161393 ) ) ;
#17178=CARTESIAN_POINT ( 'NONE',  ( 74.37543019189810423, -5.291415217122920289, -3.055000000000001492 ) ) ;
#17196=ORIENTED_EDGE ( 'NONE', *, *, #140874, .T. ) ;
#17214=CYLINDRICAL_SURFACE ( 'NONE', #116660, 7.950000000000000178 ) ;
#17217=CARTESIAN_POINT ( 'NONE',  ( 27.00000000000000000, -6.630908077684978252, -3.107243673821709962 ) ) ;
#17228=CARTESIAN_POINT ( 'NONE',  ( 70.29209685856477563, -5.291415217122921177, 3.054999999999999272 ) ) ;
#17234=CARTESIAN_POINT ( 'NONE',  ( 107.7712635252314328, 4.472830434245838482, 4.472830434245842035 ) ) ;
#17250=CARTESIAN_POINT ( 'NONE',  ( 113.6833603837962272, -2.130196079827426203, 7.949999999999996625 ) ) ;
#17265=CARTESIAN_POINT ( 'NONE',  ( 11.47373016279025748, -8.505883529166709422, 4.231315693744567064 ) ) ;
#17279=EDGE_LOOP ( 'NONE', ( #114771, #115357, #61360, #52851 ) ) ;
#17287=CARTESIAN_POINT ( 'NONE',  ( 104.8333333333333286, -6.884901960086287964, 3.974999999999998312 ) ) ;
#17293=CARTESIAN_POINT ( 'NONE',  ( 122.4333603837962130, 2.130196079827431532, -7.949999999999997513 ) ) ;
#17311=CARTESIAN_POINT ( 'NONE',  ( 83.83333333333332860, -6.884901960086287964, 3.974999999999998312 ) ) ;
#17337=CARTESIAN_POINT ( 'NONE',  ( 98.72959685856478984, -6.110000000000000320, -1.637169565754161393 ) ) ;
#17343=CARTESIAN_POINT ( 'NONE',  ( 75.52083333333332860, 7.949999999999998401, 2.130196079827431532 ) ) ;
#17345=CARTESIAN_POINT ( 'NONE',  ( 91.64126352523143737, 4.472830434245836706, 4.472830434245840259 ) ) ;
#17373=CARTESIAN_POINT ( 'NONE',  ( 115.9954301918981230, 5.291415217122916737, 3.055000000000001936 ) ) ;
#17374=DIRECTION ( 'NONE',  ( -1.000000000000000000, -0.000000000000000000, -0.000000000000000000 ) ) ;
#17394=CARTESIAN_POINT ( 'NONE',  ( 32.28709685856477307, 3.054999999999997495, 5.291415217122919401 ) ) ;
#17428=CARTESIAN_POINT ( 'NONE',  ( 101.1204301918981230, 3.055000000000002380, -5.291415217122917625 ) ) ;
#17459=CARTESIAN_POINT ( 'NONE',  ( 20.65000000000000213, 0.000000000000000000, 0.000000000000000000 ) ) ;
#17480=CARTESIAN_POINT ( 'NONE',  ( 111.1041666666666714, 2.130196079827422206, 7.950000000000001954 ) ) ;
#17491=CARTESIAN_POINT ( 'NONE',  ( 106.8962635252314328, 4.472830434245840259, -4.472830434245839371 ) ) ;
#17500=CARTESIAN_POINT ( 'NONE',  ( 40.32919371712954870, -3.975000000000001865, 6.884901960086284411 ) ) ;
#17506=CARTESIAN_POINT ( 'NONE',  ( 127.4587635252314470, 0.000000000000000000, -6.110000000000001208 ) ) ;
#17513=CARTESIAN_POINT ( 'NONE',  ( 27.85459685856477208, -1.637169565754161615, 6.110000000000000320 ) ) ;
#17523=CARTESIAN_POINT ( 'NONE',  ( 57.31293019189811133, -1.637169565754159617, -6.110000000000001208 ) ) ;
#17533=CARTESIAN_POINT ( 'NONE',  ( 45.70376352523145158, 6.109999999999998543, 1.122388791418548911E-15 ) ) ;
#17557=CARTESIAN_POINT ( 'NONE',  ( 53.57876352523144448, -7.482591942790325086E-16, 6.109999999999998543 ) ) ;
#17598=CARTESIAN_POINT ( 'NONE',  ( 108.9166666666666572, -6.884901960086287076, -3.975000000000000977 ) ) ;
#17602=CYLINDRICAL_SURFACE ( 'NONE', #44150, 9.500000000000001776 ) ;
#17627=CARTESIAN_POINT ( 'NONE',  ( 44.53709685856478728, -3.054999999999999272, -5.291415217122919401 ) ) ;
#17652=CARTESIAN_POINT ( 'NONE',  ( 62.93336038379622721, 2.130196079827431532, -7.949999999999997513 ) ) ;
#17657=CARTESIAN_POINT ( 'NONE',  ( 60.06249999999998579, -5.819803920172572198, -5.819803920172573086 ) ) ;
#17667=CARTESIAN_POINT ( 'NONE',  ( 56.72959685856476142, -6.110000000000000320, -1.637169565754161393 ) ) ;
#17713=PRODUCT_CONTEXT ( 'NONE', #80048, 'mechanical' ) ;
#17717=CARTESIAN_POINT ( 'NONE',  ( 95.14126352523143737, 4.472830434245835818, 4.472830434245840259 ) ) ;
#17735=EDGE_CURVE ( 'NONE', #79314, #83079, #128270, .T. ) ;
#17741=CARTESIAN_POINT ( 'NONE',  ( 47.83376352523143993, 6.110000000000001208, 1.122388791418549305E-15 ) ) ;
#17760=CARTESIAN_POINT ( 'NONE',  ( 0.000000000000000000, 0.000000000000000000, 0.000000000000000000 ) ) ;
#17795=CARTESIAN_POINT ( 'NONE',  ( 75.30793019189809456, -6.109999999999999432, 1.637169565754158507 ) ) ;
#17796=( BOUNDED_CURVE ( )  B_SPLINE_CURVE ( 2, ( #124499, #80312, #102762, #12159, #47004, #79631, #35389, #25173, #34645, #67279, #24468, #90447, #23768 ),
 .UNSPECIFIED., .F., .F. ) 
 B_SPLINE_CURVE_WITH_KNOTS ( ( 3, 2, 2, 2, 2, 2, 3 ),
 ( 0.2500000000000000000, 0.2527777777777777679, 0.2555555555555555358, 0.2583333333333333592, 0.2611111111111111271, 0.2638888888888888951, 0.2666666666666666630 ),
 .UNSPECIFIED. ) 
 CURVE ( )  GEOMETRIC_REPRESENTATION_ITEM ( )  RATIONAL_B_SPLINE_CURVE ( ( 1.000000000000000000, 0.9659258262890683122, 1.000000000000000000, 0.9659258262890683122, 1.000000000000000000, 0.9659258262890683122, 1.000000000000000000, 0.9659258262890683122, 1.000000000000000000, 0.9659258262890683122, 1.000000000000000000, 0.9659258262890683122, 1.000000000000000000 ) ) 
 REPRESENTATION_ITEM ( '' )  );
#17808=( BOUNDED_CURVE ( )  B_SPLINE_CURVE ( 2, ( #140885, #87244, #32147, #119142, #44488, #64066, #66924, #19825, #41583, #108965, #108232, #53167, #87953 ),
 .UNSPECIFIED., .F., .F. ) 
 B_SPLINE_CURVE_WITH_KNOTS ( ( 3, 2, 2, 2, 2, 2, 3 ),
 ( 0.4500000000000000111, 0.4527777777777777790, 0.4555555555555555469, 0.4583333333333333148, 0.4611111111111111382, 0.4638888888888889062, 0.4666666666666666741 ),
 .UNSPECIFIED. ) 
 CURVE ( )  GEOMETRIC_REPRESENTATION_ITEM ( )  RATIONAL_B_SPLINE_CURVE ( ( 1.000000000000000000, 0.9659258262890683122, 1.000000000000000000, 0.9659258262890683122, 1.000000000000000000, 0.9659258262890683122, 1.000000000000000000, 0.9659258262890683122, 1.000000000000000000, 0.9659258262890683122, 1.000000000000000000, 0.9659258262890683122, 1.000000000000000000 ) ) 
 REPRESENTATION_ITEM ( '' )  );
#17820=CARTESIAN_POINT ( 'NONE',  ( 93.99586038379622721, -3.974999999999998312, -6.884901960086286188 ) ) ;
#17831=ADVANCED_FACE ( 'NONE', ( #104930 ), #17214, .T. ) ;
#17833=CARTESIAN_POINT ( 'NONE',  ( 86.33376352523144703, 6.110000000000001208, 1.122388791418549305E-15 ) ) ;
#17854=CARTESIAN_POINT ( 'NONE',  ( 76.56293019189810423, 1.637169565754157174, 6.110000000000002984 ) ) ;
#17891=CARTESIAN_POINT ( 'NONE',  ( 27.00000000000001066, -7.055460226182286299, -2.590656038797956029 ) ) ;
#17901=CARTESIAN_POINT ( 'NONE',  ( 76.85459685856477563, -1.637169565754161615, 6.110000000000000320 ) ) ;
#17908=CARTESIAN_POINT ( 'NONE',  ( 109.2295968585647614, -6.110000000000000320, -1.637169565754161393 ) ) ;
#17943=CARTESIAN_POINT ( 'NONE',  ( 12.99975870850580861, -8.843799839164724119, 3.473668526774862819 ) ) ;
#17945=ORIENTED_EDGE ( 'NONE', *, *, #130159, .F. ) ;
#17961=ORIENTED_EDGE ( 'NONE', *, *, #65610, .F. ) ;
#17965=ORIENTED_EDGE ( 'NONE', *, *, #120106, .F. ) ;
#17973=CARTESIAN_POINT ( 'NONE',  ( 120.8291937171295700, -3.975000000000001865, 6.884901960086284411 ) ) ;
#17988=CARTESIAN_POINT ( 'NONE',  ( 86.75000000000000000, -9.735942053221458872E-16, 7.950000000000000178 ) ) ;
#17990=EDGE_LOOP ( 'NONE', ( #136684, #104395, #142497, #52816 ) ) ;
#18012=CARTESIAN_POINT ( 'NONE',  ( 98.00043019189810423, -3.055000000000002380, 5.291415217122920289 ) ) ;
#18019=CARTESIAN_POINT ( 'NONE',  ( 75.08333333333332860, 6.884901960086290629, -3.974999999999994316 ) ) ;
#18022=CARTESIAN_POINT ( 'NONE',  ( 95.14126352523143737, 4.472830434245836706, 4.472830434245840259 ) ) ;
#18030=LINE ( 'NONE', #62311, #90185 ) ;
#18071=CARTESIAN_POINT ( 'NONE',  ( 26.45376352523144803, -6.109999999999998543, -3.741295971395162543E-16 ) ) ;
#18108=CARTESIAN_POINT ( 'NONE',  ( 93.82876352523145158, 0.000000000000000000, -6.109999999999999432 ) ) ;
#18135=ORIENTED_EDGE ( 'NONE', *, *, #67174, .T. ) ;
#18148=EDGE_CURVE ( 'NONE', #9583, #133905, #77349, .T. ) ;
#18159=CARTESIAN_POINT ( 'NONE',  ( 108.3333333333333428, -6.884901960086287964, 3.974999999999998312 ) ) ;
#18174=CARTESIAN_POINT ( 'NONE',  ( 99.45876352523144703, 0.000000000000000000, -6.110000000000001208 ) ) ;
#18179=CARTESIAN_POINT ( 'NONE',  ( 83.05836038379621300, -7.949999999999996625, -2.130196079827426203 ) ) ;
#18184=CARTESIAN_POINT ( 'NONE',  ( 40.91252705046288440, -7.949999999999998401, -4.867971026610728450E-16 ) ) ;
#18189=CARTESIAN_POINT ( 'NONE',  ( 125.5629301918981042, 1.637169565754157174, 6.110000000000002984 ) ) ;
#18200=CARTESIAN_POINT ( 'NONE',  ( 122.5579301918981088, 6.110000000000000320, -1.637169565754156064 ) ) ;
#18211=CARTESIAN_POINT ( 'NONE',  ( 49.87543019189810423, -5.291415217122920289, -3.055000000000001492 ) ) ;
#18219=CARTESIAN_POINT ( 'NONE',  ( 47.30793019189811588, -6.109999999999998543, 1.637169565754158063 ) ) ;
#18230=CARTESIAN_POINT ( 'NONE',  ( 44.55836038379621300, -7.949999999999996625, -2.130196079827426203 ) ) ;
#18246=DIRECTION ( 'NONE',  ( 0.000000000000000000, 0.000000000000000000, 1.000000000000000000 ) ) ;
#18249=CARTESIAN_POINT ( 'NONE',  ( 57.37043019189810877, -3.055000000000001492, 5.291415217122917625 ) ) ;
#18267=VECTOR ( 'NONE', #82276, 1000.000000000000000 ) ;
#18287=CARTESIAN_POINT ( 'NONE',  ( 127.6620968585647802, -5.291415217122919401, 3.054999999999998384 ) ) ;
#18296=CARTESIAN_POINT ( 'NONE',  ( 75.76669371712954160, -7.949999999999998401, 2.130196079827423983 ) ) ;
#18298=CARTESIAN_POINT ( 'NONE',  ( 108.0416666666666714, -3.975000000000002753, 6.884901960086286188 ) ) ;
#18311=ORIENTED_EDGE ( 'NONE', *, *, #74417, .T. ) ;
#18324=CARTESIAN_POINT ( 'NONE',  ( 36.95376352523144448, -6.109999999999999432, -3.741295971395163529E-16 ) ) ;
#18331=ORIENTED_EDGE ( 'NONE', *, *, #74463, .T. ) ;
#18340=CARTESIAN_POINT ( 'NONE',  ( 81.93750000000000000, 5.819803920172574863, -5.819803920172573086 ) ) ;
#18351=CARTESIAN_POINT ( 'NONE',  ( 70.22502705046287019, 5.819803920172573086, -5.819803920172572198 ) ) ;
#18356=CARTESIAN_POINT ( 'NONE',  ( 53.06250000000000000, -5.819803920172572198, -5.819803920172573086 ) ) ;
#18363=CARTESIAN_POINT ( 'NONE',  ( 33.81249999999999289, 5.819803920172571310, 5.819803920172576639 ) ) ;
#18365=CARTESIAN_POINT ( 'NONE',  ( 44.91709685856476142, 3.054999999999998828, 5.291415217122922066 ) ) ;
#18371=ORIENTED_EDGE ( 'NONE', *, *, #99965, .T. ) ;
#18381=CARTESIAN_POINT ( 'NONE',  ( 100.1208603837962272, -6.884901960086286188, 3.974999999999997424 ) ) ;
#18394=CARTESIAN_POINT ( 'NONE',  ( 81.14126352523143737, 4.472830434245836706, 4.472830434245840259 ) ) ;
#18420=CARTESIAN_POINT ( 'NONE',  ( 84.49543019189812298, 5.291415217122916737, 3.055000000000001936 ) ) ;
#18443=EDGE_CURVE ( 'NONE', #113567, #942, #134204, .T. ) ;
#18446=CARTESIAN_POINT ( 'NONE',  ( 32.66709685856476852, -3.055000000000000160, -5.291415217122921177 ) ) ;
#18455=VERTEX_POINT ( 'NONE', #47931 ) ;
#18504=CARTESIAN_POINT ( 'NONE',  ( 76.62043019189812298, 3.055000000000002380, -5.291415217122917625 ) ) ;
#18527=CARTESIAN_POINT ( 'NONE',  ( 94.43336038379622721, 2.130196079827431532, -7.949999999999997513 ) ) ;
#18537=CARTESIAN_POINT ( 'NONE',  ( 46.74586038379622011, 3.974999999999996980, 6.884901960086287964 ) ) ;
#18540=CARTESIAN_POINT ( 'NONE',  ( 84.29209685856477563, -5.291415217122921177, 3.054999999999999272 ) ) ;
#18563=CARTESIAN_POINT ( 'NONE',  ( 69.41709685856477563, 3.054999999999998828, 5.291415217122922066 ) ) ;
#18577=AXIS2_PLACEMENT_3D ( 'NONE', #83574, #94414, #138662 ) ;
#18618=CARTESIAN_POINT ( 'NONE',  ( 50.58333333333332860, 6.884901960086290629, -3.974999999999994316 ) ) ;
#18625=CARTESIAN_POINT ( 'NONE',  ( 67.37543019189810423, -5.291415217122920289, -3.055000000000001492 ) ) ;
#18631=CARTESIAN_POINT ( 'NONE',  ( 112.4379301918981184, -6.110000000000001208, 1.637169565754158951 ) ) ;
#18638=( BOUNDED_CURVE ( )  B_SPLINE_CURVE ( 2, ( #73739, #63616, #42578, #95483, #30233, #74485, #130999, #20780, #18618, #65033, #139746, #40424, #86056 ),
 .UNSPECIFIED., .F., .F. ) 
 B_SPLINE_CURVE_WITH_KNOTS ( ( 3, 2, 2, 2, 2, 2, 3 ),
 ( 0.7166666666666667851, 0.7194444444444445530, 0.7222222222222223209, 0.7250000000000000888, 0.7277777777777778567, 0.7305555555555556246, 0.7333333333333333925 ),
 .UNSPECIFIED. ) 
 CURVE ( )  GEOMETRIC_REPRESENTATION_ITEM ( )  RATIONAL_B_SPLINE_CURVE ( ( 0.9999999999999986677, 0.9659258262890696445, 1.000000000000000000, 0.9659258262890683122, 1.000000000000000000, 0.9659258262890683122, 1.000000000000000000, 0.9659258262890683122, 1.000000000000000000, 0.9659258262890683122, 1.000000000000000000, 0.9659258262890669799, 1.000000000000001332 ) ) 
 REPRESENTATION_ITEM ( '' )  );
#18641=CARTESIAN_POINT ( 'NONE',  ( 77.95419371712955581, 6.884901960086283523, 3.975000000000002753 ) ) ;
#18664=CARTESIAN_POINT ( 'NONE',  ( 90.49586038379622721, -3.974999999999998312, -6.884901960086286188 ) ) ;
#18667=CARTESIAN_POINT ( 'NONE',  ( 38.18749999999999289, -5.819803920172573974, 5.819803920172573086 ) ) ;
#18681=PLANE ( 'NONE',  #6671 ) ;
#18682=CARTESIAN_POINT ( 'NONE',  ( 28.14626352523143638, -4.472830434245840259, 4.472830434245839371 ) ) ;
#18699=CARTESIAN_POINT ( 'NONE',  ( 94.14169371712955581, -2.130196079827424871, -7.949999999999998401 ) ) ;
#18700=CARTESIAN_POINT ( 'NONE',  ( 124.3291937171295700, -3.975000000000001865, 6.884901960086284411 ) ) ;
#18704=FACE_OUTER_BOUND ( 'NONE', #10307, .T. ) ;
#18715=CARTESIAN_POINT ( 'NONE',  ( 85.29166666666667140, 3.975000000000003642, -6.884901960086285300 ) ) ;
#18725=CARTESIAN_POINT ( 'NONE',  ( 29.97502705046288440, -5.819803920172573086, 5.819803920172573086 ) ) ;
#18735=CARTESIAN_POINT ( 'NONE',  ( 40.66666666666665719, 6.884901960086285300, 3.975000000000003642 ) ) ;
#18746=CARTESIAN_POINT ( 'NONE',  ( 97.70876352523144703, -7.482591942790329030E-16, 6.110000000000001208 ) ) ;
#18758=CARTESIAN_POINT ( 'NONE',  ( 97.91209685856478018, 5.291415217122921177, -3.054999999999994831 ) ) ;
#18846=( BOUNDED_CURVE ( )  B_SPLINE_CURVE ( 2, ( #136212, #28177, #36208, #94122, #36896, #72439, #81145, #116607, #17287, #3526, #2840, #92700, #47135 ),
 .UNSPECIFIED., .F., .T. ) 
 B_SPLINE_CURVE_WITH_KNOTS ( ( 3, 2, 2, 2, 2, 2, 3 ),
 ( 0.2000000000000000389, 0.2027777777777778068, 0.2055555555555555747, 0.2083333333333333703, 0.2111111111111111660, 0.2138888888888889339, 0.2166666666666667296 ),
 .UNSPECIFIED. ) 
 CURVE ( )  GEOMETRIC_REPRESENTATION_ITEM ( )  RATIONAL_B_SPLINE_CURVE ( ( 0.9999999999999996669, 0.9659258262890686453, 1.000000000000000000, 0.9659258262890683122, 1.000000000000000000, 0.9659258262890683122, 1.000000000000000000, 0.9659258262890683122, 1.000000000000000000, 0.9659258262890683122, 1.000000000000000000, 0.9659258262890676461, 1.000000000000000666 ) ) 
 REPRESENTATION_ITEM ( '' )  );
#18851=CARTESIAN_POINT ( 'NONE',  ( 87.99543019189812298, 5.291415217122917625, 3.055000000000002380 ) ) ;
#18853=DIRECTION ( 'NONE',  ( -1.000000000000000000, -0.000000000000000000, -0.000000000000000000 ) ) ;
#18881=DIRECTION ( 'NONE',  ( -1.000000000000000000, -0.000000000000000000, -0.000000000000000000 ) ) ;
#18894=CARTESIAN_POINT ( 'NONE',  ( 31.77083333333333215, -7.949999999999998401, -2.130196079827426203 ) ) ;
#18907=CARTESIAN_POINT ( 'NONE',  ( 106.4374999999999858, 5.819803920172573974, -5.819803920172572198 ) ) ;
#18922=CARTESIAN_POINT ( 'NONE',  ( 107.9170968585647756, 3.054999999999998828, 5.291415217122922066 ) ) ;
#18932=CARTESIAN_POINT ( 'NONE',  ( 30.12086038379621655, -6.884901960086286188, 3.974999999999997424 ) ) ;
#18938=CARTESIAN_POINT ( 'NONE',  ( 29.87500000000000000, 7.950000000000000178, 1.460391307983218535E-15 ) ) ;
#18952=CARTESIAN_POINT ( 'NONE',  ( 124.7454301918981230, -5.291415217122918513, -3.055000000000000160 ) ) ;
#18963=CARTESIAN_POINT ( 'NONE',  ( 50.02126352523143282, -4.472830434245839371, -4.472830434245840259 ) ) ;
#18971=CARTESIAN_POINT ( 'NONE',  ( 43.22459685856478728, -1.637169565754160949, 6.109999999999997655 ) ) ;
#18981=CARTESIAN_POINT ( 'NONE',  ( 80.14169371712957002, -2.130196079827424871, -7.949999999999998401 ) ) ;
#18989=LINE ( 'NONE', #140078, #58186 ) ;
#19000=ADVANCED_FACE ( 'NONE', ( #70245 ), #15077, .T. ) ;
#19002=CARTESIAN_POINT ( 'NONE',  ( 58.82876352523144448, 0.000000000000000000, -6.109999999999998543 ) ) ;
#19036=CARTESIAN_POINT ( 'NONE',  ( 117.5995968585647944, -6.109999999999998543, -1.637169565754160727 ) ) ;
#19077=CARTESIAN_POINT ( 'NONE',  ( 35.20376352523143737, 6.109999999999999432, 1.122388791418549108E-15 ) ) ;
#19100=CARTESIAN_POINT ( 'NONE',  ( 104.7875270504628986, 0.000000000000000000, -7.949999999999998401 ) ) ;
#19101=CARTESIAN_POINT ( 'NONE',  ( 54.03752705046288440, -9.735942053221456900E-16, 7.949999999999998401 ) ) ;
#19107=CARTESIAN_POINT ( 'NONE',  ( 51.60416666666665009, 2.130196079827422206, 7.950000000000001954 ) ) ;
#19117=CARTESIAN_POINT ( 'NONE',  ( 49.43793019189809002, -6.110000000000001208, 1.637169565754158951 ) ) ;
#19120=CARTESIAN_POINT ( 'NONE',  ( 37.74999999999999289, -9.735942053221458872E-16, 7.950000000000000178 ) ) ;
#19121=VERTEX_POINT ( 'NONE', #15751 ) ;
#19143=CARTESIAN_POINT ( 'NONE',  ( 69.03709685856478018, -3.054999999999998828, -5.291415217122919401 ) ) ;
#19175=CARTESIAN_POINT ( 'NONE',  ( 86.97459685856479439, 1.637169565754164280, -6.109999999999996767 ) ) ;
#19196=CARTESIAN_POINT ( 'NONE',  ( 122.5791937171295700, 3.975000000000002753, -6.884901960086283523 ) ) ;
#19202=CARTESIAN_POINT ( 'NONE',  ( 38.93793019189809002, -6.110000000000001208, 1.637169565754158951 ) ) ;
#19221=CARTESIAN_POINT ( 'NONE',  ( 109.6000270504628844, 5.819803920172570422, 5.819803920172575751 ) ) ;
#19254=CARTESIAN_POINT ( 'NONE',  ( 64.80793019189812298, -6.109999999999999432, 1.637169565754158507 ) ) ;
#19279=CARTESIAN_POINT ( 'NONE',  ( 92.24586038379622721, 3.974999999999996980, 6.884901960086287964 ) ) ;
#19294=CARTESIAN_POINT ( 'NONE',  ( 78.02126352523146124, -4.472830434245839371, -4.472830434245840259 ) ) ;
#19314=CARTESIAN_POINT ( 'NONE',  ( 77.58376352523144703, -6.110000000000001208, -3.741295971395164515E-16 ) ) ;
#19338=CARTESIAN_POINT ( 'NONE',  ( 127.4302689125804733, -3.175000000000002043, 5.499261314031184789 ) ) ;
#19370=CARTESIAN_POINT ( 'NONE',  ( 63.00043019189810423, -3.055000000000002380, 5.291415217122920289 ) ) ;
#19376=CARTESIAN_POINT ( 'NONE',  ( 100.9170968585647756, 3.054999999999998828, 5.291415217122922066 ) ) ;
#19383=CARTESIAN_POINT ( 'NONE',  ( 90.83333333333332860, -6.884901960086287964, 3.974999999999998312 ) ) ;
#19418=CARTESIAN_POINT ( 'NONE',  ( 30.77126352523143638, 4.472830434245839371, 4.472830434245842035 ) ) ;
#19424=DIRECTION ( 'NONE',  ( -1.000000000000000000, -0.000000000000000000, -0.000000000000000000 ) ) ;
#19440=CARTESIAN_POINT ( 'NONE',  ( 118.9333603837962414, 2.130196079827431532, -7.949999999999997513 ) ) ;
#19466=CARTESIAN_POINT ( 'NONE',  ( 92.29166666666665719, 3.975000000000003642, -6.884901960086285300 ) ) ;
#19473=CARTESIAN_POINT ( 'NONE',  ( 41.24999999999999289, -9.735942053221458872E-16, 7.950000000000000178 ) ) ;
#19480=CARTESIAN_POINT ( 'NONE',  ( 104.8545968585647756, -1.637169565754161615, 6.110000000000000320 ) ) ;
#19487=CARTESIAN_POINT ( 'NONE',  ( 74.93749999999998579, 5.819803920172574863, -5.819803920172573086 ) ) ;
#19490=CARTESIAN_POINT ( 'NONE',  ( 91.93293019189812298, 1.637169565754156508, 6.110000000000000320 ) ) ;
#19520=CARTESIAN_POINT ( 'NONE',  ( 55.83333333333332860, -6.884901960086287964, 3.974999999999998312 ) ) ;
#19539=CARTESIAN_POINT ( 'NONE',  ( 31.84959685856478373, 6.109999999999996767, 1.637169565754163836 ) ) ;
#19573=CARTESIAN_POINT ( 'NONE',  ( 93.24543019189812298, -5.291415217122919401, -3.055000000000000604 ) ) ;
#19625=CARTESIAN_POINT ( 'NONE',  ( 111.2500000000000000, -9.735942053221458872E-16, 7.950000000000000178 ) ) ;
#19639=CARTESIAN_POINT ( 'NONE',  ( 107.6254301918981042, 5.291415217122919401, 3.055000000000002824 ) ) ;
#19653=CARTESIAN_POINT ( 'NONE',  ( 28.27083333333333215, -7.949999999999999289, -2.130196079827426203 ) ) ;
#19663=CARTESIAN_POINT ( 'NONE',  ( 127.5162635252314516, -4.472830434245839371, 4.472830434245839371 ) ) ;
#19664=ORIENTED_EDGE ( 'NONE', *, *, #120721, .F. ) ;
#19667=CARTESIAN_POINT ( 'NONE',  ( 70.95419371712955581, 6.884901960086283523, 3.975000000000002753 ) ) ;
#19672=CARTESIAN_POINT ( 'NONE',  ( 44.47959685856476852, 6.109999999999999432, 1.637169565754164280 ) ) ;
#19673=ORIENTED_EDGE ( 'NONE', *, *, #83909, .F. ) ;
#19679=CARTESIAN_POINT ( 'NONE',  ( 37.09959685856476597, -6.109999999999997655, -1.637169565754160283 ) ) ;
#19707=CARTESIAN_POINT ( 'NONE',  ( 61.30793019189810877, -6.109999999999998543, 1.637169565754158507 ) ) ;
#19745=CARTESIAN_POINT ( 'NONE',  ( 121.8287635252314516, 0.000000000000000000, -6.109999999999999432 ) ) ;
#19781=CARTESIAN_POINT ( 'NONE',  ( 126.7258888818563776, -5.807073093359954363, -3.403349999535261627 ) ) ;
#19782=CARTESIAN_POINT ( 'NONE',  ( 37.24543019189811588, -5.291415217122919401, -3.055000000000000604 ) ) ;
#19806=CARTESIAN_POINT ( 'NONE',  ( 52.43336038379623432, 2.130196079827431532, -7.949999999999997513 ) ) ;
#19811=CARTESIAN_POINT ( 'NONE',  ( 50.43750000000000000, 5.819803920172573974, -5.819803920172572198 ) ) ;
#19813=AXIS2_PLACEMENT_3D ( 'NONE', #30926, #86000, #130238 ) ;
#19819=CARTESIAN_POINT ( 'NONE',  ( 43.75043019189810423, 3.055000000000002824, -5.291415217122919401 ) ) ;
#19825=CARTESIAN_POINT ( 'NONE',  ( 81.01669371712955581, 7.950000000000000178, -2.130196079827421318 ) ) ;
#19826=DIRECTION ( 'NONE',  ( -1.000000000000000000, -0.000000000000000000, -0.000000000000000000 ) ) ;
#19833=CARTESIAN_POINT ( 'NONE',  ( 85.89626352523144703, 4.472830434245840259, -4.472830434245838482 ) ) ;
#19845=CARTESIAN_POINT ( 'NONE',  ( 70.78709685856478018, 3.054999999999997495, 5.291415217122919401 ) ) ;
#19866=CARTESIAN_POINT ( 'NONE',  ( 40.62086038379622721, -6.884901960086286188, 3.974999999999997424 ) ) ;
#19872=ORIENTED_EDGE ( 'NONE', *, *, #84150, .T. ) ;
#19873=CARTESIAN_POINT ( 'NONE',  ( 83.47459685856478018, 1.637169565754164280, -6.109999999999996767 ) ) ;
#19894=CARTESIAN_POINT ( 'NONE',  ( 34.12543019189810423, 5.291415217122919401, 3.055000000000002824 ) ) ;
#19906=ORIENTED_EDGE ( 'NONE', *, *, #65832, .T. ) ;
#19946=CARTESIAN_POINT ( 'NONE',  ( 27.00000000000000355, 0.000000000000000000, 6.349999999999999645 ) ) ;
#19952=CARTESIAN_POINT ( 'NONE',  ( 62.91209685856477307, 5.291415217122922066, -3.054999999999995275 ) ) ;
#19974=CARTESIAN_POINT ( 'NONE',  ( 80.43336038379622721, 2.130196079827431532, -7.949999999999997513 ) ) ;
#19987=CARTESIAN_POINT ( 'NONE',  ( 80.06293019189810423, 1.637169565754157174, 6.110000000000002984 ) ) ;
#20006=CARTESIAN_POINT ( 'NONE',  ( 60.81293019189811133, -1.637169565754159617, -6.110000000000001208 ) ) ;
#20028=CARTESIAN_POINT ( 'NONE',  ( 127.8677689125804733, -6.349999999999999645, 1.701477371937628158 ) ) ;
#20039=CARTESIAN_POINT ( 'NONE',  ( 111.3287635252314516, 0.000000000000000000, -6.109999999999998543 ) ) ;
#20061=CARTESIAN_POINT ( 'NONE',  ( 66.35459685856476142, -1.637169565754161615, 6.110000000000000320 ) ) ;
#20067=CARTESIAN_POINT ( 'NONE',  ( 102.6670968585647756, -3.055000000000000160, -5.291415217122921177 ) ) ;
#20085=CARTESIAN_POINT ( 'NONE',  ( 117.7454301918981230, -5.291415217122918513, -3.055000000000000160 ) ) ;
#20101=CARTESIAN_POINT ( 'NONE',  ( 39.35416666666666430, -2.130196079827501698, -7.949999999999956657 ) ) ;
#20112=CARTESIAN_POINT ( 'NONE',  ( 26.68793019189810067, 6.110000000000002984, -1.637169565754156730 ) ) ;
#20137=CARTESIAN_POINT ( 'NONE',  ( 109.0166937171295416, 7.950000000000001066, -2.130196079827421318 ) ) ;
#20153=CARTESIAN_POINT ( 'NONE',  ( 0.000000000000000000, 9.735942053221458872E-16, -7.950000000000000178 ) ) ;
#20170=CARTESIAN_POINT ( 'NONE',  ( 100.1879301918980900, 6.110000000000002984, -1.637169565754156730 ) ) ;
#20179=CARTESIAN_POINT ( 'NONE',  ( 95.57876352523145158, -7.482591942790325086E-16, 6.109999999999998543 ) ) ;
#20182=CARTESIAN_POINT ( 'NONE',  ( 72.75000000000000000, -9.735942053221458872E-16, 7.950000000000000178 ) ) ;
#20209=CARTESIAN_POINT ( 'NONE',  ( 56.85416666666666430, -2.130196079827425759, -7.950000000000000178 ) ) ;
#20233=CARTESIAN_POINT ( 'NONE',  ( 29.66209685856477307, -5.291415217122919401, 3.054999999999997939 ) ) ;
#20237=CARTESIAN_POINT ( 'NONE',  ( 127.0212635252314328, -4.472830434245838482, -4.472830434245840259 ) ) ;
#20271=CARTESIAN_POINT ( 'NONE',  ( 95.14126352523143737, 4.472830434245837594, 4.472830434245841147 ) ) ;
#20273=CARTESIAN_POINT ( 'NONE',  ( 8.129312396003866681, -8.710846131291567929, 3.794790648306943126 ) ) ;
#20297=CARTESIAN_POINT ( 'NONE',  ( 0.000000000000000000, 0.000000000000000000, 7.950000000000000178 ) ) ;
#20306=CARTESIAN_POINT ( 'NONE',  ( 32.49999999999998579, 0.000000000000000000, -7.950000000000000178 ) ) ;
#20319=CARTESIAN_POINT ( 'NONE',  ( 99.58333333333332860, 6.884901960086290629, -3.974999999999994316 ) ) ;
#20333=CARTESIAN_POINT ( 'NONE',  ( 104.8545968585647756, -1.637169565754161615, 6.110000000000000320 ) ) ;
#20342=CARTESIAN_POINT ( 'NONE',  ( 30.85002705046288085, -5.819803920172572198, -5.819803920172572198 ) ) ;
#20346=CARTESIAN_POINT ( 'NONE',  ( 30.60416666666665719, 2.130196079827422206, 7.950000000000001954 ) ) ;
#20355=CARTESIAN_POINT ( 'NONE',  ( 119.9329301918981230, 1.637169565754156508, 6.110000000000000320 ) ) ;
#20360=( NAMED_UNIT ( * ) PLANE_ANGLE_UNIT ( ) SI_UNIT ( $, .RADIAN. ) );
#20366=CARTESIAN_POINT ( 'NONE',  ( 45.64626352523142572, -4.472830434245840259, 4.472830434245839371 ) ) ;
#20376=CARTESIAN_POINT ( 'NONE',  ( 39.14126352523145869, 4.472830434245836706, 4.472830434245840259 ) ) ;
#20404=CARTESIAN_POINT ( 'NONE',  ( 53.87043019189811588, -3.055000000000001492, 5.291415217122917625 ) ) ;
#20413=DIRECTION ( 'NONE',  ( 0.000000000000000000, 0.000000000000000000, 1.000000000000000000 ) ) ;
#20443=CARTESIAN_POINT ( 'NONE',  ( 120.0787635252314516, -7.482591942790327058E-16, 6.109999999999999432 ) ) ;
#20471=DIRECTION ( 'NONE',  ( -1.000000000000000000, -0.000000000000000000, -0.000000000000000000 ) ) ;
#20481=CARTESIAN_POINT ( 'NONE',  ( 33.89126352523143737, -4.472830434245839371, -4.472830434245839371 ) ) ;
#20495=CARTESIAN_POINT ( 'NONE',  ( 127.3129301918980900, -1.637169565754159617, -6.110000000000001208 ) ) ;
#20504=CARTESIAN_POINT ( 'NONE',  ( 60.45419371712955581, 6.884901960086283523, 3.975000000000002753 ) ) ;
#20508=CARTESIAN_POINT ( 'NONE',  ( 56.99999999999999289, 0.000000000000000000, -7.950000000000000178 ) ) ;
#20516=CARTESIAN_POINT ( 'NONE',  ( 50.89626352523143993, 4.472830434245840259, -4.472830434245839371 ) ) ;
#20536=CARTESIAN_POINT ( 'NONE',  ( 84.58376352523144703, -6.110000000000001208, -3.741295971395164515E-16 ) ) ;
#20547=CARTESIAN_POINT ( 'NONE',  ( 70.64126352523145158, 4.472830434245836706, 4.472830434245840259 ) ) ;
#20563=VERTEX_POINT ( 'NONE', #96747 ) ;
#20584=CARTESIAN_POINT ( 'NONE',  ( 86.68293019189812298, -1.637169565754158951, -6.109999999999998543 ) ) ;
#20609=CARTESIAN_POINT ( 'NONE',  ( 38.79209685856477563, -5.291415217122921177, 3.054999999999999272 ) ) ;
#20610=VERTEX_POINT ( 'NONE', #97487 ) ;
#20611=CARTESIAN_POINT ( 'NONE',  ( 46.06249999999999289, -5.819803920172573086, -5.819803920172573974 ) ) ;
#20647=VERTEX_POINT ( 'NONE', #135167 ) ;
#20663=CARTESIAN_POINT ( 'NONE',  ( 65.09959685856478018, -6.109999999999998543, -1.637169565754160727 ) ) ;
#20695=CARTESIAN_POINT ( 'NONE',  ( 87.87086038379622721, 6.884901960086289741, -3.974999999999993427 ) ) ;
#20706=CARTESIAN_POINT ( 'NONE',  ( 72.18793019189810423, 6.110000000000002984, -1.637169565754156730 ) ) ;
#20726=CARTESIAN_POINT ( 'NONE',  ( 61.68793019189811844, 6.110000000000002984, -1.637169565754156730 ) ) ;
#20753=CIRCLE ( 'NONE', #50897, 6.349999999999997868 ) ;
#20760=CARTESIAN_POINT ( 'NONE',  ( 108.5579301918981088, 6.110000000000000320, -1.637169565754156064 ) ) ;
#20780=CARTESIAN_POINT ( 'NONE',  ( 50.72916666666665719, 7.950000000000001954, -2.130196079827421762 ) ) ;
#20786=CARTESIAN_POINT ( 'NONE',  ( 59.20876352523143993, -7.482591942790329030E-16, 6.110000000000001208 ) ) ;
#20792=CARTESIAN_POINT ( 'NONE',  ( 99.31293019189810423, -1.637169565754159617, -6.110000000000001208 ) ) ;
#20808=CARTESIAN_POINT ( 'NONE',  ( 121.3912635252314374, -4.472830434245838482, -4.472830434245838482 ) ) ;
#20820=CARTESIAN_POINT ( 'NONE',  ( 11.04893972570927296, -8.462477794511665152, -4.317117199209826062 ) ) ;
#20824=DIRECTION ( 'NONE',  ( 0.000000000000000000, 0.000000000000000000, 1.000000000000000000 ) ) ;
#20832=CARTESIAN_POINT ( 'NONE',  ( 33.68793019189809712, 6.110000000000002984, -1.637169565754156730 ) ) ;
#20835=VERTEX_POINT ( 'NONE', #39407 ) ;
#20855=CARTESIAN_POINT ( 'NONE',  ( 117.1833603837962272, -2.130196079827426203, 7.949999999999997513 ) ) ;
#20856=CARTESIAN_POINT ( 'NONE',  ( 49.37086038379622011, 6.884901960086289741, -3.974999999999993427 ) ) ;
#20882=CARTESIAN_POINT ( 'NONE',  ( 0.000000000000000000, 0.000000000000000000, 0.000000000000000000 ) ) ;
#20886=CARTESIAN_POINT ( 'NONE',  ( 69.54166666666667140, -3.975000000000002753, 6.884901960086286188 ) ) ;
#20893=CARTESIAN_POINT ( 'NONE',  ( 93.77126352523141861, 4.472830434245839371, 4.472830434245842035 ) ) ;
#20896=ADVANCED_FACE ( 'NONE', ( #103205 ), #15450, .T. ) ;
#20904=CARTESIAN_POINT ( 'NONE',  ( 82.74543019189812298, -5.291415217122918513, -3.055000000000000160 ) ) ;
#20907=CARTESIAN_POINT ( 'NONE',  ( 114.8958333333333428, -2.130196079827447075, 7.949999999999988631 ) ) ;
#20918=AXIS2_PLACEMENT_3D ( 'NONE', #122862, #112695, #23549 ) ;
#20924=( BOUNDED_CURVE ( )  B_SPLINE_CURVE ( 2, ( #19473, #128945, #107187, #131098, #18735, #52101, #107876, #118776, #41217, #85422, #52790, #96989, #108579 ),
 .UNSPECIFIED., .F., .T. ) 
 B_SPLINE_CURVE_WITH_KNOTS ( ( 3, 2, 2, 2, 2, 2, 3 ),
 ( 0.8166666666666666519, 0.8194444444444444198, 0.8222222222222221877, 0.8249999999999999556, 0.8277777777777778345, 0.8305555555555557135, 0.8333333333333334814 ),
 .UNSPECIFIED. ) 
 CURVE ( )  GEOMETRIC_REPRESENTATION_ITEM ( )  RATIONAL_B_SPLINE_CURVE ( ( 1.000000000000000000, 0.9659258262890683122, 1.000000000000000000, 0.9659258262890683122, 1.000000000000000000, 0.9659258262890683122, 1.000000000000000000, 0.9659258262890683122, 1.000000000000000000, 0.9659258262890683122, 1.000000000000000000, 0.9659258262890669799, 1.000000000000001332 ) ) 
 REPRESENTATION_ITEM ( '' )  );
#20940=AXIS2_PLACEMENT_3D ( 'NONE', #42645, #75267, #96946 ) ;
#20942=CARTESIAN_POINT ( 'NONE',  ( 119.2708333333333286, -7.949999999999998401, -2.130196079827426203 ) ) ;
#20960=CARTESIAN_POINT ( 'NONE',  ( 124.5420968585647756, 5.291415217122923842, -3.054999999999996163 ) ) ;
#20993=CARTESIAN_POINT ( 'NONE',  ( 94.84959685856476597, 6.109999999999997655, 1.637169565754163836 ) ) ;
#20994=CARTESIAN_POINT ( 'NONE',  ( 6.613632711652026153, -9.212947288752639352, -2.320845120914358795 ) ) ;
#20998=FACE_OUTER_BOUND ( 'NONE', #66717, .T. ) ;
#21042=CARTESIAN_POINT ( 'NONE',  ( 105.7083333333333286, -3.974999999999999201, -6.884901960086287964 ) ) ;
#21065=CARTESIAN_POINT ( 'NONE',  ( 30.70419371712955581, -6.884901960086285300, -3.975000000000000089 ) ) ;
#21071=CARTESIAN_POINT ( 'NONE',  ( 122.9379301918981042, -6.110000000000001208, 1.637169565754158951 ) ) ;
#21086=CARTESIAN_POINT ( 'NONE',  ( 125.1829301918981372, -1.637169565754158951, -6.109999999999998543 ) ) ;
#21094=CARTESIAN_POINT ( 'NONE',  ( 43.02126352523142572, -4.472830434245839371, -4.472830434245840259 ) ) ;
#21104=CARTESIAN_POINT ( 'NONE',  ( 38.26626352523144448, 4.472830434245839371, -4.472830434245838482 ) ) ;
#21137=CARTESIAN_POINT ( 'NONE',  ( 44.97459685856478018, 1.637169565754164280, -6.109999999999996767 ) ) ;
#21175=CARTESIAN_POINT ( 'NONE',  ( 119.6412635252314658, 4.472830434245837594, 4.472830434245841147 ) ) ;
#21218=CARTESIAN_POINT ( 'NONE',  ( 41.18293019189811588, -1.637169565754159173, -6.109999999999999432 ) ) ;
#21240=CARTESIAN_POINT ( 'NONE',  ( 79.02083333333331439, 7.949999999999998401, 2.130196079827431532 ) ) ;
#21246=CARTESIAN_POINT ( 'NONE',  ( 58.85002705046289151, -5.819803920172572198, -5.819803920172572198 ) ) ;
#21251=CARTESIAN_POINT ( 'NONE',  ( 55.10416666666665009, 2.130196079827422206, 7.950000000000001954 ) ) ;
#21258=CARTESIAN_POINT ( 'NONE',  ( 127.0000000000000000, -4.017717506652945580, -5.045834523320674059 ) ) ;
#21264=CARTESIAN_POINT ( 'NONE',  ( 49.00043019189810423, -3.055000000000002380, 5.291415217122920289 ) ) ;
#21281=CARTESIAN_POINT ( 'NONE',  ( 83.70876352523143282, -7.482591942790329030E-16, 6.110000000000001208 ) ) ;
#21291=CARTESIAN_POINT ( 'NONE',  ( 68.45376352523143737, -6.109999999999998543, -3.741295971395162543E-16 ) ) ;
#21312=CARTESIAN_POINT ( 'NONE',  ( 41.78752705046289151, 0.000000000000000000, -7.949999999999998401 ) ) ;
#21313=CARTESIAN_POINT ( 'NONE',  ( 0.000000000000000000, 0.000000000000000000, 0.000000000000000000 ) ) ;
#21321=CARTESIAN_POINT ( 'NONE',  ( 87.99543019189812298, 5.291415217122916737, 3.055000000000001936 ) ) ;
#21345=CARTESIAN_POINT ( 'NONE',  ( 33.54209685856476852, 5.291415217122923842, -3.054999999999996163 ) ) ;
#21353=DIRECTION ( 'NONE',  ( -1.000000000000000000, -0.000000000000000000, -0.000000000000000000 ) ) ;
#21363=DIRECTION ( 'NONE',  ( 0.000000000000000000, 1.000000000000000000, -1.224646799147353207E-16 ) ) ;
#21377=DIRECTION ( 'NONE',  ( 1.000000000000000000, 0.000000000000000000, 0.000000000000000000 ) ) ;
#21402=CARTESIAN_POINT ( 'NONE',  ( 65.97459685856479439, 1.637169565754164280, -6.109999999999997655 ) ) ;
#21423=DIRECTION ( 'NONE',  ( 0.000000000000000000, 0.000000000000000000, 1.000000000000000000 ) ) ;
#21428=CARTESIAN_POINT ( 'NONE',  ( 85.97502705046288440, -5.819803920172572198, 5.819803920172572198 ) ) ;
#21432=CARTESIAN_POINT ( 'NONE',  ( 81.64583333333332860, 2.130196079827431976, -7.949999999999999289 ) ) ;
#21442=CARTESIAN_POINT ( 'NONE',  ( 74.37543019189810423, -5.291415217122920289, -3.055000000000001492 ) ) ;
#21457=CARTESIAN_POINT ( 'NONE',  ( 76.54166666666667140, -3.975000000000002753, 6.884901960086286188 ) ) ;
#21461=CARTESIAN_POINT ( 'NONE',  ( 66.50043019189810423, -3.055000000000002380, 5.291415217122920289 ) ) ;
#21488=CARTESIAN_POINT ( 'NONE',  ( 128.5969355792471447, -3.174999999999999378, -5.499261314031185677 ) ) ;
#21489=CARTESIAN_POINT ( 'NONE',  ( 60.93750000000000000, 5.819803920172574863, -5.819803920172573086 ) ) ;
#21497=CARTESIAN_POINT ( 'NONE',  ( 109.1412635252314374, 4.472830434245835818, 4.472830434245840259 ) ) ;
#21520=CARTESIAN_POINT ( 'NONE',  ( 64.45876352523144703, 0.000000000000000000, -6.110000000000001208 ) ) ;
#21525=CARTESIAN_POINT ( 'NONE',  ( 97.41709685856478984, 3.054999999999998828, 5.291415217122922066 ) ) ;
#21539=CARTESIAN_POINT ( 'NONE',  ( 119.3495968585647944, 6.109999999999996767, 1.637169565754163836 ) ) ;
#21569=EDGE_CURVE ( 'NONE', #61826, #91561, #97997, .T. ) ;
#21571=CARTESIAN_POINT ( 'NONE',  ( 31.64626352523143638, -4.472830434245840259, 4.472830434245839371 ) ) ;
#21593=CARTESIAN_POINT ( 'NONE',  ( 113.5375270504628986, -9.735942053221456900E-16, 7.949999999999998401 ) ) ;
#21610=LINE ( 'NONE', #20153, #39326 ) ;
#21624=CARTESIAN_POINT ( 'NONE',  ( 71.00000000000000000, 0.000000000000000000, -7.950000000000000178 ) ) ;
#21633=CARTESIAN_POINT ( 'NONE',  ( 92.16709685856477563, -3.055000000000000160, -5.291415217122921177 ) ) ;
#21644=CARTESIAN_POINT ( 'NONE',  ( 87.99543019189812298, 5.291415217122916737, 3.055000000000001936 ) ) ;
#21648=CARTESIAN_POINT ( 'NONE',  ( 116.5000000000000000, 0.000000000000000000, -7.950000000000000178 ) ) ;
#21724=CARTESIAN_POINT ( 'NONE',  ( 87.26626352523145158, 4.472830434245839371, -4.472830434245839371 ) ) ;
#21770=CARTESIAN_POINT ( 'NONE',  ( 110.8125000000000142, 5.819803920172571310, 5.819803920172576639 ) ) ;
#21775=CARTESIAN_POINT ( 'NONE',  ( 100.7500000000000000, -9.735942053221458872E-16, 7.950000000000000178 ) ) ;
#21794=CARTESIAN_POINT ( 'NONE',  ( 29.10002705046288085, 5.819803920172570422, 5.819803920172574863 ) ) ;
#21800=CARTESIAN_POINT ( 'NONE',  ( 117.8337635252314470, 6.110000000000001208, 1.122388791418549305E-15 ) ) ;
#21809=CARTESIAN_POINT ( 'NONE',  ( 117.1620968585647802, -5.291415217122919401, 3.054999999999997939 ) ) ;
#21818=CARTESIAN_POINT ( 'NONE',  ( 36.31293019189809002, -1.637169565754159617, -6.110000000000001208 ) ) ;
#21828=CARTESIAN_POINT ( 'NONE',  ( 27.03709685856478373, -3.054999999999998828, -5.291415217122919401 ) ) ;
#21833=ORIENTED_EDGE ( 'NONE', *, *, #27453, .F. ) ;
#21852=CARTESIAN_POINT ( 'NONE',  ( 46.57876352523145158, -7.482591942790325086E-16, 6.109999999999998543 ) ) ;
#21886=CARTESIAN_POINT ( 'NONE',  ( 118.0370968585647802, -3.054999999999999272, -5.291415217122919401 ) ) ;
#21898=CARTESIAN_POINT ( 'NONE',  ( 121.0208333333333144, 7.949999999999998401, 2.130196079827431532 ) ) ;
#21927=CARTESIAN_POINT ( 'NONE',  ( 31.26626352523144092, 4.472830434245839371, -4.472830434245839371 ) ) ;
#21931=CARTESIAN_POINT ( 'NONE',  ( 125.5416666666666572, -3.975000000000002753, 6.884901960086286188 ) ) ;
#21942=CARTESIAN_POINT ( 'NONE',  ( 123.0837635252314470, -6.110000000000001208, -3.741295971395164515E-16 ) ) ;
#21953=CARTESIAN_POINT ( 'NONE',  ( 52.14169371712954160, -2.130196079827424871, -7.949999999999999289 ) ) ;
#21959=CARTESIAN_POINT ( 'NONE',  ( 49.12500000000000000, -7.950000000000000178, -4.867971026610729436E-16 ) ) ;
#21966=CARTESIAN_POINT ( 'NONE',  ( 35.87543019189811133, -5.291415217122920289, -3.055000000000001492 ) ) ;
#21978=CARTESIAN_POINT ( 'NONE',  ( 85.31293019189811844, -1.637169565754159617, -6.110000000000001208 ) ) ;
#21986=CARTESIAN_POINT ( 'NONE',  ( 70.93293019189810877, 1.637169565754156508, 6.110000000000000320 ) ) ;
#22016=CARTESIAN_POINT ( 'NONE',  ( 72.97459685856478018, 1.637169565754164280, -6.109999999999996767 ) ) ;
#22071=ADVANCED_FACE ( 'NONE', ( #77772 ), #108928, .T. ) ;
#22091=CARTESIAN_POINT ( 'NONE',  ( 66.26626352523145158, 4.472830434245839371, -4.472830434245839371 ) ) ;
#22114=CARTESIAN_POINT ( 'NONE',  ( 88.60002705046288440, 5.819803920172570422, 5.819803920172574863 ) ) ;
#22119=CARTESIAN_POINT ( 'NONE',  ( 71.14583333333332860, 2.130196079827431976, -7.949999999999999289 ) ) ;
#22129=CARTESIAN_POINT ( 'NONE',  ( 79.62543019189810423, 5.291415217122919401, 3.055000000000002824 ) ) ;
#22135=DIRECTION ( 'NONE',  ( -1.000000000000000000, -0.000000000000000000, -0.000000000000000000 ) ) ;
#22141=CARTESIAN_POINT ( 'NONE',  ( 77.27083333333332860, -7.949999999999998401, -2.130196079827426203 ) ) ;
#22145=CARTESIAN_POINT ( 'NONE',  ( 64.60459685856477563, 1.637169565754164946, -6.109999999999999432 ) ) ;
#22175=CARTESIAN_POINT ( 'NONE',  ( 99.80793019189812298, -6.109999999999998543, 1.637169565754158507 ) ) ;
#22201=CARTESIAN_POINT ( 'NONE',  ( 56.00043019189809712, -3.055000000000002380, 5.291415217122920289 ) ) ;
#22208=CARTESIAN_POINT ( 'NONE',  ( 101.2087635252314470, -7.482591942790329030E-16, 6.110000000000001208 ) ) ;
#22224=CARTESIAN_POINT ( 'NONE',  ( 121.5370968585647802, -3.054999999999998828, -5.291415217122919401 ) ) ;
#22226=DIRECTION ( 'NONE',  ( -0.000000000000000000, 1.000000000000000000, -0.000000000000000000 ) ) ;
#22259=EDGE_LOOP ( 'NONE', ( #132083, #56128 ) ) ;
#22264=CARTESIAN_POINT ( 'NONE',  ( 114.9958603837962272, -3.974999999999998312, -6.884901960086286188 ) ) ;
#22281=CARTESIAN_POINT ( 'NONE',  ( 32.49999999999998579, 0.000000000000000000, -7.950000000000000178 ) ) ;
#22302=CARTESIAN_POINT ( 'NONE',  ( 88.66709685856477563, -3.055000000000000160, -5.291415217122921177 ) ) ;
#22312=CARTESIAN_POINT ( 'NONE',  ( 88.57876352523145158, -7.482591942790325086E-16, 6.109999999999998543 ) ) ;
#22370=CARTESIAN_POINT ( 'NONE',  ( 127.1670968585647756, -3.055000000000000160, -5.291415217122921177 ) ) ;
#22389=CARTESIAN_POINT ( 'NONE',  ( 106.6833603837962272, -2.130196079827426203, 7.949999999999996625 ) ) ;
#22403=CARTESIAN_POINT ( 'NONE',  ( 85.51626352523145158, -4.472830434245839371, 4.472830434245839371 ) ) ;
#22448=DIRECTION ( 'NONE',  ( -1.000000000000000000, -0.000000000000000000, -0.000000000000000000 ) ) ;
#22455=CARTESIAN_POINT ( 'NONE',  ( 102.2083333333333286, -3.974999999999999201, -6.884901960086287964 ) ) ;
#22479=CARTESIAN_POINT ( 'NONE',  ( 119.5837635252314470, -6.110000000000001208, -3.741295971395164515E-16 ) ) ;
#22486=CARTESIAN_POINT ( 'NONE',  ( 115.7037635252314516, 6.109999999999998543, 1.122388791418548911E-15 ) ) ;
#22493=AXIS2_PLACEMENT_3D ( 'NONE', #86919, #10052, #75335 ) ;
#22494=CARTESIAN_POINT ( 'NONE',  ( 36.89626352523143993, 4.472830434245840259, -4.472830434245839371 ) ) ;
#22504=CARTESIAN_POINT ( 'NONE',  ( 31.99543019189811233, 5.291415217122916737, 3.055000000000001936 ) ) ;
#22535=CARTESIAN_POINT ( 'NONE',  ( 50.66209685856478018, -5.291415217122919401, 3.054999999999997939 ) ) ;
#22566=CARTESIAN_POINT ( 'NONE',  ( 110.3079301918980946, -6.109999999999999432, 1.637169565754158507 ) ) ;
#22572=EDGE_LOOP ( 'NONE', ( #123361, #100491, #115822, #136836 ) ) ;
#22587=VECTOR ( 'NONE', #47612, 1000.000000000000000 ) ;
#22608=CARTESIAN_POINT ( 'NONE',  ( 128.1208603837962130, -6.884901960086286188, 3.974999999999997424 ) ) ;
#22624=CARTESIAN_POINT ( 'NONE',  ( 119.8754301918981184, -5.291415217122920289, -3.055000000000001492 ) ) ;
#22635=CARTESIAN_POINT ( 'NONE',  ( 103.0375270504628986, -9.735942053221456900E-16, 7.949999999999998401 ) ) ;
#22637=CARTESIAN_POINT ( 'NONE',  ( 46.45419371712955581, 6.884901960086283523, 3.975000000000002753 ) ) ;
#22642=CARTESIAN_POINT ( 'NONE',  ( 41.68749999999997868, -5.819803920172573086, 5.819803920172572198 ) ) ;
#22649=CARTESIAN_POINT ( 'NONE',  ( 36.45876352523143282, 0.000000000000000000, -6.110000000000001208 ) ) ;
#22662=CARTESIAN_POINT ( 'NONE',  ( 82.68793019189810423, 6.110000000000002984, -1.637169565754156730 ) ) ;
#22670=CARTESIAN_POINT ( 'NONE',  ( 87.43336038379622721, 2.130196079827431532, -7.949999999999996625 ) ) ;
#22671=CARTESIAN_POINT ( 'NONE',  ( 62.47459685856478018, 1.637169565754164058, -6.109999999999996767 ) ) ;
#22679=EDGE_CURVE ( 'NONE', #49576, #83993, #73852, .T. ) ;
#22702=CARTESIAN_POINT ( 'NONE',  ( 72.39126352523145158, -4.472830434245838482, -4.472830434245838482 ) ) ;
#22759=CARTESIAN_POINT ( 'NONE',  ( 96.18336038379621300, -2.130196079827426203, 7.949999999999996625 ) ) ;
#22773=CARTESIAN_POINT ( 'NONE',  ( 58.97459685856478018, 1.637169565754164280, -6.109999999999997655 ) ) ;
#22776=CARTESIAN_POINT ( 'NONE',  ( 31.87086038379621655, 6.884901960086289741, -3.974999999999993427 ) ) ;
#22797=DIRECTION ( 'NONE',  ( -1.000000000000000000, -0.000000000000000000, -0.000000000000000000 ) ) ;
#22803=CARTESIAN_POINT ( 'NONE',  ( 73.57919371712957002, 3.975000000000002753, -6.884901960086283523 ) ) ;
#22808=CARTESIAN_POINT ( 'NONE',  ( 69.10416666666665719, 2.130196079827422206, 7.950000000000001954 ) ) ;
#22810=DIRECTION ( 'NONE',  ( 0.000000000000000000, 0.000000000000000000, 1.000000000000000000 ) ) ;
#22820=CARTESIAN_POINT ( 'NONE',  ( 67.66709685856477563, -3.055000000000000160, -5.291415217122921177 ) ) ;
#22842=CARTESIAN_POINT ( 'NONE',  ( 63.58376352523143993, -6.110000000000001208, -3.741295971395164515E-16 ) ) ;
#22873=CARTESIAN_POINT ( 'NONE',  ( 103.4537635252314516, -6.109999999999998543, -3.741295971395162543E-16 ) ) ;
#22902=CARTESIAN_POINT ( 'NONE',  ( 51.77126352523143993, 4.472830434245838482, 4.472830434245842035 ) ) ;
#22908=CARTESIAN_POINT ( 'NONE',  ( 92.75043019189810423, 3.055000000000002824, -5.291415217122919401 ) ) ;
#22924=CARTESIAN_POINT ( 'NONE',  ( 122.7037635252314516, 6.109999999999998543, 1.122388791418548911E-15 ) ) ;
#22947=CARTESIAN_POINT ( 'NONE',  ( 6.179508952642605912, 9.395989132568409730, 1.427142123928949013 ) ) ;
#22973=CARTESIAN_POINT ( 'NONE',  ( 116.3083603837962130, 7.949999999999997513, 2.130196079827431088 ) ) ;
#22988=CARTESIAN_POINT ( 'NONE',  ( 95.81293019189807580, -1.637169565754159617, -6.110000000000001208 ) ) ;
#23008=DIRECTION ( 'NONE',  ( 0.000000000000000000, 0.000000000000000000, 1.000000000000000000 ) ) ;
#23016=CARTESIAN_POINT ( 'NONE',  ( 89.39626352523144703, 4.472830434245840259, -4.472830434245839371 ) ) ;
#23023=CARTESIAN_POINT ( 'NONE',  ( 84.80836038379621300, 7.949999999999996625, 2.130196079827431088 ) ) ;
#23031=CARTESIAN_POINT ( 'NONE',  ( 87.84959685856476597, 6.109999999999996767, 1.637169565754163836 ) ) ;
#23040=ORIENTED_EDGE ( 'NONE', *, *, #16286, .T. ) ;
#23068=CARTESIAN_POINT ( 'NONE',  ( 115.2875270504628986, 0.000000000000000000, -7.949999999999998401 ) ) ;
#23078=CARTESIAN_POINT ( 'NONE',  ( 121.6254301918981184, 5.291415217122919401, 3.055000000000002824 ) ) ;
#23109=CARTESIAN_POINT ( 'NONE',  ( 85.37043019189812298, -3.055000000000001936, 5.291415217122918513 ) ) ;
#23111=CARTESIAN_POINT ( 'NONE',  ( 97.93336038379622721, 2.130196079827431532, -7.949999999999996625 ) ) ;
#23163=CARTESIAN_POINT ( 'NONE',  ( 110.2291666666666714, 7.950000000000001954, -2.130196079827421762 ) ) ;
#23167=CARTESIAN_POINT ( 'NONE',  ( 102.6458333333333144, 2.130196079827431976, -7.949999999999999289 ) ) ;
#23175=CARTESIAN_POINT ( 'NONE',  ( 11.74866626111222878, 8.548044547423961248, 4.146786111629948479 ) ) ;
#23181=CARTESIAN_POINT ( 'NONE',  ( 127.5162635252314658, -4.472830434245838482, 4.472830434245838482 ) ) ;
#23194=CARTESIAN_POINT ( 'NONE',  ( 123.5212635252314470, -4.472830434245839371, -4.472830434245840259 ) ) ;
#23204=CARTESIAN_POINT ( 'NONE',  ( 110.7454301918981088, -5.291415217122918513, -3.055000000000000160 ) ) ;
#23218=CARTESIAN_POINT ( 'NONE',  ( 35.58376352523143282, -6.110000000000001208, -3.741295971395164515E-16 ) ) ;
#23224=CARTESIAN_POINT ( 'NONE',  ( 33.45376352523145158, -6.109999999999998543, -3.741295971395162543E-16 ) ) ;
#23255=ORIENTED_EDGE ( 'NONE', *, *, #109265, .T. ) ;
#23257=CARTESIAN_POINT ( 'NONE',  ( 45.41209685856478728, 5.291415217122921177, -3.054999999999994831 ) ) ;
#23258=ORIENTED_EDGE ( 'NONE', *, *, #47475, .F. ) ;
#23266=ADVANCED_FACE ( 'NONE', ( #99703 ), #85984, .F. ) ;
#23292=CARTESIAN_POINT ( 'NONE',  ( 110.8912635252314658, -4.472830434245839371, -4.472830434245839371 ) ) ;
#23342=CARTESIAN_POINT ( 'NONE',  ( 126.3365768546761956, -7.119864409971977004, -0.03876453820169215719 ) ) ;
#23344=CARTESIAN_POINT ( 'NONE',  ( 129.1416937171295558, -2.130196079827424871, -7.949999999999999289 ) ) ;
#23365=CARTESIAN_POINT ( 'NONE',  ( 122.6462635252314328, -4.472830434245840259, 4.472830434245839371 ) ) ;
#23375=CARTESIAN_POINT ( 'NONE',  ( 48.20419371712955581, -6.884901960086285300, -3.975000000000000089 ) ) ;
#23381=CARTESIAN_POINT ( 'NONE',  ( 45.04166666666665719, -3.975000000000002753, 6.884901960086286188 ) ) ;
#23389=CARTESIAN_POINT ( 'NONE',  ( 34.56293019189810423, 1.637169565754157174, 6.110000000000002984 ) ) ;
#23413=CARTESIAN_POINT ( 'NONE',  ( 57.51626352523144448, -4.472830434245839371, 4.472830434245839371 ) ) ;
#23415=ADVANCED_FACE ( 'NONE', ( #5189 ), #58956, .T. ) ;
#23419=CARTESIAN_POINT ( 'NONE',  ( 0.000000000000000000, 0.000000000000000000, 0.000000000000000000 ) ) ;
#23441=DIRECTION ( 'NONE',  ( 0.000000000000000000, 0.000000000000000000, 1.000000000000000000 ) ) ;
#23448=CARTESIAN_POINT ( 'NONE',  ( 76.18293019189810877, -1.637169565754158951, -6.109999999999998543 ) ) ;
#23457=CARTESIAN_POINT ( 'NONE',  ( 122.4791666666666714, -7.950000000000000178, 2.130196079827424427 ) ) ;
#23477=APPLICATION_CONTEXT ( 'automotive_design' ) ;
#23478=CARTESIAN_POINT ( 'NONE',  ( 29.89626352523142927, 4.472830434245840259, -4.472830434245838482 ) ) ;
#23481=CARTESIAN_POINT ( 'NONE',  ( 89.62086038379622721, -6.884901960086286188, 3.974999999999997424 ) ) ;
#23512=AXIS2_PLACEMENT_3D ( 'NONE', #3910, #61255, #49646 ) ;
#23530=CARTESIAN_POINT ( 'NONE',  ( 57.80793019189810877, -6.109999999999999432, 1.637169565754158507 ) ) ;
#23543=CIRCLE ( 'NONE', #30492, 6.349999999999999645 ) ;
#23549=DIRECTION ( 'NONE',  ( 0.000000000000000000, 0.000000000000000000, 1.000000000000000000 ) ) ;
#23558=CARTESIAN_POINT ( 'NONE',  ( 78.24586038379621300, 3.974999999999996980, 6.884901960086287964 ) ) ;
#23562=CARTESIAN_POINT ( 'NONE',  ( 71.72916666666667140, 7.950000000000001954, -2.130196079827421762 ) ) ;
#23571=CARTESIAN_POINT ( 'NONE',  ( 64.16709685856476142, -3.055000000000000160, -5.291415217122921177 ) ) ;
#23591=CARTESIAN_POINT ( 'NONE',  ( 53.37543019189811133, -5.291415217122920289, -3.055000000000001492 ) ) ;
#23622=CARTESIAN_POINT ( 'NONE',  ( 106.3704301918981230, -3.055000000000001492, 5.291415217122917625 ) ) ;
#23632=AXIS2_PLACEMENT_3D ( 'NONE', #46691, #100998, #89417 ) ;
#23655=CARTESIAN_POINT ( 'NONE',  ( 57.31293019189810423, -1.637169565754159617, -6.110000000000001208 ) ) ;
#23659=CARTESIAN_POINT ( 'NONE',  ( 89.97959685856477563, 6.109999999999999432, 1.637169565754164280 ) ) ;
#23701=CARTESIAN_POINT ( 'NONE',  ( 10.03591437549700771, 8.432637487761468265, -4.375000000000003553 ) ) ;
#23727=CARTESIAN_POINT ( 'NONE',  ( 107.5583603837962414, -7.949999999999997513, -2.130196079827425759 ) ) ;
#23748=CARTESIAN_POINT ( 'NONE',  ( 94.93793019189810423, -6.110000000000001208, 1.637169565754158951 ) ) ;
#23768=CARTESIAN_POINT ( 'NONE',  ( 101.2875270504628986, 0.000000000000000000, -7.949999999999998401 ) ) ;
#23776=CARTESIAN_POINT ( 'NONE',  ( 93.47959685856474721, 6.109999999999999432, 1.637169565754164280 ) ) ;
#23784=CARTESIAN_POINT ( 'NONE',  ( 103.2291666666666714, 7.950000000000001954, -2.130196079827421762 ) ) ;
#23788=CARTESIAN_POINT ( 'NONE',  ( 84.34959685856478018, 6.109999999999996767, 1.637169565754163836 ) ) ;
#23837=CARTESIAN_POINT ( 'NONE',  ( 114.1879301918981042, 6.110000000000002984, -1.637169565754156730 ) ) ;
#23871=CARTESIAN_POINT ( 'NONE',  ( 82.01626352523142316, -4.472830434245839371, 4.472830434245839371 ) ) ;
#23886=EDGE_CURVE ( 'NONE', #94004, #125681, #5249, .T. ) ;
#23913=CARTESIAN_POINT ( 'NONE',  ( 47.18336038379622721, -2.130196079827426203, 7.949999999999996625 ) ) ;
#23927=CARTESIAN_POINT ( 'NONE',  ( 92.72916666666664298, 7.950000000000001954, -2.130196079827421762 ) ) ;
#23945=CARTESIAN_POINT ( 'NONE',  ( 26.99999999999998579, 4.092321363584886740, 6.547056572790977746 ) ) ;
#23954=CARTESIAN_POINT ( 'NONE',  ( 124.1045968585647756, 1.637169565754164946, -6.109999999999999432 ) ) ;
#23961=CARTESIAN_POINT ( 'NONE',  ( 115.9954301918981230, 5.291415217122916737, 3.055000000000001936 ) ) ;
#23973=CARTESIAN_POINT ( 'NONE',  ( 28.34959685856477662, 6.109999999999996767, 1.637169565754163836 ) ) ;
#23975=EDGE_LOOP ( 'NONE', ( #59627, #125479, #68697, #16819 ) ) ;
#24006=CARTESIAN_POINT ( 'NONE',  ( 47.01626352523143737, -4.472830434245838482, 4.472830434245838482 ) ) ;
#24039=CARTESIAN_POINT ( 'NONE',  ( 106.3704301918981230, -3.055000000000001936, 5.291415217122918513 ) ) ;
#24076=ORIENTED_EDGE ( 'NONE', *, *, #89113, .F. ) ;
#24082=CARTESIAN_POINT ( 'NONE',  ( 125.6129489383715736, -4.459058803571000595, 6.473095785633507404 ) ) ;
#24099=VECTOR ( 'NONE', #111035, 1000.000000000000000 ) ;
#24103=CARTESIAN_POINT ( 'NONE',  ( 125.4170968585647756, 3.054999999999998828, 5.291415217122922066 ) ) ;
#24113=CARTESIAN_POINT ( 'NONE',  ( 51.26669371712954160, -7.949999999999999289, 2.130196079827424427 ) ) ;
#24119=CARTESIAN_POINT ( 'NONE',  ( 47.81249999999999289, 5.819803920172571310, 5.819803920172575751 ) ) ;
#24126=CARTESIAN_POINT ( 'NONE',  ( 39.66709685856477563, -3.055000000000000160, -5.291415217122921177 ) ) ;
#24146=CARTESIAN_POINT ( 'NONE',  ( 56.49543019189812298, 5.291415217122916737, 3.055000000000001936 ) ) ;
#24178=CARTESIAN_POINT ( 'NONE',  ( 79.39126352523146579, -4.472830434245838482, -4.472830434245838482 ) ) ;
#24180=EDGE_CURVE ( 'NONE', #102725, #93151, #87827, .T. ) ;
#24211=CARTESIAN_POINT ( 'NONE',  ( 42.07919371712954870, 3.975000000000002753, -6.884901960086283523 ) ) ;
#24250=EDGE_LOOP ( 'NONE', ( #96209, #45193, #2320, #131019, #102936 ) ) ;
#24254=CARTESIAN_POINT ( 'NONE',  ( 53.72459685856478018, -1.637169565754161171, 6.109999999999998543 ) ) ;
#24272=CARTESIAN_POINT ( 'NONE',  ( 27.00000000000000355, -4.083527258847093222, -4.862849486279972488 ) ) ;
#24275=CARTESIAN_POINT ( 'NONE',  ( 72.85002705046289861, -5.819803920172572198, -5.819803920172572198 ) ) ;
#24281=CARTESIAN_POINT ( 'NONE',  ( 70.41666666666665719, -6.884901960086287076, -3.975000000000000977 ) ) ;
#24292=CARTESIAN_POINT ( 'NONE',  ( 63.14626352523143282, -4.472830434245840259, 4.472830434245839371 ) ) ;
#24297=CARTESIAN_POINT ( 'NONE',  ( 44.31249999999999289, 5.819803920172571310, 5.819803920172576639 ) ) ;
#24309=CARTESIAN_POINT ( 'NONE',  ( 52.93793019189809002, -6.110000000000001208, 1.637169565754158951 ) ) ;
#24338=CARTESIAN_POINT ( 'NONE',  ( 101.2662635252314374, 4.472830434245838482, -4.472830434245837594 ) ) ;
#24364=CARTESIAN_POINT ( 'NONE',  ( 50.02126352523143282, -4.472830434245838482, -4.472830434245840259 ) ) ;
#24371=CARTESIAN_POINT ( 'NONE',  ( 87.50043019189810423, -3.055000000000002380, 5.291415217122920289 ) ) ;
#24382=CARTESIAN_POINT ( 'NONE',  ( 126.4954301918981230, 5.291415217122917625, 3.055000000000002380 ) ) ;
#24409=CARTESIAN_POINT ( 'NONE',  ( 57.14583333333332860, 2.130196079827431976, -7.949999999999998401 ) ) ;
#24414=CARTESIAN_POINT ( 'NONE',  ( 7.650458736803186888, 8.843704551814687065, 3.473947073368465421 ) ) ;
#24436=CARTESIAN_POINT ( 'NONE',  ( 105.6625270504628844, 7.949999999999998401, 1.460391307983218338E-15 ) ) ;
#24452=CARTESIAN_POINT ( 'NONE',  ( 90.85459685856477563, -1.637169565754161615, 6.110000000000000320 ) ) ;
#24468=CARTESIAN_POINT ( 'NONE',  ( 101.5791937171295558, 3.975000000000002753, -6.884901960086283523 ) ) ;
#24476=CARTESIAN_POINT ( 'NONE',  ( 82.83376352523144703, 6.110000000000001208, 1.122388791418549305E-15 ) ) ;
#24488=CARTESIAN_POINT ( 'NONE',  ( 73.41209685856478018, 5.291415217122921177, -3.054999999999994831 ) ) ;
#24516=ORIENTED_EDGE ( 'NONE', *, *, #18148, .F. ) ;
#24539=CARTESIAN_POINT ( 'NONE',  ( 119.0004301918981184, -3.055000000000002380, 5.291415217122920289 ) ) ;
#24590=VERTEX_POINT ( 'NONE', #48213 ) ;
#24620=CARTESIAN_POINT ( 'NONE',  ( 94.47916666666664298, -7.950000000000001066, 2.130196079827424427 ) ) ;
#24624=ORIENTED_EDGE ( 'NONE', *, *, #6013, .F. ) ;
#24626=CARTESIAN_POINT ( 'NONE',  ( 88.79166666666665719, 3.975000000000003642, -6.884901960086285300 ) ) ;
#24627=CARTESIAN_POINT ( 'NONE',  ( 14.70014206744062690, 9.500065425788731588, 0.2867161110784761102 ) ) ;
#24632=CARTESIAN_POINT ( 'NONE',  ( 125.7873552745503503, 0.9952826964532990317, -7.614395392956494923 ) ) ;
#24634=CARTESIAN_POINT ( 'NONE',  ( 128.2454301918981230, -5.291415217122918513, -3.055000000000000160 ) ) ;
#24644=CARTESIAN_POINT ( 'NONE',  ( 112.1462635252314328, -4.472830434245840259, 4.472830434245839371 ) ) ;
#24648=CARTESIAN_POINT ( 'NONE',  ( 99.14583333333334281, 2.130196079827470168, -7.949999999999977973 ) ) ;
#24654=CARTESIAN_POINT ( 'NONE',  ( 117.8912635252314516, -4.472830434245839371, -4.472830434245839371 ) ) ;
#24668=CARTESIAN_POINT ( 'NONE',  ( 31.55793019189810522, 6.110000000000000320, -1.637169565754156064 ) ) ;
#24674=ORIENTED_EDGE ( 'NONE', *, *, #1920, .T. ) ;
#24675=ORIENTED_EDGE ( 'NONE', *, *, #35226, .T. ) ;
#24678=EDGE_CURVE ( 'NONE', #143427, #116147, #29305, .T. ) ;
#24699=VERTEX_POINT ( 'NONE', #117710 ) ;
#24704=CARTESIAN_POINT ( 'NONE',  ( 39.14126352523145158, 4.472830434245835818, 4.472830434245840259 ) ) ;
#24706=VERTEX_POINT ( 'NONE', #27162 ) ;
#24709=DIRECTION ( 'NONE',  ( -1.000000000000000000, -0.000000000000000000, -0.000000000000000000 ) ) ;
#24740=CARTESIAN_POINT ( 'NONE',  ( 112.7870968585647802, 3.054999999999997939, 5.291415217122920289 ) ) ;
#24776=ADVANCED_FACE ( 'NONE', ( #138080 ), #32172, .T. ) ;
#24778=CARTESIAN_POINT ( 'NONE',  ( 104.2500000000000000, -9.735942053221458872E-16, 7.950000000000000178 ) ) ;
#24780=CARTESIAN_POINT ( 'NONE',  ( 126.3673795226528682, -7.080845498744676725, -0.3407821965100499839 ) ) ;
#24786=CARTESIAN_POINT ( 'NONE',  ( 122.7708333333333286, -7.949999999999999289, -2.130196079827426203 ) ) ;
#24799=CARTESIAN_POINT ( 'NONE',  ( 118.5629301918981042, 1.637169565754157174, 6.110000000000002984 ) ) ;
#24813=CARTESIAN_POINT ( 'NONE',  ( 44.12086038379622721, -6.884901960086286188, 3.974999999999997424 ) ) ;
#24820=CARTESIAN_POINT ( 'NONE',  ( 37.02083333333332149, 7.949999999999999289, 2.130196079827431532 ) ) ;
#24826=EDGE_LOOP ( 'NONE', ( #19906, #90876, #83230, #124829, #66858, #44857, #32174, #94810, #11706, #13472, #6778, #137535, #129058, #23040, #1703, #103612, #107448, #29737, #27327, #31153, #85027, #32216, #111106, #54212, #30347, #97092, #35556, #47882, #15222, #32773, #35666, #66403, #25892, #135592, #140142, #141247, #56332, #112819, #75625, #10544, #65313, #139754, #11477, #32261, #104541, #45613, #24674, #12592, #14813, #129991, #121483, #80789, #8407, #110097, #61779, #110023, #138499, #18135, #119506, #131579, #107451, #77975, #13204, #52, #57985, #113303 ) ) ;
#24830=CARTESIAN_POINT ( 'NONE',  ( 35.58376352523143282, -6.110000000000001208, -3.741295971395164515E-16 ) ) ;
#24851=CARTESIAN_POINT ( 'NONE',  ( 61.30793019189810877, -6.109999999999998543, 1.637169565754158063 ) ) ;
#24877=CARTESIAN_POINT ( 'NONE',  ( 75.30793019189810877, -6.109999999999998543, 1.637169565754158507 ) ) ;
#24899=CARTESIAN_POINT ( 'NONE',  ( 25.08376352523143638, -6.110000000000001208, -3.741295971395164515E-16 ) ) ;
#24911=VECTOR ( 'NONE', #98322, 1000.000000000000000 ) ;
#24921=CARTESIAN_POINT ( 'NONE',  ( 28.12499999999999645, -7.950000000000000178, -4.867971026610729436E-16 ) ) ;
#24934=CARTESIAN_POINT ( 'NONE',  ( 65.55836038379622721, -7.949999999999996625, -2.130196079827426203 ) ) ;
#24939=CARTESIAN_POINT ( 'NONE',  ( 47.03752705046289151, -9.735942053221456900E-16, 7.949999999999998401 ) ) ;
#24941=CARTESIAN_POINT ( 'NONE',  ( 52.55793019189811588, 6.110000000000001208, -1.637169565754156286 ) ) ;
#24951=ADVANCED_FACE ( 'NONE', ( #102449 ), #34312, .T. ) ;
#24965=CARTESIAN_POINT ( 'NONE',  ( 79.70419371712955581, -6.884901960086285300, -3.975000000000000089 ) ) ;
#24971=CARTESIAN_POINT ( 'NONE',  ( 74.79166666666667140, 3.975000000000003642, -6.884901960086285300 ) ) ;
#24982=CARTESIAN_POINT ( 'NONE',  ( 65.62543019189810423, 5.291415217122919401, 3.055000000000002824 ) ) ;
#24984=ORIENTED_EDGE ( 'NONE', *, *, #79741, .F. ) ;
#25004=CARTESIAN_POINT ( 'NONE',  ( 52.20876352523143282, -7.482591942790329030E-16, 6.110000000000001208 ) ) ;
#25012=ORIENTED_EDGE ( 'NONE', *, *, #69124, .F. ) ;
#25020=CARTESIAN_POINT ( 'NONE',  ( 111.7875270504628986, 0.000000000000000000, -7.949999999999998401 ) ) ;
#25037=CARTESIAN_POINT ( 'NONE',  ( 107.3912635252314516, -4.472830434245838482, -4.472830434245838482 ) ) ;
#25051=CARTESIAN_POINT ( 'NONE',  ( 67.50000000000000000, 0.000000000000000000, -7.950000000000000178 ) ) ;
#25061=CARTESIAN_POINT ( 'NONE',  ( 53.95876352523143282, 0.000000000000000000, -6.110000000000001208 ) ) ;
#25065=CARTESIAN_POINT ( 'NONE',  ( 92.31293019189810423, -1.637169565754159617, -6.110000000000001208 ) ) ;
#25102=ORIENTED_EDGE ( 'NONE', *, *, #26008, .F. ) ;
#25105=CARTESIAN_POINT ( 'NONE',  ( 95.30836038379619879, 7.949999999999996625, 2.130196079827431088 ) ) ;
#25137=CARTESIAN_POINT ( 'NONE',  ( 107.8500270504629128, -5.819803920172572198, -5.819803920172572198 ) ) ;
#25138=ADVANCED_FACE ( 'NONE', ( #125620 ), #134559, .T. ) ;
#25157=CARTESIAN_POINT ( 'NONE',  ( 96.25043019189810423, 3.055000000000002824, -5.291415217122919401 ) ) ;
#25170=LINE ( 'NONE', #91857, #26650 ) ;
#25173=CARTESIAN_POINT ( 'NONE',  ( 102.0166937171295558, 7.950000000000000178, -2.130196079827421318 ) ) ;
#25181=CARTESIAN_POINT ( 'NONE',  ( 84.72959685856476142, -6.110000000000000320, -1.637169565754161393 ) ) ;
#25191=CARTESIAN_POINT ( 'NONE',  ( 79.09959685856478018, -6.109999999999997655, -1.637169565754160283 ) ) ;
#25248=CARTESIAN_POINT ( 'NONE',  ( 115.9379301918980900, -6.110000000000001208, 1.637169565754158951 ) ) ;
#25261=ORIENTED_EDGE ( 'NONE', *, *, #105948, .T. ) ;
#25327=CARTESIAN_POINT ( 'NONE',  ( 93.16666666666667140, 6.884901960086285300, 3.975000000000003642 ) ) ;
#25333=CARTESIAN_POINT ( 'NONE',  ( 13.21584829534196182, 8.912386969599870312, 3.296154402857504273 ) ) ;
#25341=CARTESIAN_POINT ( 'NONE',  ( 125.8175036712048609, 1.497365648122270798, -7.501076162823921756 ) ) ;
#25343=CARTESIAN_POINT ( 'NONE',  ( 127.6620968585647802, -5.291415217122919401, 3.054999999999997939 ) ) ;
#25348=CARTESIAN_POINT ( 'NONE',  ( 26.99999999999999289, 5.724939966758856968, 3.387577145584128591 ) ) ;
#25357=CARTESIAN_POINT ( 'NONE',  ( 106.7504301918981184, 3.055000000000002824, -5.291415217122919401 ) ) ;
#25364=CARTESIAN_POINT ( 'NONE',  ( 108.8495968585647660, 6.109999999999996767, 1.637169565754163836 ) ) ;
#25394=CARTESIAN_POINT ( 'NONE',  ( 63.37086038379622011, 6.884901960086289741, -3.974999999999993427 ) ) ;
#25403=CARTESIAN_POINT ( 'NONE',  ( 41.18293019189811588, -1.637169565754158951, -6.109999999999998543 ) ) ;
#25424=VECTOR ( 'NONE', #119309, 1000.000000000000000 ) ;
#25441=ORIENTED_EDGE ( 'NONE', *, *, #33969, .T. ) ;
#25442=CARTESIAN_POINT ( 'NONE',  ( 110.7454301918981088, -5.291415217122919401, -3.055000000000000604 ) ) ;
#25483=CARTESIAN_POINT ( 'NONE',  ( 126.1492088369915194, -7.085075694611017383, 1.787438164688350817 ) ) ;
#25491=CARTESIAN_POINT ( 'NONE',  ( 116.3541666666666856, -2.130196079827425315, -7.950000000000001066 ) ) ;
#25494=VERTEX_POINT ( 'NONE', #109025 ) ;
#25506=CARTESIAN_POINT ( 'NONE',  ( 113.3129301918981042, -1.637169565754159617, -6.110000000000001208 ) ) ;
#25517=CARTESIAN_POINT ( 'NONE',  ( 42.80836038379622011, 7.949999999999997513, 2.130196079827431088 ) ) ;
#25522=CARTESIAN_POINT ( 'NONE',  ( 35.85416666666666430, -2.130196079827425315, -7.950000000000001066 ) ) ;
#25536=CARTESIAN_POINT ( 'NONE',  ( 26.97959685856476497, 6.109999999999999432, 1.637169565754164280 ) ) ;
#25557=EDGE_CURVE ( 'NONE', #7223, #34604, #108287, .T. ) ;
#25559=CARTESIAN_POINT ( 'NONE',  ( 54.89126352523145158, -4.472830434245839371, -4.472830434245839371 ) ) ;
#25583=CARTESIAN_POINT ( 'NONE',  ( 61.89126352523144448, -4.472830434245838482, -4.472830434245838482 ) ) ;
#25635=CARTESIAN_POINT ( 'NONE',  ( 0.000000000000000000, 9.735942053221458872E-16, -7.950000000000000178 ) ) ;
#25666=CARTESIAN_POINT ( 'NONE',  ( 56.93293019189810877, 1.637169565754156730, 6.110000000000001208 ) ) ;
#25692=CARTESIAN_POINT ( 'NONE',  ( 75.47502705046287019, -5.819803920172572198, 5.819803920172572198 ) ) ;
#25695=CARTESIAN_POINT ( 'NONE',  ( 62.39583333333332149, -2.130196079827427091, 7.949999999999999289 ) ) ;
#25707=CARTESIAN_POINT ( 'NONE',  ( 64.89626352523144703, 4.472830434245840259, -4.472830434245839371 ) ) ;
#25708=CARTESIAN_POINT ( 'NONE',  ( 0.000000000000000000, 0.000000000000000000, 0.000000000000000000 ) ) ;
#25718=CARTESIAN_POINT ( 'NONE',  ( 43.14583333333332860, 2.130196079827431976, -7.949999999999998401 ) ) ;
#25755=CARTESIAN_POINT ( 'NONE',  ( 36.68336038379622721, -2.130196079827426203, 7.949999999999996625 ) ) ;
#25761=CARTESIAN_POINT ( 'NONE',  ( 98.34959685856479439, 6.109999999999996767, 1.637169565754163836 ) ) ;
#25773=CARTESIAN_POINT ( 'NONE',  ( 27.78752705046289151, 0.000000000000000000, -7.949999999999998401 ) ) ;
#25785=CARTESIAN_POINT ( 'NONE',  ( 43.60459685856476852, 1.637169565754164946, -6.109999999999999432 ) ) ;
#25841=CARTESIAN_POINT ( 'NONE',  ( 80.33333333333334281, -6.884901960086287964, 3.974999999999998312 ) ) ;
#25867=CARTESIAN_POINT ( 'NONE',  ( 102.8916937171295274, 2.130196079827421762, 7.950000000000001066 ) ) ;
#25885=CARTESIAN_POINT ( 'NONE',  ( 93.62543019189811844, 5.291415217122919401, 3.055000000000002824 ) ) ;
#25892=ORIENTED_EDGE ( 'NONE', *, *, #3980, .T. ) ;
#25899=LINE ( 'NONE', #70853, #61122 ) ;
#25911=CARTESIAN_POINT ( 'NONE',  ( 83.70876352523143282, -7.482591942790329030E-16, 6.110000000000001208 ) ) ;
#25920=CARTESIAN_POINT ( 'NONE',  ( 102.6458333333333286, 2.130196079827470168, -7.949999999999977973 ) ) ;
#25925=CARTESIAN_POINT ( 'NONE',  ( 80.12043019189810877, 3.055000000000001936, -5.291415217122916737 ) ) ;
#25937=CARTESIAN_POINT ( 'NONE',  ( 64.58333333333332860, 6.884901960086290629, -3.974999999999994316 ) ) ;
#25964=CARTESIAN_POINT ( 'NONE',  ( 55.78752705046288440, 0.000000000000000000, -7.949999999999998401 ) ) ;
#25979=CARTESIAN_POINT ( 'NONE',  ( 114.3337635252314470, 6.110000000000001208, 1.122388791418549305E-15 ) ) ;
#26008=EDGE_CURVE ( 'NONE', #93151, #133915, #11662, .T. ) ;
#26048=CARTESIAN_POINT ( 'NONE',  ( 31.84959685856478373, 6.109999999999997655, 1.637169565754163836 ) ) ;
#26050=CARTESIAN_POINT ( 'NONE',  ( 48.49586038379622011, -3.974999999999998312, -6.884901960086286188 ) ) ;
#26052=CARTESIAN_POINT ( 'NONE',  ( 153.6500000000000057, 0.000000000000000000, 4.749999999999997335 ) ) ;
#26063=CARTESIAN_POINT ( 'NONE',  ( 88.20833333333332860, -3.974999999999999201, -6.884901960086287964 ) ) ;
#26072=CARTESIAN_POINT ( 'NONE',  ( 12.27715408423077648, 8.651771236590469982, 3.925780828071965267 ) ) ;
#26077=CARTESIAN_POINT ( 'NONE',  ( 125.9962588284267184, 4.199175705864780284, -6.163519753944560975 ) ) ;
#26092=CARTESIAN_POINT ( 'NONE',  ( 108.7920968585647756, -5.291415217122921177, 3.054999999999999272 ) ) ;
#26101=CARTESIAN_POINT ( 'NONE',  ( 105.3495968585647944, 6.109999999999996767, 1.637169565754163836 ) ) ;
#26124=DIRECTION ( 'NONE',  ( 0.000000000000000000, 0.000000000000000000, 1.000000000000000000 ) ) ;
#26145=CARTESIAN_POINT ( 'NONE',  ( 36.22459685856478728, -1.637169565754160949, 6.109999999999997655 ) ) ;
#26185=CARTESIAN_POINT ( 'NONE',  ( 104.9120968585647802, 5.291415217122922066, -3.054999999999995275 ) ) ;
#26188=LINE ( 'NONE', #123379, #62777 ) ;
#26190=AXIS2_PLACEMENT_3D ( 'NONE', #132438, #135281, #13436 ) ;
#26232=CARTESIAN_POINT ( 'NONE',  ( 122.9166666666666714, -6.884901960086287076, -3.975000000000000977 ) ) ;
#26246=CARTESIAN_POINT ( 'NONE',  ( 111.1254301918981042, 5.291415217122919401, 3.055000000000002824 ) ) ;
#26256=CARTESIAN_POINT ( 'NONE',  ( 34.93336038379622011, 2.130196079827431532, -7.949999999999997513 ) ) ;
#26262=CARTESIAN_POINT ( 'NONE',  ( 36.43750000000000000, 5.819803920172573974, -5.819803920172572198 ) ) ;
#26272=CARTESIAN_POINT ( 'NONE',  ( 29.75043019189810423, 3.055000000000002824, -5.291415217122919401 ) ) ;
#26282=CARTESIAN_POINT ( 'NONE',  ( 62.68749999999999289, -5.819803920172573974, 5.819803920172573086 ) ) ;
#26293=CARTESIAN_POINT ( 'NONE',  ( 48.03709685856477307, -3.054999999999998828, -5.291415217122919401 ) ) ;
#26294=CARTESIAN_POINT ( 'NONE',  ( 123.9375000000000000, 5.819803920172574863, -5.819803920172573086 ) ) ;
#26322=CARTESIAN_POINT ( 'NONE',  ( 63.78709685856477307, 3.054999999999997495, 5.291415217122919401 ) ) ;
#26403=CARTESIAN_POINT ( 'NONE',  ( 47.16209685856477307, -5.291415217122919401, 3.054999999999998384 ) ) ;
#26422=CARTESIAN_POINT ( 'NONE',  ( 66.57919371712955581, 3.975000000000002753, -6.884901960086283523 ) ) ;
#26427=CARTESIAN_POINT ( 'NONE',  ( 66.04166666666667140, -3.975000000000002753, 6.884901960086286188 ) ) ;
#26435=CARTESIAN_POINT ( 'NONE',  ( 58.77126352523142572, 4.472830434245839371, 4.472830434245842035 ) ) ;
#26445=CARTESIAN_POINT ( 'NONE',  ( 85.87500000000000000, 7.950000000000000178, 1.460391307983218535E-15 ) ) ;
#26459=CARTESIAN_POINT ( 'NONE',  ( 111.6416937171295842, -2.130196079827424871, -7.949999999999998401 ) ) ;
#26487=CARTESIAN_POINT ( 'NONE',  ( 96.59959685856476597, -6.109999999999997655, -1.637169565754160283 ) ) ;
#26513=CARTESIAN_POINT ( 'NONE',  ( 41.70876352523143993, -7.482591942790329030E-16, 6.110000000000001208 ) ) ;
#26523=DIRECTION ( 'NONE',  ( -0.000000000000000000, 1.000000000000000000, -0.000000000000000000 ) ) ;
#26562=CARTESIAN_POINT ( 'NONE',  ( 71.22459685856478018, -1.637169565754161171, 6.109999999999998543 ) ) ;
#26563=CARTESIAN_POINT ( 'NONE',  ( 74.45419371712955581, 6.884901960086283523, 3.975000000000002753 ) ) ;
#26580=CARTESIAN_POINT ( 'NONE',  ( 121.5583603837962272, -7.949999999999996625, -2.130196079827426203 ) ) ;
#26584=CARTESIAN_POINT ( 'NONE',  ( 100.7041937171295558, -6.884901960086285300, -3.975000000000000089 ) ) ;
#26601=CARTESIAN_POINT ( 'NONE',  ( 86.47959685856477563, 6.109999999999999432, 1.637169565754164280 ) ) ;
#26623=CARTESIAN_POINT ( 'NONE',  ( 84.29209685856477563, -5.291415217122921177, 3.054999999999999272 ) ) ;
#26632=CARTESIAN_POINT ( 'NONE',  ( 57.53752705046289151, -9.735942053221456900E-16, 7.949999999999998401 ) ) ;
#26634=CARTESIAN_POINT ( 'NONE',  ( 72.68293019189810877, -1.637169565754158951, -6.109999999999998543 ) ) ;
#26650=VECTOR ( 'NONE', #125216, 1000.000000000000000 ) ;
#26678=CARTESIAN_POINT ( 'NONE',  ( 75.97959685856477563, 6.109999999999999432, 1.637169565754164280 ) ) ;
#26685=CARTESIAN_POINT ( 'NONE',  ( 107.9170968585647756, 3.054999999999998828, 5.291415217122922066 ) ) ;
#26705=CARTESIAN_POINT ( 'NONE',  ( 113.0000000000000000, 0.000000000000000000, -7.950000000000000178 ) ) ;
#26715=CARTESIAN_POINT ( 'NONE',  ( 13.22094965600862970, -8.914091344047001542, 3.291399616463569267 ) ) ;
#26730=VERTEX_POINT ( 'NONE', #75734 ) ;
#26731=CARTESIAN_POINT ( 'NONE',  ( 73.47916666666665719, -7.950000000000000178, 2.130196079827424427 ) ) ;
#26748=CARTESIAN_POINT ( 'NONE',  ( 30.09959685856478018, -6.109999999999998543, -1.637169565754160727 ) ) ;
#26762=CARTESIAN_POINT ( 'NONE',  ( 90.25000000000000000, -9.735942053221458872E-16, 7.950000000000000178 ) ) ;
#26774=CARTESIAN_POINT ( 'NONE',  ( 126.0262699974396838, 4.592503512758394635, -5.848864093691881649 ) ) ;
#26786=EDGE_CURVE ( 'NONE', #55968, #66284, #128494, .T. ) ;
#26791=CARTESIAN_POINT ( 'NONE',  ( 107.3337635252314470, 6.110000000000001208, 1.122388791418549305E-15 ) ) ;
#26802=CARTESIAN_POINT ( 'NONE',  ( 103.8912635252314516, -4.472830434245839371, -4.472830434245839371 ) ) ;
#26809=ORIENTED_EDGE ( 'NONE', *, *, #109435, .F. ) ;
#26814=PRESENTATION_STYLE_ASSIGNMENT (( #66947 ) ) ;
#26835=CARTESIAN_POINT ( 'NONE',  ( 63.51669371712956291, 7.950000000000000178, -2.130196079827421318 ) ) ;
#26844=CARTESIAN_POINT ( 'NONE',  ( 35.78709685856478018, 3.054999999999997495, 5.291415217122919401 ) ) ;
#26882=CARTESIAN_POINT ( 'NONE',  ( 98.20376352523145158, 6.109999999999999432, 1.122388791418549108E-15 ) ) ;
#26931=CARTESIAN_POINT ( 'NONE',  ( 124.5208333333333428, 7.949999999999999289, 2.130196079827431532 ) ) ;
#26942=CARTESIAN_POINT ( 'NONE',  ( 108.5004301918981184, -3.055000000000002380, 5.291415217122920289 ) ) ;
#26946=CARTESIAN_POINT ( 'NONE',  ( 106.5375270504628844, -9.735942053221456900E-16, 7.949999999999998401 ) ) ;
#26951=CARTESIAN_POINT ( 'NONE',  ( 39.45419371712956291, 6.884901960086283523, 3.975000000000002753 ) ) ;
#26952=CIRCLE ( 'NONE', #73231, 6.349999999999997868 ) ;
#26957=CARTESIAN_POINT ( 'NONE',  ( 39.79166666666665719, 3.975000000000003642, -6.884901960086285300 ) ) ;
#26965=EDGE_CURVE ( 'NONE', #30975, #68687, #27047, .T. ) ;
#26969=CARTESIAN_POINT ( 'NONE',  ( 30.47959685856476852, 6.109999999999999432, 1.637169565754164280 ) ) ;
#26980=ORIENTED_EDGE ( 'NONE', *, *, #83909, .T. ) ;
#26992=CARTESIAN_POINT ( 'NONE',  ( 48.32876352523145158, 0.000000000000000000, -6.109999999999998543 ) ) ;
#27019=CARTESIAN_POINT ( 'NONE',  ( 62.47459685856478018, 1.637169565754164280, -6.109999999999996767 ) ) ;
#27022=CARTESIAN_POINT ( 'NONE',  ( 0.000000000000000000, 9.735942053221458872E-16, -7.950000000000000178 ) ) ;
#27042=CARTESIAN_POINT ( 'NONE',  ( 54.76669371712954870, -7.949999999999998401, 2.130196079827423983 ) ) ;
#27045=CARTESIAN_POINT ( 'NONE',  ( 28.99999999999999645, 0.000000000000000000, -7.950000000000000178 ) ) ;
#27047=LINE ( 'NONE', #114748, #118055 ) ;
#27049=CARTESIAN_POINT ( 'NONE',  ( 42.51669371712955581, 7.950000000000000178, -2.130196079827421318 ) ) ;
#27067=CARTESIAN_POINT ( 'NONE',  ( 125.3739199777178754, -1.810106405121186368, 7.950000000000005507 ) ) ;
#27095=CARTESIAN_POINT ( 'NONE',  ( 49.93293019189810167, 1.637169565754156730, 6.110000000000001208 ) ) ;
#27116=CARTESIAN_POINT ( 'NONE',  ( 63.37086038379622011, 6.884901960086289741, -3.974999999999993427 ) ) ;
#27122=CARTESIAN_POINT ( 'NONE',  ( 63.12500000000000000, -7.950000000000000178, -4.867971026610729436E-16 ) ) ;
#27134=CARTESIAN_POINT ( 'NONE',  ( 54.97959685856476852, 6.109999999999999432, 1.637169565754164280 ) ) ;
#27162=CARTESIAN_POINT ( 'NONE',  ( 123.5000000000000000, 0.000000000000000000, -7.950000000000000178 ) ) ;
#27183=CARTESIAN_POINT ( 'NONE',  ( 94.99543019189812298, 5.291415217122916737, 3.055000000000001936 ) ) ;
#27192=DIRECTION ( 'NONE',  ( 0.000000000000000000, 0.000000000000000000, 1.000000000000000000 ) ) ;
#27207=CARTESIAN_POINT ( 'NONE',  ( 46.81293019189811133, -1.637169565754159617, -6.110000000000001208 ) ) ;
#27254=CARTESIAN_POINT ( 'NONE',  ( 77.20376352523145158, 6.109999999999999432, 1.122388791418549108E-15 ) ) ;
#27256=CARTESIAN_POINT ( 'NONE',  ( 80.62500000000000000, -7.950000000000000178, -4.867971026610729436E-16 ) ) ;
#27278=CARTESIAN_POINT ( 'NONE',  ( 90.93336038379621300, 2.130196079827431532, -7.949999999999997513 ) ) ;
#27279=CARTESIAN_POINT ( 'NONE',  ( 72.60416666666665719, 2.130196079827422206, 7.950000000000001954 ) ) ;
#27292=CARTESIAN_POINT ( 'NONE',  ( 45.57919371712955581, 3.975000000000002753, -6.884901960086283523 ) ) ;
#27294=CARTESIAN_POINT ( 'NONE',  ( 85.75043019189810423, 3.055000000000002824, -5.291415217122919401 ) ) ;
#27302=CARTESIAN_POINT ( 'NONE',  ( 117.0375270504628986, -9.735942053221456900E-16, 7.949999999999998401 ) ) ;
#27306=ORIENTED_EDGE ( 'NONE', *, *, #139933, .T. ) ;
#27311=( BOUNDED_CURVE ( )  B_SPLINE_CURVE ( 2, ( #24272, #2481, #66365, #55490, #12663 ),
 .UNSPECIFIED., .F., .T. ) 
 B_SPLINE_CURVE_WITH_KNOTS ( ( 3, 2, 3 ),
 ( 0.9703747093734275131, 0.9722222222222222099, 0.9749999999999999778 ),
 .UNSPECIFIED. ) 
 CURVE ( )  GEOMETRIC_REPRESENTATION_ITEM ( )  RATIONAL_B_SPLINE_CURVE ( ( 0.9848206055686921090, 0.9773371094525169500, 1.000000000000000000, 0.9659258262890684232, 1.000000000000000000 ) ) 
 REPRESENTATION_ITEM ( '' )  );
#27315=CARTESIAN_POINT ( 'NONE',  ( 78.45876352523144703, 0.000000000000000000, -6.110000000000001208 ) ) ;
#27322=ORIENTED_EDGE ( 'NONE', *, *, #65445, .T. ) ;
#27327=ORIENTED_EDGE ( 'NONE', *, *, #35134, .T. ) ;
#27366=CARTESIAN_POINT ( 'NONE',  ( 75.54209685856477563, 5.291415217122923842, -3.054999999999996163 ) ) ;
#27372=CARTESIAN_POINT ( 'NONE',  ( 109.8129301918981184, -1.637169565754159617, -6.110000000000001208 ) ) ;
#27393=CARTESIAN_POINT ( 'NONE',  ( 114.6041666666666856, 2.130196079827402666, 7.950000000000014388 ) ) ;
#27440=CARTESIAN_POINT ( 'NONE',  ( 125.2041937171295700, -6.884901960086285300, -3.975000000000000089 ) ) ;
#27453=EDGE_CURVE ( 'NONE', #68687, #74997, #90357, .T. ) ;
#27456=CARTESIAN_POINT ( 'NONE',  ( 80.04166666666665719, -3.975000000000002753, 6.884901960086286188 ) ) ;
#27471=CARTESIAN_POINT ( 'NONE',  ( 126.4635698499963752, 6.971130382529067582, 0.5264722768656378005 ) ) ;
#27484=CARTESIAN_POINT ( 'NONE',  ( 109.3754301918981042, -5.291415217122920289, -3.055000000000001492 ) ) ;
#27493=CARTESIAN_POINT ( 'NONE',  ( 106.8079301918981230, -6.109999999999998543, 1.637169565754158063 ) ) ;
#27522=CARTESIAN_POINT ( 'NONE',  ( 112.2037635252314516, 6.109999999999998543, 1.122388791418548911E-15 ) ) ;
#27542=CARTESIAN_POINT ( 'NONE',  ( 41.62043019189810877, 3.055000000000001936, -5.291415217122916737 ) ) ;
#27584=CARTESIAN_POINT ( 'NONE',  ( 99.37043019189812298, -3.055000000000001936, 5.291415217122918513 ) ) ;
#27630=CARTESIAN_POINT ( 'NONE',  ( 26.33642480454907187, 4.648522628062373485, -4.648522628062370821 ) ) ;
#27631=CARTESIAN_POINT ( 'NONE',  ( 29.39169371712955936, 2.130196079827421762, 7.950000000000000178 ) ) ;
#27637=CARTESIAN_POINT ( 'NONE',  ( 119.4166666666666714, -6.884901960086287076, -3.975000000000000977 ) ) ;
#27650=CARTESIAN_POINT ( 'NONE',  ( 113.8962635252314328, 4.472830434245840259, -4.472830434245839371 ) ) ;
#27660=CARTESIAN_POINT ( 'NONE',  ( 33.62086038379622011, -6.884901960086286188, 3.974999999999997424 ) ) ;
#27665=CARTESIAN_POINT ( 'NONE',  ( 33.95833333333332860, 3.974999999999997424, 6.884901960086288852 ) ) ;
#27669=CARTESIAN_POINT ( 'NONE',  ( 150.3000000000000114, 0.000000000000000000, 0.000000000000000000 ) ) ;
#27675=CARTESIAN_POINT ( 'NONE',  ( 31.06293019189809712, 1.637169565754157174, 6.110000000000002984 ) ) ;
#27689=CARTESIAN_POINT ( 'NONE',  ( 59.35459685856476142, -1.637169565754161615, 6.110000000000000320 ) ) ;
#27700=CARTESIAN_POINT ( 'NONE',  ( 49.93293019189810167, 1.637169565754156508, 6.110000000000000320 ) ) ;
#27735=CARTESIAN_POINT ( 'NONE',  ( 65.97459685856478018, 1.637169565754164280, -6.109999999999996767 ) ) ;
#27741=CARTESIAN_POINT ( 'NONE',  ( 34.54166666666666430, -3.975000000000002753, 6.884901960086286188 ) ) ;
#27784=CARTESIAN_POINT ( 'NONE',  ( 0.000000000000000000, 0.000000000000000000, 0.000000000000000000 ) ) ;
#27814=CARTESIAN_POINT ( 'NONE',  ( 46.14126352523144448, 4.472830434245837594, 4.472830434245841147 ) ) ;
#27818=ORIENTED_EDGE ( 'NONE', *, *, #25557, .T. ) ;
#27838=CARTESIAN_POINT ( 'NONE',  ( 68.62086038379622721, -6.884901960086286188, 3.974999999999997424 ) ) ;
#27843=CARTESIAN_POINT ( 'NONE',  ( 68.66666666666665719, 6.884901960086285300, 3.975000000000003642 ) ) ;
#27851=CARTESIAN_POINT ( 'NONE',  ( 55.56293019189809712, 1.637169565754157174, 6.110000000000002984 ) ) ;
#27862=CARTESIAN_POINT ( 'NONE',  ( 100.7041937171295558, -6.884901960086285300, -3.975000000000000089 ) ) ;
#27875=CARTESIAN_POINT ( 'NONE',  ( 111.2041937171295558, -6.884901960086285300, -3.975000000000000089 ) ) ;
#27890=CARTESIAN_POINT ( 'NONE',  ( 61.32919371712955581, -3.975000000000001865, 6.884901960086284411 ) ) ;
#27907=CARTESIAN_POINT ( 'NONE',  ( 96.74543019189810877, -5.291415217122918513, -3.055000000000000160 ) ) ;
#27928=AXIS2_PLACEMENT_3D ( 'NONE', #99653, #111238, #132333 ) ;
#27935=CARTESIAN_POINT ( 'NONE',  ( 44.18793019189811133, 6.110000000000002984, -1.637169565754156730 ) ) ;
#27970=CARTESIAN_POINT ( 'NONE',  ( 66.18749999999998579, -5.819803920172573974, 5.819803920172573086 ) ) ;
#27988=CARTESIAN_POINT ( 'NONE',  ( 75.59959685856478018, -6.109999999999998543, -1.637169565754160727 ) ) ;
#28017=CARTESIAN_POINT ( 'NONE',  ( 89.32919371712955581, -3.975000000000001865, 6.884901960086284411 ) ) ;
#28028=ORIENTED_EDGE ( 'NONE', *, *, #139767, .F. ) ;
#28030=CARTESIAN_POINT ( 'NONE',  ( 45.72502705046288440, 5.819803920172573974, -5.819803920172573086 ) ) ;
#28034=CARTESIAN_POINT ( 'NONE',  ( 82.83376352523144703, 6.110000000000001208, 1.122388791418549305E-15 ) ) ;
#28043=CARTESIAN_POINT ( 'NONE',  ( 118.6416937171303516, -2.130196079817768595, -7.950000000005574385 ) ) ;
#28051=CARTESIAN_POINT ( 'NONE',  ( 59.62500000000000000, -7.950000000000000178, -4.867971026610729436E-16 ) ) ;
#28054=CARTESIAN_POINT ( 'NONE',  ( 72.62543019189810423, 5.291415217122919401, 3.055000000000002824 ) ) ;
#28097=AXIS2_PLACEMENT_3D ( 'NONE', #143408, #576, #54298 ) ;
#28112=CARTESIAN_POINT ( 'NONE',  ( 77.72959685856477563, -6.110000000000000320, -1.637169565754161393 ) ) ;
#28117=CARTESIAN_POINT ( 'NONE',  ( 111.8545968585647756, -1.637169565754161615, 6.110000000000000320 ) ) ;
#28126=CARTESIAN_POINT ( 'NONE',  ( 35.07919371712955581, 3.975000000000002753, -6.884901960086283523 ) ) ;
#28138=CARTESIAN_POINT ( 'NONE',  ( 113.7291666666666572, 7.950000000000001954, -2.130196079827421762 ) ) ;
#28177=CARTESIAN_POINT ( 'NONE',  ( 105.8541666666666714, -2.130196079827445299, -7.949999999999990408 ) ) ;
#28186=CARTESIAN_POINT ( 'NONE',  ( 117.3291937171295558, -3.975000000000001865, 6.884901960086284411 ) ) ;
#28202=CARTESIAN_POINT ( 'NONE',  ( 78.58333333333334281, 6.884901960086290629, -3.974999999999994316 ) ) ;
#28219=STYLED_ITEM ( 'NONE', ( #108786 ), #142006 ) ;
#28228=CARTESIAN_POINT ( 'NONE',  ( 102.5212635252314328, -4.472830434245839371, -4.472830434245840259 ) ) ;
#28237=CARTESIAN_POINT ( 'NONE',  ( 106.0787635252314516, -7.482591942790325086E-16, 6.109999999999998543 ) ) ;
#28266=CARTESIAN_POINT ( 'NONE',  ( 110.4537635252314516, -6.109999999999998543, -3.741295971395162543E-16 ) ) ;
#28268=FACE_OUTER_BOUND ( 'NONE', #50792, .T. ) ;
#28279=CARTESIAN_POINT ( 'NONE',  ( 37.02083333333332149, 7.949999999999998401, 2.130196079827431532 ) ) ;
#28290=CARTESIAN_POINT ( 'NONE',  ( 33.30793019189810877, -6.109999999999998543, 1.637169565754158507 ) ) ;
#28303=EDGE_CURVE ( 'NONE', #113567, #72906, #37009, .T. ) ;
#28331=CARTESIAN_POINT ( 'NONE',  ( 103.0162635252314374, -4.472830434245839371, 4.472830434245839371 ) ) ;
#28374=EDGE_CURVE ( 'NONE', #10908, #129366, #51853, .T. ) ;
#28380=CARTESIAN_POINT ( 'NONE',  ( 112.5624999999999858, -5.819803920172572198, -5.819803920172573086 ) ) ;
#28391=CARTESIAN_POINT ( 'NONE',  ( 110.5420968585647756, 5.291415217122923842, -3.054999999999996163 ) ) ;
#28399=CARTESIAN_POINT ( 'NONE',  ( 40.76669371712956291, -7.949999999999999289, 2.130196079827424427 ) ) ;
#28404=CARTESIAN_POINT ( 'NONE',  ( 25.20833333333333215, -3.974999999999999201, -6.884901960086287964 ) ) ;
#28417=CARTESIAN_POINT ( 'NONE',  ( 25.22959685856476142, -6.110000000000000320, -1.637169565754161393 ) ) ;
#28428=CARTESIAN_POINT ( 'NONE',  ( 57.45876352523143993, 0.000000000000000000, -6.110000000000001208 ) ) ;
#28439=CARTESIAN_POINT ( 'NONE',  ( 46.14126352523144448, 4.472830434245836706, 4.472830434245840259 ) ) ;
#28472=CARTESIAN_POINT ( 'NONE',  ( 65.24543019189810877, -5.291415217122918513, -3.055000000000000160 ) ) ;
#28504=ORIENTED_EDGE ( 'NONE', *, *, #73493, .T. ) ;
#28547=CARTESIAN_POINT ( 'NONE',  ( 47.74543019189811588, -5.291415217122919401, -3.055000000000000604 ) ) ;
#28572=CARTESIAN_POINT ( 'NONE',  ( 66.14169371712955581, -2.130196079827424871, -7.949999999999999289 ) ) ;
#28578=CARTESIAN_POINT ( 'NONE',  ( 60.20833333333333570, -3.974999999999999201, -6.884901960086287964 ) ) ;
#28586=CARTESIAN_POINT ( 'NONE',  ( 61.10459685856476852, 1.637169565754164946, -6.109999999999999432 ) ) ;
#28600=CARTESIAN_POINT ( 'NONE',  ( 100.4125270504628986, -7.949999999999998401, -4.867971026610728450E-16 ) ) ;
#28619=CARTESIAN_POINT ( 'NONE',  ( 72.12086038379622721, -6.884901960086286188, 3.974999999999997424 ) ) ;
#28646=CARTESIAN_POINT ( 'NONE',  ( 89.74543019189812298, -5.291415217122918513, -3.055000000000000160 ) ) ;
#28672=CARTESIAN_POINT ( 'NONE',  ( 46.08376352523143993, -6.110000000000001208, -3.741295971395164515E-16 ) ) ;
#28684=DIRECTION ( 'NONE',  ( -1.000000000000000000, -0.000000000000000000, -0.000000000000000000 ) ) ;
#28689=DIRECTION ( 'NONE',  ( 0.000000000000000000, 0.000000000000000000, 1.000000000000000000 ) ) ;
#28690=ORIENTED_EDGE ( 'NONE', *, *, #66417, .F. ) ;
#28721=CARTESIAN_POINT ( 'NONE',  ( 73.55793019189812298, 6.110000000000001208, -1.637169565754156286 ) ) ;
#28728=CYLINDRICAL_SURFACE ( 'NONE', #34940, 7.950000000000000178 ) ;
#28745=CARTESIAN_POINT ( 'NONE',  ( 93.12086038379622721, -6.884901960086286188, 3.974999999999997424 ) ) ;
#28757=CARTESIAN_POINT ( 'NONE',  ( 81.95876352523143282, 0.000000000000000000, -6.110000000000001208 ) ) ;
#28779=CARTESIAN_POINT ( 'NONE',  ( 75.97959685856477563, 6.109999999999999432, 1.637169565754164280 ) ) ;
#28830=CARTESIAN_POINT ( 'NONE',  ( 75.68793019189809002, 6.110000000000002984, -1.637169565754156730 ) ) ;
#28836=CARTESIAN_POINT ( 'NONE',  ( 104.5629301918980900, 1.637169565754157174, 6.110000000000002984 ) ) ;
#28869=CARTESIAN_POINT ( 'NONE',  ( 14.47191377450093697, -9.396605767970752865, -1.423631233415600050 ) ) ;
#28884=CARTESIAN_POINT ( 'NONE',  ( 73.91666666666665719, -6.884901960086287076, -3.975000000000000977 ) ) ;
#28899=CARTESIAN_POINT ( 'NONE',  ( 126.2250270504628986, 5.819803920172573086, -5.819803920172572198 ) ) ;
#28914=CARTESIAN_POINT ( 'NONE',  ( 82.08333333333334281, 6.884901960086290629, -3.974999999999994316 ) ) ;
#28917=CARTESIAN_POINT ( 'NONE',  ( 92.39169371712955581, 2.130196079827421762, 7.950000000000000178 ) ) ;
#28937=CARTESIAN_POINT ( 'NONE',  ( 100.0420968585647756, 5.291415217122923842, -3.054999999999996163 ) ) ;
#28948=CARTESIAN_POINT ( 'NONE',  ( 97.62043019189812298, 3.055000000000001936, -5.291415217122916737 ) ) ;
#28954=LINE ( 'NONE', #85446, #102487 ) ;
#28976=CARTESIAN_POINT ( 'NONE',  ( 113.6620968585647944, -5.291415217122919401, 3.054999999999997939 ) ) ;
#28977=CYLINDRICAL_SURFACE ( 'NONE', #60545, 4.749999999999997335 ) ;
#28999=CARTESIAN_POINT ( 'NONE',  ( 31.12043019189811233, 3.055000000000001936, -5.291415217122916737 ) ) ;
#29032=CARTESIAN_POINT ( 'NONE',  ( 102.1412635252314232, 4.472830434245837594, 4.472830434245841147 ) ) ;
#29083=CARTESIAN_POINT ( 'NONE',  ( 108.1874999999999858, -5.819803920172573086, 5.819803920172572198 ) ) ;
#29094=CARTESIAN_POINT ( 'NONE',  ( 101.9379301918980900, -6.110000000000001208, 1.637169565754158951 ) ) ;
#29102=CARTESIAN_POINT ( 'NONE',  ( 38.57919371712956291, 3.975000000000002753, -6.884901960086283523 ) ) ;
#29108=CARTESIAN_POINT ( 'NONE',  ( 30.45833333333332504, 3.974999999999997424, 6.884901960086288852 ) ) ;
#29117=CARTESIAN_POINT ( 'NONE',  ( 125.3287635252314516, 0.000000000000000000, -6.109999999999998543 ) ) ;
#29126=CARTESIAN_POINT ( 'NONE',  ( 46.95876352523143993, 0.000000000000000000, -6.110000000000001208 ) ) ;
#29137=CARTESIAN_POINT ( 'NONE',  ( 51.09959685856477307, -6.109999999999997655, -1.637169565754160283 ) ) ;
#29146=CARTESIAN_POINT ( 'NONE',  ( 60.30836038379622011, 7.949999999999996625, 2.130196079827431088 ) ) ;
#29148=CARTESIAN_POINT ( 'NONE',  ( 43.53752705046289151, -9.735942053221456900E-16, 7.949999999999998401 ) ) ;
#29163=CARTESIAN_POINT ( 'NONE',  ( 57.07876352523144448, -7.482591942790325086E-16, 6.109999999999998543 ) ) ;
#29174=CARTESIAN_POINT ( 'NONE',  ( 100.7500000000000000, -9.735942053221458872E-16, 7.950000000000000178 ) ) ;
#29185=CARTESIAN_POINT ( 'NONE',  ( 55.64169371712955581, -2.130196079827424871, -7.949999999999998401 ) ) ;
#29193=CARTESIAN_POINT ( 'NONE',  ( 128.0995968585647802, -6.109999999999998543, -1.637169565754160727 ) ) ;
#29202=CARTESIAN_POINT ( 'NONE',  ( 76.35002705046288440, -5.819803920172573086, -5.819803920172573086 ) ) ;
#29234=CARTESIAN_POINT ( 'NONE',  ( 49.20376352523145158, 6.109999999999999432, 1.122388791418549108E-15 ) ) ;
#29260=CARTESIAN_POINT ( 'NONE',  ( 67.01669371712957002, 7.950000000000001066, -2.130196079827421318 ) ) ;
#29263=ORIENTED_EDGE ( 'NONE', *, *, #15031, .F. ) ;
#29265=CARTESIAN_POINT ( 'NONE',  ( 54.95833333333332860, 3.974999999999997424, 6.884901960086288852 ) ) ;
#29274=CARTESIAN_POINT ( 'NONE',  ( 57.16709685856477563, -3.055000000000000160, -5.291415217122921177 ) ) ;
#29298=CARTESIAN_POINT ( 'NONE',  ( 72.24543019189810877, -5.291415217122918513, -3.055000000000000160 ) ) ;
#29305=LINE ( 'NONE', #139545, #114035 ) ;
#29310=ORIENTED_EDGE ( 'NONE', *, *, #125828, .T. ) ;
#29325=CARTESIAN_POINT ( 'NONE',  ( 87.41209685856478018, 5.291415217122921177, -3.054999999999994831 ) ) ;
#29346=CARTESIAN_POINT ( 'NONE',  ( 33.25043019189810423, 3.055000000000002824, -5.291415217122919401 ) ) ;
#29359=CYLINDRICAL_SURFACE ( 'NONE', #38281, 7.950000000000000178 ) ;
#29391=CARTESIAN_POINT ( 'NONE',  ( 96.22916666666667140, 7.950000000000001954, -2.130196079827421762 ) ) ;
#29404=CARTESIAN_POINT ( 'NONE',  ( 76.91209685856479439, 5.291415217122922066, -3.054999999999995275 ) ) ;
#29421=VERTEX_POINT ( 'NONE', #107311 ) ;
#29426=CARTESIAN_POINT ( 'NONE',  ( 96.62086038379621300, -6.884901960086286188, 3.974999999999997424 ) ) ;
#29430=LINE ( 'NONE', #129462, #63165 ) ;
#29439=CARTESIAN_POINT ( 'NONE',  ( 83.27126352523143282, 4.472830434245839371, 4.472830434245842035 ) ) ;
#29445=ADVANCED_FACE ( 'NONE', ( #84854 ), #85547, .T. ) ;
#29462=CARTESIAN_POINT ( 'NONE',  ( 71.89626352523144703, 4.472830434245840259, -4.472830434245839371 ) ) ;
#29503=CARTESIAN_POINT ( 'NONE',  ( 26.99999999999999289, -4.294289084967417125, -4.784050195499812475 ) ) ;
#29514=CARTESIAN_POINT ( 'NONE',  ( 71.60459685856476142, 1.637169565754164946, -6.109999999999999432 ) ) ;
#29520=CARTESIAN_POINT ( 'NONE',  ( 113.6045968585647614, 1.637169565754164946, -6.109999999999999432 ) ) ;
#29527=CARTESIAN_POINT ( 'NONE',  ( 77.37086038379622721, 6.884901960086289741, -3.974999999999993427 ) ) ;
#29561=ADVANCED_FACE ( 'NONE', ( #12979 ), #110846, .T. ) ;
#29569=CARTESIAN_POINT ( 'NONE',  ( 28.87543019189810067, -5.291415217122920289, -3.055000000000001492 ) ) ;
#29573=CARTESIAN_POINT ( 'NONE',  ( 26.45376352523144803, -6.109999999999998543, -3.741295971395162543E-16 ) ) ;
#29589=CARTESIAN_POINT ( 'NONE',  ( 120.5375270504628844, -9.735942053221456900E-16, 7.949999999999998401 ) ) ;
#29601=CARTESIAN_POINT ( 'NONE',  ( 85.14583333333334281, 2.130196079827431976, -7.949999999999999289 ) ) ;
#29625=CARTESIAN_POINT ( 'NONE',  ( 105.8754301918981042, -5.291415217122920289, -3.055000000000001492 ) ) ;
#29634=CARTESIAN_POINT ( 'NONE',  ( 93.82876352523145158, 0.000000000000000000, -6.109999999999998543 ) ) ;
#29665=ORIENTED_EDGE ( 'NONE', *, *, #111905, .F. ) ;
#29718=CARTESIAN_POINT ( 'NONE',  ( 88.57876352523145158, -7.482591942790327058E-16, 6.109999999999999432 ) ) ;
#29737=ORIENTED_EDGE ( 'NONE', *, *, #125407, .T. ) ;
#29746=CARTESIAN_POINT ( 'NONE',  ( 10.32500000000000107, -8.432637487761466488, 4.375000000000001776 ) ) ;
#29769=VERTEX_POINT ( 'NONE', #51354 ) ;
#29771=CARTESIAN_POINT ( 'NONE',  ( 110.9583333333333286, 3.974999999999997424, 6.884901960086288852 ) ) ;
#29788=CARTESIAN_POINT ( 'NONE',  ( 104.1254301918981184, 5.291415217122919401, 3.055000000000002824 ) ) ;
#29805=CARTESIAN_POINT ( 'NONE',  ( 126.0004301918981042, -3.055000000000002380, 5.291415217122920289 ) ) ;
#29814=CARTESIAN_POINT ( 'NONE',  ( 126.4954301918981230, 5.291415217122916737, 3.055000000000001936 ) ) ;
#29824=CARTESIAN_POINT ( 'NONE',  ( 49.58376352523144703, -6.110000000000001208, -3.741295971395164515E-16 ) ) ;
#29831=CARTESIAN_POINT ( 'NONE',  ( 42.20376352523144448, 6.109999999999998543, 1.122388791418548911E-15 ) ) ;
#29862=CARTESIAN_POINT ( 'NONE',  ( 59.26626352523145869, 4.472830434245838482, -4.472830434245837594 ) ) ;
#29885=DIRECTION ( 'NONE',  ( -1.000000000000000000, -0.000000000000000000, -0.000000000000000000 ) ) ;
#29886=CARTESIAN_POINT ( 'NONE',  ( 54.18336038379622721, -2.130196079827426203, 7.949999999999996625 ) ) ;
#29898=CARTESIAN_POINT ( 'NONE',  ( 118.1829301918981372, -1.637169565754159173, -6.109999999999999432 ) ) ;
#29939=CARTESIAN_POINT ( 'NONE',  ( 35.49543019189811588, 5.291415217122917625, 3.055000000000002380 ) ) ;
#29966=CARTESIAN_POINT ( 'NONE',  ( 55.49586038379622721, -3.974999999999998312, -6.884901960086286188 ) ) ;
#29972=CARTESIAN_POINT ( 'NONE',  ( 56.41666666666665719, -6.884901960086287076, -3.975000000000000977 ) ) ;
#29979=CARTESIAN_POINT ( 'NONE',  ( 127.0544956184052552, -3.708120683632985859, -5.191463943825122662 ) ) ;
#29982=CARTESIAN_POINT ( 'NONE',  ( 46.66709685856476852, -3.055000000000000160, -5.291415217122921177 ) ) ;
#30007=CARTESIAN_POINT ( 'NONE',  ( 67.57876352523145158, -7.482591942790325086E-16, 6.109999999999998543 ) ) ;
#30019=CARTESIAN_POINT ( 'NONE',  ( 64.00000000000000000, 0.000000000000000000, -7.950000000000000178 ) ) ;
#30026=CARTESIAN_POINT ( 'NONE',  ( 40.03752705046288440, -9.735942053221456900E-16, 7.949999999999998401 ) ) ;
#30035=CARTESIAN_POINT ( 'NONE',  ( 81.57876352523143737, -7.482591942790325086E-16, 6.109999999999998543 ) ) ;
#30061=CARTESIAN_POINT ( 'NONE',  ( 36.60459685856475431, 1.637169565754164946, -6.109999999999999432 ) ) ;
#30117=CARTESIAN_POINT ( 'NONE',  ( 64.37043019189810877, -3.055000000000001936, 5.291415217122918513 ) ) ;
#30143=CARTESIAN_POINT ( 'NONE',  ( 97.35002705046287019, -5.819803920172572198, -5.819803920172572198 ) ) ;
#30148=DIRECTION ( 'NONE',  ( -1.000000000000000000, -0.000000000000000000, -0.000000000000000000 ) ) ;
#30158=CARTESIAN_POINT ( 'NONE',  ( 75.83376352523144703, 6.110000000000001208, 1.122388791418549305E-15 ) ) ;
#30162=ORIENTED_EDGE ( 'NONE', *, *, #32571, .F. ) ;
#30180=CARTESIAN_POINT ( 'NONE',  ( 72.04209685856477563, 5.291415217122923842, -3.054999999999996163 ) ) ;
#30226=CARTESIAN_POINT ( 'NONE',  ( 58.70419371712954870, -6.884901960086285300, -3.975000000000000089 ) ) ;
#30233=CARTESIAN_POINT ( 'NONE',  ( 51.16666666666666430, 6.884901960086285300, 3.975000000000003642 ) ) ;
#30239=CARTESIAN_POINT ( 'NONE',  ( 61.25043019189810423, 3.055000000000002824, -5.291415217122919401 ) ) ;
#30246=CARTESIAN_POINT ( 'NONE',  ( 95.22959685856476142, -6.110000000000000320, -1.637169565754161393 ) ) ;
#30297=CARTESIAN_POINT ( 'NONE',  ( 26.83376352523143993, 6.110000000000001208, 1.122388791418549305E-15 ) ) ;
#30319=CARTESIAN_POINT ( 'NONE',  ( 118.4958603837962272, -3.974999999999998312, -6.884901960086286188 ) ) ;
#30320=CARTESIAN_POINT ( 'NONE',  ( 49.80836038379622721, 7.949999999999996625, 2.130196079827431088 ) ) ;
#30323=CARTESIAN_POINT ( 'NONE',  ( 153.6500000000000057, 4.749999999999997335, 0.000000000000000000 ) ) ;
#30334=EDGE_CURVE ( 'NONE', #55557, #14445, #51724, .T. ) ;
#30343=CARTESIAN_POINT ( 'NONE',  ( 92.43749999999998579, 5.819803920172574863, -5.819803920172573086 ) ) ;
#30347=ORIENTED_EDGE ( 'NONE', *, *, #28374, .T. ) ;
#30357=CARTESIAN_POINT ( 'NONE',  ( 101.6462635252314186, -4.472830434245840259, 4.472830434245839371 ) ) ;
#30367=CARTESIAN_POINT ( 'NONE',  ( 94.41209685856478018, 5.291415217122921177, -3.054999999999994831 ) ) ;
#30432=CARTESIAN_POINT ( 'NONE',  ( 126.1462635252314186, -4.472830434245840259, 4.472830434245838482 ) ) ;
#30463=CARTESIAN_POINT ( 'NONE',  ( 87.70376352523146579, 6.109999999999999432, 1.122388791418549108E-15 ) ) ;
#30464=CARTESIAN_POINT ( 'NONE',  ( 74.50000000000000000, 0.000000000000000000, -7.950000000000000178 ) ) ;
#30492=AXIS2_PLACEMENT_3D ( 'NONE', #140400, #93330, #40401 ) ;
#30521=CARTESIAN_POINT ( 'NONE',  ( 110.0833333333333428, 6.884901960086290629, -3.974999999999994316 ) ) ;
#30535=CARTESIAN_POINT ( 'NONE',  ( 99.75043019189810423, 3.055000000000002824, -5.291415217122919401 ) ) ;
#30548=CARTESIAN_POINT ( 'NONE',  ( 30.16666666666666075, 6.884901960086285300, 3.975000000000003642 ) ) ;
#30559=CARTESIAN_POINT ( 'NONE',  ( 121.5370968585647802, -3.054999999999998828, -5.291415217122919401 ) ) ;
#30565=CARTESIAN_POINT ( 'NONE',  ( 71.10002705046289861, 5.819803920172570422, 5.819803920172575751 ) ) ;
#30571=CARTESIAN_POINT ( 'NONE',  ( 42.00043019189809712, -3.055000000000002380, 5.291415217122920289 ) ) ;
#30579=CARTESIAN_POINT ( 'NONE',  ( 41.76626352523145158, 4.472830434245839371, -4.472830434245838482 ) ) ;
#30616=CARTESIAN_POINT ( 'NONE',  ( 56.78709685856478728, 3.054999999999997495, 5.291415217122919401 ) ) ;
#30649=CARTESIAN_POINT ( 'NONE',  ( 120.5162635252314374, -4.472830434245839371, 4.472830434245839371 ) ) ;
#30692=CARTESIAN_POINT ( 'NONE',  ( 41.47459685856477307, 1.637169565754164280, -6.109999999999997655 ) ) ;
#30721=CARTESIAN_POINT ( 'NONE',  ( 53.74586038379622011, 3.974999999999996980, 6.884901960086287964 ) ) ;
#30726=CARTESIAN_POINT ( 'NONE',  ( 56.27083333333332860, -7.949999999999999289, -2.130196079827426203 ) ) ;
#30733=CARTESIAN_POINT ( 'NONE',  ( 51.18793019189810423, 6.110000000000002984, -1.637169565754156730 ) ) ;
#30749=CARTESIAN_POINT ( 'NONE',  ( 85.16709685856477563, -3.055000000000000160, -5.291415217122921177 ) ) ;
#30755=CARTESIAN_POINT ( 'NONE',  ( 66.70376352523143737, 6.109999999999998543, 1.122388791418548911E-15 ) ) ;
#30787=CARTESIAN_POINT ( 'NONE',  ( 82.59959685856476597, -6.109999999999997655, -1.637169565754160283 ) ) ;
#30815=CARTESIAN_POINT ( 'NONE',  ( 37.18793019189810423, 6.110000000000002984, -1.637169565754156730 ) ) ;
#30866=CARTESIAN_POINT ( 'NONE',  ( 66.55793019189812298, 6.110000000000001208, -1.637169565754156286 ) ) ;
#30890=CARTESIAN_POINT ( 'NONE',  ( 80.57919371712955581, 3.975000000000002753, -6.884901960086283523 ) ) ;
#30904=CARTESIAN_POINT ( 'NONE',  ( 72.62543019189810423, 5.291415217122919401, 3.055000000000002824 ) ) ;
#30923=CARTESIAN_POINT ( 'NONE',  ( 60.95876352523143993, 0.000000000000000000, -6.110000000000001208 ) ) ;
#30926=CARTESIAN_POINT ( 'NONE',  ( 0.000000000000000000, 0.000000000000000000, 0.000000000000000000 ) ) ;
#30951=CARTESIAN_POINT ( 'NONE',  ( 62.25000000000000000, -9.735942053221458872E-16, 7.950000000000000178 ) ) ;
#30965=( BOUNDED_CURVE ( )  B_SPLINE_CURVE ( 2, ( #126438, #29979, #115530, #38735, #118413 ),
 .UNSPECIFIED., .F., .F. ) 
 B_SPLINE_CURVE_WITH_KNOTS ( ( 3, 2, 3 ),
 ( 0.9711948811556444516, 0.9722222222222222099, 0.9749999999999999778 ),
 .UNSPECIFIED. ) 
 CURVE ( )  GEOMETRIC_REPRESENTATION_ITEM ( )  RATIONAL_B_SPLINE_CURVE ( ( 0.9841174075436982527, 0.9873979127333399886, 1.000000000000000000, 0.9659258262890683122, 1.000000000000000000 ) ) 
 REPRESENTATION_ITEM ( '' )  );
#30975=VERTEX_POINT ( 'NONE', #26052 ) ;
#30984=CARTESIAN_POINT ( 'NONE',  ( 61.68793019189811844, 6.110000000000002984, -1.637169565754156730 ) ) ;
#30992=CARTESIAN_POINT ( 'NONE',  ( 96.97959685856477563, 6.109999999999999432, 1.637169565754164280 ) ) ;
#31000=CARTESIAN_POINT ( 'NONE',  ( 90.39583333333335702, -2.130196079827389344, 7.950000000000021494 ) ) ;
#31006=VERTEX_POINT ( 'NONE', #70314 ) ;
#31007=CARTESIAN_POINT ( 'NONE',  ( 118.4745968585647944, 1.637169565754164280, -6.109999999999996767 ) ) ;
#31020=CARTESIAN_POINT ( 'NONE',  ( 38.62499999999999289, -7.950000000000000178, -4.867971026610729436E-16 ) ) ;
#31021=ORIENTED_EDGE ( 'NONE', *, *, #30334, .F. ) ;
#31032=CARTESIAN_POINT ( 'NONE',  ( 29.89626352523142927, 4.472830434245840259, -4.472830434245839371 ) ) ;
#31055=CARTESIAN_POINT ( 'NONE',  ( 109.3083603837961988, 7.949999999999997513, 2.130196079827431088 ) ) ;
#31056=CARTESIAN_POINT ( 'NONE',  ( 49.66252705046289861, 7.949999999999998401, 1.460391307983218338E-15 ) ) ;
#31060=DIRECTION ( 'NONE',  ( 0.000000000000000000, 0.000000000000000000, -1.000000000000000000 ) ) ;
#31085=ADVANCED_FACE ( 'NONE', ( #130368, #18704 ), #8519, .F. ) ;
#31093=CARTESIAN_POINT ( 'NONE',  ( 102.6670968585647756, -3.055000000000000160, -5.291415217122921177 ) ) ;
#31103=CARTESIAN_POINT ( 'NONE',  ( 99.95376352523145158, -6.109999999999998543, -3.741295971395162543E-16 ) ) ;
#31108=CARTESIAN_POINT ( 'NONE',  ( 115.1874999999999858, -5.819803920172573974, 5.819803920172573086 ) ) ;
#31134=CARTESIAN_POINT ( 'NONE',  ( 55.68749999999999289, -5.819803920172573974, 5.819803920172573086 ) ) ;
#31152=( BOUNDED_CURVE ( )  B_SPLINE_CURVE ( 2, ( #79676, #1316, #55740, #69480, #58644, #101363, #123144, #57899, #78932, #68767, #133307, #45597, #99945 ),
 .UNSPECIFIED., .F., .T. ) 
 B_SPLINE_CURVE_WITH_KNOTS ( ( 3, 2, 2, 2, 2, 2, 3 ),
 ( 0.6833333333333333481, 0.6861111111111111160, 0.6888888888888888840, 0.6916666666666666519, 0.6944444444444444198, 0.6972222222222221877, 0.6999999999999999556 ),
 .UNSPECIFIED. ) 
 CURVE ( )  GEOMETRIC_REPRESENTATION_ITEM ( )  RATIONAL_B_SPLINE_CURVE ( ( 1.000000000000000000, 0.9659258262890683122, 1.000000000000000000, 0.9659258262890683122, 1.000000000000000000, 0.9659258262890683122, 1.000000000000000000, 0.9659258262890683122, 1.000000000000000000, 0.9659258262890683122, 1.000000000000000000, 0.9659258262890683122, 1.000000000000000000 ) ) 
 REPRESENTATION_ITEM ( '' )  );
#31153=ORIENTED_EDGE ( 'NONE', *, *, #66417, .T. ) ;
#31155=CARTESIAN_POINT ( 'NONE',  ( 28.05793019189811233, 6.110000000000000320, -1.637169565754156064 ) ) ;
#31185=CARTESIAN_POINT ( 'NONE',  ( 93.68293019189812298, -1.637169565754159173, -6.109999999999999432 ) ) ;
#31186=CARTESIAN_POINT ( 'NONE',  ( 8.900575677527392315, -8.548178872310858267, -4.146506754080105495 ) ) ;
#31201=CARTESIAN_POINT ( 'NONE',  ( 0.000000000000000000, 0.000000000000000000, 0.000000000000000000 ) ) ;
#31223=CARTESIAN_POINT ( 'NONE',  ( 31.18749999999998934, -5.819803920172573974, 5.819803920172573086 ) ) ;
#31237=CARTESIAN_POINT ( 'NONE',  ( 114.0208333333333144, 7.949999999999999289, 2.130196079827431532 ) ) ;
#31250=CARTESIAN_POINT ( 'NONE',  ( 104.4170968585647756, 3.054999999999998828, 5.291415217122922066 ) ) ;
#31259=CARTESIAN_POINT ( 'NONE',  ( 29.97502705046288796, -5.819803920172572198, 5.819803920172572198 ) ) ;
#31265=CARTESIAN_POINT ( 'NONE',  ( 27.39583333333332149, -2.130196079827427091, 7.949999999999999289 ) ) ;
#31274=CARTESIAN_POINT ( 'NONE',  ( 123.7245968585647660, -1.637169565754160949, 6.109999999999997655 ) ) ;
#31286=CARTESIAN_POINT ( 'NONE',  ( 47.83376352523143993, 6.110000000000001208, 1.122388791418549305E-15 ) ) ;
#31292=CARTESIAN_POINT ( 'NONE',  ( 35.93293019189811588, 1.637169565754156508, 6.110000000000000320 ) ) ;
#31317=CARTESIAN_POINT ( 'NONE',  ( 54.16209685856478018, -5.291415217122919401, 3.054999999999997939 ) ) ;
#31353=CYLINDRICAL_SURFACE ( 'NONE', #60043, 7.950000000000000178 ) ;
#31355=CARTESIAN_POINT ( 'NONE',  ( 118.9120968585647802, 5.291415217122922066, -3.054999999999995275 ) ) ;
#31360=CARTESIAN_POINT ( 'NONE',  ( 67.74586038379622721, 3.974999999999996980, 6.884901960086287964 ) ) ;
#31378=CARTESIAN_POINT ( 'NONE',  ( 125.5000000000000000, 0.000000000000000000, 0.000000000000000000 ) ) ;
#31389=CARTESIAN_POINT ( 'NONE',  ( 126.6604541630265999, -6.146688740034715437, -2.899546345087764543 ) ) ;
#31391=CARTESIAN_POINT ( 'NONE',  ( 40.01626352523144448, -4.472830434245839371, 4.472830434245839371 ) ) ;
#31403=( BOUNDED_CURVE ( )  B_SPLINE_CURVE ( 2, ( #79183, #80590, #841, #56726, #46567, #21898, #100887, #1540, #99438, #90754, #45129, #35682, #89307 ),
 .UNSPECIFIED., .F., .T. ) 
 B_SPLINE_CURVE_WITH_KNOTS ( ( 3, 2, 2, 2, 2, 2, 3 ),
 ( 0.05000000000000004441, 0.05277777777777781926, 0.05555555555555560104, 0.05833333333333338283, 0.06111111111111115768, 0.06388888888888893947, 0.06666666666666672125 ),
 .UNSPECIFIED. ) 
 CURVE ( )  GEOMETRIC_REPRESENTATION_ITEM ( )  RATIONAL_B_SPLINE_CURVE ( ( 0.9999999999999994449, 0.9659258262890688673, 1.000000000000000000, 0.9659258262890683122, 1.000000000000000000, 0.9659258262890683122, 1.000000000000000000, 0.9659258262890683122, 1.000000000000000000, 0.9659258262890683122, 1.000000000000000000, 0.9659258262890676461, 1.000000000000000666 ) ) 
 REPRESENTATION_ITEM ( '' )  );
#31410=FACE_OUTER_BOUND ( 'NONE', #33600, .T. ) ;
#31414=CARTESIAN_POINT ( 'NONE',  ( 79.31250000000000000, 5.819803920172571310, 5.819803920172576639 ) ) ;
#31420=CARTESIAN_POINT ( 'NONE',  ( 52.28752705046288440, 0.000000000000000000, -7.949999999999998401 ) ) ;
#31425=CARTESIAN_POINT ( 'NONE',  ( 53.35416666666666430, -2.130196079827425315, -7.950000000000001066 ) ) ;
#31433=CARTESIAN_POINT ( 'NONE',  ( 43.16709685856477563, -3.055000000000000160, -5.291415217122921177 ) ) ;
#31435=EDGE_CURVE ( 'NONE', #91561, #128706, #29430, .T. ) ;
#31447=CARTESIAN_POINT ( 'NONE',  ( 81.37543019189810423, -5.291415217122920289, -3.055000000000001492 ) ) ;
#31458=CARTESIAN_POINT ( 'NONE',  ( 70.20376352523143737, 6.109999999999998543, 1.122388791418548911E-15 ) ) ;
#31481=CARTESIAN_POINT ( 'NONE',  ( 50.82919371712955581, -3.975000000000001865, 6.884901960086284411 ) ) ;
#31487=CARTESIAN_POINT ( 'NONE',  ( 86.24543019189812298, -5.291415217122918513, -3.055000000000000160 ) ) ;
#31504=CARTESIAN_POINT ( 'NONE',  ( 122.4333603837967530, 2.130196079833805989, -7.949999999996317790 ) ) ;
#31510=CARTESIAN_POINT ( 'NONE',  ( 35.87543019189811133, -5.291415217122920289, -3.055000000000001492 ) ) ;
#31532=CARTESIAN_POINT ( 'NONE',  ( 109.0166937171295416, 7.950000000000000178, -2.130196079827421318 ) ) ;
#31549=AXIS2_PLACEMENT_3D ( 'NONE', #36594, #80846, #126452 ) ;
#31556=CARTESIAN_POINT ( 'NONE',  ( 0.000000000000000000, 0.000000000000000000, 7.950000000000000178 ) ) ;
#31567=CARTESIAN_POINT ( 'NONE',  ( 63.78709685856477307, 3.054999999999997939, 5.291415217122920289 ) ) ;
#31577=ORIENTED_EDGE ( 'NONE', *, *, #49407, .T. ) ;
#31583=EDGE_CURVE ( 'NONE', #66284, #74755, #116454, .T. ) ;
#31593=CARTESIAN_POINT ( 'NONE',  ( 85.39169371712957002, 2.130196079827421762, 7.950000000000001066 ) ) ;
#31606=CARTESIAN_POINT ( 'NONE',  ( 75.25043019189811844, 3.055000000000002824, -5.291415217122919401 ) ) ;
#31608=ADVANCED_FACE ( 'NONE', ( #1763 ), #78669, .T. ) ;
#31626=CARTESIAN_POINT ( 'NONE',  ( 67.52126352523141861, -4.472830434245839371, -4.472830434245840259 ) ) ;
#31658=CARTESIAN_POINT ( 'NONE',  ( 108.8495968585647660, 6.109999999999996767, 1.637169565754163836 ) ) ;
#31682=CARTESIAN_POINT ( 'NONE',  ( 59.64626352523142572, -4.472830434245840259, 4.472830434245838482 ) ) ;
#31686=CARTESIAN_POINT ( 'NONE',  ( 100.1879301918981184, 6.110000000000002984, -1.637169565754156730 ) ) ;
#31688=CARTESIAN_POINT ( 'NONE',  ( 51.74999999999999289, -9.735942053221458872E-16, 7.950000000000000178 ) ) ;
#31701=CARTESIAN_POINT ( 'NONE',  ( 117.4537635252314516, -6.109999999999998543, -3.741295971395162543E-16 ) ) ;
#31729=CARTESIAN_POINT ( 'NONE',  ( 28.00043019189810067, -3.055000000000002380, 5.291415217122920289 ) ) ;
#31753=CARTESIAN_POINT ( 'NONE',  ( 108.4333603837962272, 2.130196079827431532, -7.949999999999997513 ) ) ;
#31754=CARTESIAN_POINT ( 'NONE',  ( 49.95419371712955581, 6.884901960086283523, 3.975000000000002753 ) ) ;
#31764=CYLINDRICAL_SURFACE ( 'NONE', #35095, 7.950000000000000178 ) ;
#31792=ORIENTED_EDGE ( 'NONE', *, *, #99454, .F. ) ;
#31793=CARTESIAN_POINT ( 'NONE',  ( 95.66709685856477563, -3.055000000000000160, -5.291415217122921177 ) ) ;
#31804=CARTESIAN_POINT ( 'NONE',  ( 92.07876352523145158, -7.482591942790325086E-16, 6.109999999999998543 ) ) ;
#31807=CARTESIAN_POINT ( 'NONE',  ( 117.0375270504628986, -9.735942053221456900E-16, 7.949999999999998401 ) ) ;
#31812=CARTESIAN_POINT ( 'NONE',  ( 60.50000000000000000, 0.000000000000000000, -7.950000000000000178 ) ) ;
#31827=CARTESIAN_POINT ( 'NONE',  ( 81.49999999999998579, 0.000000000000000000, -7.950000000000000178 ) ) ;
#31886=CARTESIAN_POINT ( 'NONE',  ( 94.70376352523145158, 6.109999999999999432, 1.122388791418549108E-15 ) ) ;
#31937=CARTESIAN_POINT ( 'NONE',  ( 97.83333333333332860, -6.884901960086287964, 3.974999999999998312 ) ) ;
#31958=CARTESIAN_POINT ( 'NONE',  ( 32.16252705046289151, 7.949999999999998401, 1.460391307983218338E-15 ) ) ;
#31964=CARTESIAN_POINT ( 'NONE',  ( 124.3962635252314470, 4.472830434245840259, -4.472830434245839371 ) ) ;
#31972=CARTESIAN_POINT ( 'NONE',  ( 118.7662635252314516, 4.472830434245839371, -4.472830434245838482 ) ) ;
#31979=CARTESIAN_POINT ( 'NONE',  ( 43.89626352523143282, 4.472830434245840259, -4.472830434245839371 ) ) ;
#31987=CARTESIAN_POINT ( 'NONE',  ( 42.93293019189812298, 1.637169565754156508, 6.110000000000000320 ) ) ;
#31998=ORIENTED_EDGE ( 'NONE', *, *, #87360, .F. ) ;
#32018=CARTESIAN_POINT ( 'NONE',  ( 47.74543019189811588, -5.291415217122918513, -3.055000000000000160 ) ) ;
#32058=CARTESIAN_POINT ( 'NONE',  ( 122.8495968585647518, 6.109999999999997655, 1.637169565754163836 ) ) ;
#32075=VERTEX_POINT ( 'NONE', #130755 ) ;
#32092=CARTESIAN_POINT ( 'NONE',  ( 124.0375270504628986, -9.735942053221456900E-16, 7.949999999999998401 ) ) ;
#32100=CARTESIAN_POINT ( 'NONE',  ( 39.14126352523145869, 4.472830434245837594, 4.472830434245841147 ) ) ;
#32104=CARTESIAN_POINT ( 'NONE',  ( 126.7083333333333428, -3.974999999999999201, -6.884901960086287964 ) ) ;
#32124=CARTESIAN_POINT ( 'NONE',  ( 56.07919371712956291, 3.975000000000002753, -6.884901960086283523 ) ) ;
#32129=CARTESIAN_POINT ( 'NONE',  ( 59.47916666666666430, -7.950000000000001066, 2.130196079827424427 ) ) ;
#32138=CARTESIAN_POINT ( 'NONE',  ( 47.54209685856476852, 5.291415217122923842, -3.054999999999996163 ) ) ;
#32147=CARTESIAN_POINT ( 'NONE',  ( 81.74586038379622721, 3.974999999999996980, 6.884901960086287964 ) ) ;
#32155=CARTESIAN_POINT ( 'NONE',  ( 79.04209685856477563, 5.291415217122923842, -3.054999999999996163 ) ) ;
#32163=CARTESIAN_POINT ( 'NONE',  ( 69.62043019189812298, 3.055000000000001936, -5.291415217122916737 ) ) ;
#32172=CYLINDRICAL_SURFACE ( 'NONE', #79322, 7.950000000000000178 ) ;
#32174=ORIENTED_EDGE ( 'NONE', *, *, #105058, .T. ) ;
#32190=CARTESIAN_POINT ( 'NONE',  ( 51.55836038379622011, -7.949999999999996625, -2.130196079827426203 ) ) ;
#32199=CARTESIAN_POINT ( 'NONE',  ( 87.12043019189812298, 3.055000000000001936, -5.291415217122916737 ) ) ;
#32213=DIRECTION ( 'NONE',  ( 0.000000000000000000, 0.000000000000000000, 1.000000000000000000 ) ) ;
#32216=ORIENTED_EDGE ( 'NONE', *, *, #121014, .T. ) ;
#32219=CARTESIAN_POINT ( 'NONE',  ( 124.0375270504628986, -9.735942053221456900E-16, 7.949999999999998401 ) ) ;
#32224=CARTESIAN_POINT ( 'NONE',  ( 34.56293019189809712, 1.637169565754157174, 6.110000000000002984 ) ) ;
#32228=CARTESIAN_POINT ( 'NONE',  ( 90.35002705046288440, -5.819803920172573086, -5.819803920172573086 ) ) ;
#32232=CARTESIAN_POINT ( 'NONE',  ( 0.000000000000000000, 0.000000000000000000, 0.000000000000000000 ) ) ;
#32236=CARTESIAN_POINT ( 'NONE',  ( 0.000000000000000000, 7.776507174585692163E-16, -6.349999999999999645 ) ) ;
#32257=FACE_OUTER_BOUND ( 'NONE', #5173, .T. ) ;
#32261=ORIENTED_EDGE ( 'NONE', *, *, #92935, .T. ) ;
#32263=ORIENTED_EDGE ( 'NONE', *, *, #118281, .F. ) ;
#32282=CARTESIAN_POINT ( 'NONE',  ( 68.59959685856476597, -6.109999999999998543, -1.637169565754160727 ) ) ;
#32311=CARTESIAN_POINT ( 'NONE',  ( 83.05836038379621300, -7.949999999999997513, -2.130196079827425759 ) ) ;
#32315=CARTESIAN_POINT ( 'NONE',  ( 83.54166666666667140, -3.975000000000002753, 6.884901960086286188 ) ) ;
#32318=CARTESIAN_POINT ( 'NONE',  ( 78.53752705046289861, -9.735942053221456900E-16, 7.949999999999998401 ) ) ;
#32324=CARTESIAN_POINT ( 'NONE',  ( 74.81293019189809002, -1.637169565754159617, -6.110000000000001208 ) ) ;
#32341=CARTESIAN_POINT ( 'NONE',  ( 65.77126352523144703, 4.472830434245839371, 4.472830434245842035 ) ) ;
#32345=LINE ( 'NONE', #96142, #24911 ) ;
#32363=CARTESIAN_POINT ( 'NONE',  ( 61.08333333333332149, 6.884901960086290629, -3.974999999999994316 ) ) ;
#32372=CARTESIAN_POINT ( 'NONE',  ( 108.2662635252314374, 4.472830434245838482, -4.472830434245837594 ) ) ;
#32378=ADVANCED_FACE ( 'NONE', ( #141237 ), #53535, .T. ) ;
#32403=CARTESIAN_POINT ( 'NONE',  ( 63.43793019189811133, -6.110000000000001208, 1.637169565754158951 ) ) ;
#32409=CARTESIAN_POINT ( 'NONE',  ( 95.37543019189810423, -5.291415217122920289, -3.055000000000001492 ) ) ;
#32416=CARTESIAN_POINT ( 'NONE',  ( 91.70833333333334281, -3.974999999999999201, -6.884901960086287964 ) ) ;
#32424=CARTESIAN_POINT ( 'NONE',  ( 121.6829301918981088, -1.637169565754158951, -6.109999999999998543 ) ) ;
#32443=CARTESIAN_POINT ( 'NONE',  ( 58.75000000000000000, -9.735942053221458872E-16, 7.950000000000000178 ) ) ;
#32447=DIRECTION ( 'NONE',  ( 1.000000000000000000, 0.000000000000000000, 0.000000000000000000 ) ) ;
#32448=CARTESIAN_POINT ( 'NONE',  ( 28.43793019189810423, -6.110000000000001208, 1.637169565754158951 ) ) ;
#32463=CARTESIAN_POINT ( 'NONE',  ( 42.70833333333333570, -3.974999999999999201, -6.884901960086287964 ) ) ;
#32472=ORIENTED_EDGE ( 'NONE', *, *, #112897, .F. ) ;
#32474=CARTESIAN_POINT ( 'NONE',  ( 108.2875270504628986, 0.000000000000000000, -7.949999999999998401 ) ) ;
#32515=CARTESIAN_POINT ( 'NONE',  ( 97.12543019189810423, 5.291415217122919401, 3.055000000000002824 ) ) ;
#32524=CARTESIAN_POINT ( 'NONE',  ( 49.56249999999999289, -5.819803920172573086, -5.819803920172573974 ) ) ;
#32525=CARTESIAN_POINT ( 'NONE',  ( 90.47459685856479439, 1.637169565754164058, -6.109999999999996767 ) ) ;
#32571=EDGE_CURVE ( 'NONE', #94004, #24699, #25899, .T. ) ;
#32582=CARTESIAN_POINT ( 'NONE',  ( 123.5212635252314470, -4.472830434245838482, -4.472830434245840259 ) ) ;
#32618=CARTESIAN_POINT ( 'NONE',  ( 89.59959685856475176, -6.109999999999998543, -1.637169565754160727 ) ) ;
#32619=CARTESIAN_POINT ( 'NONE',  ( 6.849737334536333044, -9.119535513348605349, -2.672630034853287206 ) ) ;
#32651=CARTESIAN_POINT ( 'NONE',  ( 32.20833333333332149, -3.974999999999999201, -6.884901960086287964 ) ) ;
#32665=CARTESIAN_POINT ( 'NONE',  ( 99.87499999999998579, 7.950000000000000178, 1.460391307983218535E-15 ) ) ;
#32696=CARTESIAN_POINT ( 'NONE',  ( 118.8545968585647898, -1.637169565754161615, 6.110000000000000320 ) ) ;
#32708=CARTESIAN_POINT ( 'NONE',  ( 115.5579301918981088, 6.110000000000000320, -1.637169565754156064 ) ) ;
#32718=CARTESIAN_POINT ( 'NONE',  ( 40.10459685856476142, 1.637169565754164946, -6.109999999999999432 ) ) ;
#32724=CARTESIAN_POINT ( 'NONE',  ( 39.87043019189810877, -3.055000000000001492, 5.291415217122917625 ) ) ;
#32744=CARTESIAN_POINT ( 'NONE',  ( 0.000000000000000000, 0.000000000000000000, 0.000000000000000000 ) ) ;
#32755=CARTESIAN_POINT ( 'NONE',  ( 48.18293019189812298, -1.637169565754158951, -6.109999999999998543 ) ) ;
#32773=ORIENTED_EDGE ( 'NONE', *, *, #91067, .T. ) ;
#32797=CARTESIAN_POINT ( 'NONE',  ( 117.4537635252314516, -6.109999999999999432, -3.741295971395163529E-16 ) ) ;
#32830=VERTEX_POINT ( 'NONE', #89685 ) ;
#32839=CARTESIAN_POINT ( 'NONE',  ( 41.32876352523144448, 0.000000000000000000, -6.109999999999999432 ) ) ;
#32853=EDGE_CURVE ( 'NONE', #31006, #2581, #34601, .T. ) ;
#32856=CARTESIAN_POINT ( 'NONE',  ( 124.8337635252314470, 6.110000000000001208, 1.122388791418549305E-15 ) ) ;
#32867=CARTESIAN_POINT ( 'NONE',  ( 54.32919371712956291, -3.975000000000001865, 6.884901960086284411 ) ) ;
#32873=CARTESIAN_POINT ( 'NONE',  ( 47.52083333333332860, 7.949999999999999289, 2.130196079827431532 ) ) ;
#32880=CARTESIAN_POINT ( 'NONE',  ( 127.0000000000000000, -4.071459123471990793, -4.960746789751230068 ) ) ;
#32885=CARTESIAN_POINT ( 'NONE',  ( 44.18793019189810423, 6.110000000000002984, -1.637169565754156730 ) ) ;
#32902=CARTESIAN_POINT ( 'NONE',  ( 81.22959685856476142, -6.110000000000000320, -1.637169565754161393 ) ) ;
#32910=CARTESIAN_POINT ( 'NONE',  ( 65.39126352523145158, -4.472830434245839371, -4.472830434245839371 ) ) ;
#32933=CARTESIAN_POINT ( 'NONE',  ( 40.76669371712956291, -7.949999999999998401, 2.130196079827423983 ) ) ;
#32935=CARTESIAN_POINT ( 'NONE',  ( 51.12086038379622011, -6.884901960086286188, 3.974999999999997424 ) ) ;
#32942=CARTESIAN_POINT ( 'NONE',  ( 75.74543019189810877, -5.291415217122918513, -3.055000000000000160 ) ) ;
#32968=CARTESIAN_POINT ( 'NONE',  ( 26.54209685856477563, 5.291415217122923842, -3.054999999999996163 ) ) ;
#32987=CARTESIAN_POINT ( 'NONE',  ( 115.2875270504628986, 0.000000000000000000, -7.949999999999998401 ) ) ;
#33008=CARTESIAN_POINT ( 'NONE',  ( 97.35002705046287019, -5.819803920172573086, -5.819803920172573086 ) ) ;
#33022=CARTESIAN_POINT ( 'NONE',  ( 52.04166666666666430, -3.975000000000002753, 6.884901960086286188 ) ) ;
#33024=CARTESIAN_POINT ( 'NONE',  ( 67.57876352523145158, -7.482591942790327058E-16, 6.109999999999999432 ) ) ;
#33028=CARTESIAN_POINT ( 'NONE',  ( 33.03752705046289151, -9.735942053221456900E-16, 7.949999999999998401 ) ) ;
#33054=CARTESIAN_POINT ( 'NONE',  ( 82.62086038379624142, -6.884901960086286188, 3.974999999999997424 ) ) ;
#33060=CARTESIAN_POINT ( 'NONE',  ( 76.83333333333334281, -6.884901960086287964, 3.974999999999998312 ) ) ;
#33073=CARTESIAN_POINT ( 'NONE',  ( 79.18793019189810423, 6.110000000000002984, -1.637169565754156730 ) ) ;
#33090=CARTESIAN_POINT ( 'NONE',  ( 64.45876352523144703, 0.000000000000000000, -6.110000000000001208 ) ) ;
#33117=CARTESIAN_POINT ( 'NONE',  ( 127.5761022459138161, -4.648522628062369932, 4.648522628062369932 ) ) ;
#33124=CARTESIAN_POINT ( 'NONE',  ( 107.8287635252314516, 0.000000000000000000, -6.109999999999998543 ) ) ;
#33139=CARTESIAN_POINT ( 'NONE',  ( 59.28752705046289151, 0.000000000000000000, -7.949999999999998401 ) ) ;
#33150=CARTESIAN_POINT ( 'NONE',  ( 64.75043019189810423, 3.055000000000002824, -5.291415217122919401 ) ) ;
#33156=CARTESIAN_POINT ( 'NONE',  ( 98.14626352523143282, -4.472830434245840259, 4.472830434245838482 ) ) ;
#33172=CARTESIAN_POINT ( 'NONE',  ( 123.8704301918981230, -3.055000000000001492, 5.291415217122917625 ) ) ;
#33219=CARTESIAN_POINT ( 'NONE',  ( 111.6416937171295558, -2.130196079827424871, -7.949999999999999289 ) ) ;
#33231=DIRECTION ( 'NONE',  ( 0.000000000000000000, 0.000000000000000000, 1.000000000000000000 ) ) ;
#33255=CYLINDRICAL_SURFACE ( 'NONE', #35417, 7.950000000000000178 ) ;
#33265=CARTESIAN_POINT ( 'NONE',  ( 88.81293019189809002, -1.637169565754159617, -6.110000000000001208 ) ) ;
#33271=CARTESIAN_POINT ( 'NONE',  ( 83.78752705046288440, 0.000000000000000000, -7.949999999999998401 ) ) ;
#33275=CARTESIAN_POINT ( 'NONE',  ( 86.53709685856478018, -3.054999999999998828, -5.291415217122919401 ) ) ;
#33304=CARTESIAN_POINT ( 'NONE',  ( 56.41666666666665719, -6.884901960086287076, -3.975000000000000977 ) ) ;
#33323=( BOUNDED_CURVE ( )  B_SPLINE_CURVE ( 2, ( #95018, #94320, #137855, #27630, #127687, #115319, #84880, #72630, #73308 ),
 .UNSPECIFIED., .F., .T. ) 
 B_SPLINE_CURVE_WITH_KNOTS ( ( 3, 2, 2, 2, 3 ),
 ( 0.008333333333333340157, 0.01111111111111109939, 0.01388888888888885689, 0.01666666666666661439, 0.01881059163983938437 ),
 .UNSPECIFIED. ) 
 CURVE ( )  GEOMETRIC_REPRESENTATION_ITEM ( )  RATIONAL_B_SPLINE_CURVE ( ( 0.9999999999999995559, 0.9659258262890687563, 1.000000000000000000, 0.9659258262890683122, 1.000000000000000000, 0.9659258262890683122, 1.000000000000000000, 0.9737011100947261522, 0.9879978699103917350 ) ) 
 REPRESENTATION_ITEM ( '' )  );
#33346=CARTESIAN_POINT ( 'NONE',  ( 107.7041937171295558, -6.884901960086285300, -3.975000000000000089 ) ) ;
#33359=CARTESIAN_POINT ( 'NONE',  ( 81.72459685856476597, -1.637169565754161171, 6.109999999999998543 ) ) ;
#33408=CARTESIAN_POINT ( 'NONE',  ( 99.43749999999998579, 5.819803920172573974, -5.819803920172572198 ) ) ;
#33409=ORIENTED_EDGE ( 'NONE', *, *, #64663, .F. ) ;
#33431=ORIENTED_EDGE ( 'NONE', *, *, #107335, .F. ) ;
#33433=CARTESIAN_POINT ( 'NONE',  ( 120.0212635252314328, -4.472830434245839371, -4.472830434245840259 ) ) ;
#33440=CARTESIAN_POINT ( 'NONE',  ( 116.8704301918981230, -3.055000000000001492, 5.291415217122917625 ) ) ;
#33445=CARTESIAN_POINT ( 'NONE',  ( 70.07919371712955581, 3.975000000000002753, -6.884901960086283523 ) ) ;
#33446=CARTESIAN_POINT ( 'NONE',  ( 98.85416666666665719, -2.130196079827387567, -7.950000000000023270 ) ) ;
#33449=CARTESIAN_POINT ( 'NONE',  ( 39.95876352523143282, 0.000000000000000000, -6.110000000000001208 ) ) ;
#33458=CARTESIAN_POINT ( 'NONE',  ( 32.28709685856477307, 3.054999999999997495, 5.291415217122919401 ) ) ;
#33482=CARTESIAN_POINT ( 'NONE',  ( 47.89126352523143737, -4.472830434245838482, -4.472830434245838482 ) ) ;
#33483=ORIENTED_EDGE ( 'NONE', *, *, #70240, .T. ) ;
#33516=CARTESIAN_POINT ( 'NONE',  ( 107.3912635252314516, -4.472830434245839371, -4.472830434245839371 ) ) ;
#33532=CIRCLE ( 'NONE', #40454, 9.500000000000000000 ) ;
#33537=( BOUNDED_CURVE ( )  B_SPLINE_CURVE ( 2, ( #4214, #2098, #26050, #92003, #89856, #123946, #48507, #134102, #122478, #70313, #13001, #23913, #114462 ),
 .UNSPECIFIED., .F., .T. ) 
 B_SPLINE_CURVE_WITH_KNOTS ( ( 3, 2, 2, 2, 2, 2, 3 ),
 ( 0.7666666666666667185, 0.7694444444444444864, 0.7722222222222222543, 0.7750000000000000222, 0.7777777777777777901, 0.7805555555555555580, 0.7833333333333333259 ),
 .UNSPECIFIED. ) 
 CURVE ( )  GEOMETRIC_REPRESENTATION_ITEM ( )  RATIONAL_B_SPLINE_CURVE ( ( 1.000000000000000000, 0.9659258262890683122, 1.000000000000000000, 0.9659258262890683122, 1.000000000000000000, 0.9659258262890683122, 1.000000000000000000, 0.9659258262890683122, 1.000000000000000000, 0.9659258262890683122, 1.000000000000000000, 0.9659258262890683122, 1.000000000000000000 ) ) 
 REPRESENTATION_ITEM ( '' )  );
#33559=CARTESIAN_POINT ( 'NONE',  ( 30.24543019189811233, -5.291415217122919401, -3.055000000000000604 ) ) ;
#33562=ADVANCED_FACE ( 'NONE', ( #31410 ), #82340, .T. ) ;
#33565=CARTESIAN_POINT ( 'NONE',  ( 125.2500000000000000, -9.735942053221458872E-16, 7.950000000000000178 ) ) ;
#33576=CARTESIAN_POINT ( 'NONE',  ( 122.0629301918981042, 1.637169565754157174, 6.110000000000002984 ) ) ;
#33580=CARTESIAN_POINT ( 'NONE',  ( 78.87500000000000000, 7.950000000000000178, 1.460391307983218535E-15 ) ) ;
#33584=CARTESIAN_POINT ( 'NONE',  ( 47.18336038379622721, -2.130196079827426203, 7.949999999999997513 ) ) ;
#33589=CARTESIAN_POINT ( 'NONE',  ( 45.62500000000000000, -7.950000000000000178, -4.867971026610729436E-16 ) ) ;
#33597=CARTESIAN_POINT ( 'NONE',  ( 41.70876352523143993, -7.482591942790329030E-16, 6.110000000000001208 ) ) ;
#33600=EDGE_LOOP ( 'NONE', ( #1312, #19872, #115860, #79418 ) ) ;
#33610=CARTESIAN_POINT ( 'NONE',  ( 85.02126352523144703, -4.472830434245838482, -4.472830434245840259 ) ) ;
#33614=LINE ( 'NONE', #65543, #104124 ) ;
#33620=CARTESIAN_POINT ( 'NONE',  ( 58.24543019189810877, -5.291415217122918513, -3.055000000000000160 ) ) ;
#33627=FILL_AREA_STYLE_COLOUR ( '', #60746 ) ;
#33631=CARTESIAN_POINT ( 'NONE',  ( 0.000000000000000000, 0.000000000000000000, 7.950000000000000178 ) ) ;
#33649=CARTESIAN_POINT ( 'NONE',  ( 77.49543019189810877, 5.291415217122916737, 3.055000000000001936 ) ) ;
#33673=CARTESIAN_POINT ( 'NONE',  ( 30.33376352523143993, 6.110000000000001208, 1.122388791418549305E-15 ) ) ;
#33708=DIRECTION ( 'NONE',  ( 0.000000000000000000, 0.000000000000000000, 1.000000000000000000 ) ) ;
#33722=CARTESIAN_POINT ( 'NONE',  ( 112.8541666666666714, -2.130196079827406219, -7.950000000000012612 ) ) ;
#33724=CARTESIAN_POINT ( 'NONE',  ( 52.77083333333332149, -7.949999999999998401, -2.130196079827426203 ) ) ;
#33726=CARTESIAN_POINT ( 'NONE',  ( 53.57876352523144448, -7.482591942790327058E-16, 6.109999999999999432 ) ) ;
#33751=CARTESIAN_POINT ( 'NONE',  ( 88.01669371712955581, 7.950000000000001066, -2.130196079827421318 ) ) ;
#33756=CARTESIAN_POINT ( 'NONE',  ( 76.10416666666667140, 2.130196079827422206, 7.950000000000001954 ) ) ;
#33768=CARTESIAN_POINT ( 'NONE',  ( 70.72959685856477563, -6.110000000000000320, -1.637169565754161393 ) ) ;
#33776=CARTESIAN_POINT ( 'NONE',  ( 127.0000000000000000, 1.864289179696898779, 6.174700466780991270 ) ) ;
#33782=VERTEX_POINT ( 'NONE', #70904 ) ;
#33784=CARTESIAN_POINT ( 'NONE',  ( 64.89626352523144703, 4.472830434245840259, -4.472830434245839371 ) ) ;
#33809=CARTESIAN_POINT ( 'NONE',  ( 101.1204301918981230, 3.055000000000001936, -5.291415217122916737 ) ) ;
#33836=CARTESIAN_POINT ( 'NONE',  ( 53.08376352523143282, -6.110000000000001208, -3.741295971395164515E-16 ) ) ;
#33844=CARTESIAN_POINT ( 'NONE',  ( 93.33376352523144703, 6.110000000000001208, 1.122388791418549305E-15 ) ) ;
#33848=VERTEX_POINT ( 'NONE', #141112 ) ;
#33856=VERTEX_POINT ( 'NONE', #65021 ) ;
#33861=CARTESIAN_POINT ( 'NONE',  ( 122.8495968585647660, 6.109999999999996767, 1.637169565754163836 ) ) ;
#33870=CARTESIAN_POINT ( 'NONE',  ( 125.2500000000000000, -9.735942053221458872E-16, 7.950000000000000178 ) ) ;
#33876=CARTESIAN_POINT ( 'NONE',  ( 58.45833333333333570, 3.974999999999997424, 6.884901960086288852 ) ) ;
#33906=CARTESIAN_POINT ( 'NONE',  ( 116.6000270504628844, 5.819803920172570422, 5.819803920172574863 ) ) ;
#33918=( BOUNDED_CURVE ( )  B_SPLINE_CURVE ( 2, ( #9257, #64400, #108575, #41949, #118771, #8538, #97744, #87583, #86164, #30343, #19466, #96985, #141235 ),
 .UNSPECIFIED., .F., .F. ) 
 B_SPLINE_CURVE_WITH_KNOTS ( ( 3, 2, 2, 2, 2, 2, 3 ),
 ( 0.3166666666666666519, 0.3194444444444444198, 0.3222222222222222432, 0.3250000000000000111, 0.3277777777777777790, 0.3305555555555555469, 0.3333333333333333148 ),
 .UNSPECIFIED. ) 
 CURVE ( )  GEOMETRIC_REPRESENTATION_ITEM ( )  RATIONAL_B_SPLINE_CURVE ( ( 1.000000000000000000, 0.9659258262890683122, 1.000000000000000000, 0.9659258262890683122, 1.000000000000000000, 0.9659258262890683122, 1.000000000000000000, 0.9659258262890683122, 1.000000000000000000, 0.9659258262890683122, 1.000000000000000000, 0.9659258262890683122, 1.000000000000000000 ) ) 
 REPRESENTATION_ITEM ( '' )  );
#33923=CARTESIAN_POINT ( 'NONE',  ( 94.50043019189810423, -3.055000000000002380, 5.291415217122920289 ) ) ;
#33950=CARTESIAN_POINT ( 'NONE',  ( 89.54209685856477563, 5.291415217122923842, -3.054999999999996163 ) ) ;
#33961=CARTESIAN_POINT ( 'NONE',  ( 89.01626352523143737, -4.472830434245839371, 4.472830434245839371 ) ) ;
#33969=EDGE_CURVE ( 'NONE', #96308, #79314, #113479, .T. ) ;
#34000=ORIENTED_EDGE ( 'NONE', *, *, #52449, .F. ) ;
#34010=CARTESIAN_POINT ( 'NONE',  ( 117.5420968585647756, 5.291415217122923842, -3.054999999999996163 ) ) ;
#34046=CARTESIAN_POINT ( 'NONE',  ( 82.59959685856478018, -6.109999999999998543, -1.637169565754160727 ) ) ;
#34047=CARTESIAN_POINT ( 'NONE',  ( 6.181419415492839242, -9.395137122893222781, 1.432941346517488723 ) ) ;
#34091=FACE_OUTER_BOUND ( 'NONE', #81129, .T. ) ;
#34096=CARTESIAN_POINT ( 'NONE',  ( 103.6666666666666714, 6.884901960086285300, 3.975000000000003642 ) ) ;
#34110=CARTESIAN_POINT ( 'NONE',  ( 127.9537635252314658, -6.109999999999998543, -3.741295971395162543E-16 ) ) ;
#34119=CARTESIAN_POINT ( 'NONE',  ( 116.8129301918981184, -1.637169565754159617, -6.110000000000001208 ) ) ;
#34127=CARTESIAN_POINT ( 'NONE',  ( 111.6204301918981088, 3.055000000000001936, -5.291415217122916737 ) ) ;
#34136=CARTESIAN_POINT ( 'NONE',  ( 40.54209685856477563, 5.291415217122923842, -3.054999999999996163 ) ) ;
#34145=CARTESIAN_POINT ( 'NONE',  ( 28.93293019189811943, 1.637169565754156508, 6.110000000000000320 ) ) ;
#34168=AXIS2_PLACEMENT_3D ( 'NONE', #32232, #21353, #121367 ) ;
#34172=CARTESIAN_POINT ( 'NONE',  ( 43.07876352523144448, -7.482591942790325086E-16, 6.109999999999998543 ) ) ;
#34206=CARTESIAN_POINT ( 'NONE',  ( 113.3704301918981230, -3.055000000000001936, 5.291415217122918513 ) ) ;
#34209=DIRECTION ( 'NONE',  ( -1.000000000000000000, -0.000000000000000000, -0.000000000000000000 ) ) ;
#34247=CARTESIAN_POINT ( 'NONE',  ( 29.37043019189811233, -3.055000000000001936, 5.291415217122918513 ) ) ;
#34262=CARTESIAN_POINT ( 'NONE',  ( 119.5837635252314470, -6.110000000000001208, -3.741295971395164515E-16 ) ) ;
#34272=CARTESIAN_POINT ( 'NONE',  ( 44.70419371712955581, -6.884901960086285300, -3.975000000000000089 ) ) ;
#34277=CARTESIAN_POINT ( 'NONE',  ( 43.58333333333333570, 6.884901960086290629, -3.974999999999994316 ) ) ;
#34284=CARTESIAN_POINT ( 'NONE',  ( 40.97959685856477563, 6.109999999999999432, 1.637169565754164280 ) ) ;
#34297=CARTESIAN_POINT ( 'NONE',  ( 39.45419371712956291, 6.884901960086283523, 3.975000000000002753 ) ) ;
#34307=CARTESIAN_POINT ( 'NONE',  ( 62.32876352523145158, 0.000000000000000000, -6.109999999999998543 ) ) ;
#34312=CYLINDRICAL_SURFACE ( 'NONE', #125756, 7.950000000000000178 ) ;
#34331=AXIS2_PLACEMENT_3D ( 'NONE', #46713, #90895, #124210 ) ;
#34337=CARTESIAN_POINT ( 'NONE',  ( 74.28709685856478018, 3.054999999999997495, 5.291415217122919401 ) ) ;
#34388=CARTESIAN_POINT ( 'NONE',  ( 27.54166666666665719, -3.975000000000002753, 6.884901960086286188 ) ) ;
#34404=CARTESIAN_POINT ( 'NONE',  ( 65.41252705046289861, -7.949999999999998401, -4.867971026610728450E-16 ) ) ;
#34408=ORIENTED_EDGE ( 'NONE', *, *, #130157, .T. ) ;
#34413=CARTESIAN_POINT ( 'NONE',  ( 52.84959685856479439, 6.109999999999997655, 1.637169565754163836 ) ) ;
#34439=CARTESIAN_POINT ( 'NONE',  ( 73.43336038379621300, 2.130196079827431532, -7.949999999999997513 ) ) ;
#34443=CARTESIAN_POINT ( 'NONE',  ( 72.45833333333332860, 3.974999999999997424, 6.884901960086288852 ) ) ;
#34453=CARTESIAN_POINT ( 'NONE',  ( 68.39626352523141861, 4.472830434245840259, -4.472830434245839371 ) ) ;
#34477=CARTESIAN_POINT ( 'NONE',  ( 53.95876352523143282, 0.000000000000000000, -6.110000000000001208 ) ) ;
#34483=CARTESIAN_POINT ( 'NONE',  ( 125.4958603837962272, -3.974999999999998312, -6.884901960086286188 ) ) ;
#34505=CARTESIAN_POINT ( 'NONE',  ( 104.7662635252314516, 4.472830434245838482, -4.472830434245837594 ) ) ;
#34527=CARTESIAN_POINT ( 'NONE',  ( 88.50000000000000000, 0.000000000000000000, -7.950000000000000178 ) ) ;
#34535=CARTESIAN_POINT ( 'NONE',  ( 58.77126352523141861, 4.472830434245838482, 4.472830434245842035 ) ) ;
#34542=CARTESIAN_POINT ( 'NONE',  ( 93.77126352523141861, 4.472830434245838482, 4.472830434245842035 ) ) ;
#34587=CARTESIAN_POINT ( 'NONE',  ( 8.901524630118204939, 8.548075541684278633, -4.146687777219522530 ) ) ;
#34588=DIRECTION ( 'NONE',  ( 0.000000000000000000, 0.000000000000000000, 1.000000000000000000 ) ) ;
#34601=LINE ( 'NONE', #91820, #58839 ) ;
#34604=VERTEX_POINT ( 'NONE', #90576 ) ;
#34608=CARTESIAN_POINT ( 'NONE',  ( 105.3708603837962272, 6.884901960086289741, -3.974999999999993427 ) ) ;
#34624=CARTESIAN_POINT ( 'NONE',  ( 89.54209685856477563, 5.291415217122923842, -3.054999999999996163 ) ) ;
#34645=CARTESIAN_POINT ( 'NONE',  ( 101.8708603837962272, 6.884901960086289741, -3.974999999999993427 ) ) ;
#34655=CARTESIAN_POINT ( 'NONE',  ( 96.25043019189810423, 3.055000000000002824, -5.291415217122919401 ) ) ;
#34668=CARTESIAN_POINT ( 'NONE',  ( 89.59959685856475176, -6.109999999999997655, -1.637169565754160283 ) ) ;
#34681=DIRECTION ( 'NONE',  ( -1.000000000000000000, 0.000000000000000000, -0.000000000000000000 ) ) ;
#34718=CARTESIAN_POINT ( 'NONE',  ( 114.7712635252314328, 4.472830434245838482, 4.472830434245842035 ) ) ;
#34740=CARTESIAN_POINT ( 'NONE',  ( 107.8500270504628844, -5.819803920172573086, -5.819803920172573086 ) ) ;
#34753=CARTESIAN_POINT ( 'NONE',  ( 85.22459685856478018, -1.637169565754161171, 6.109999999999998543 ) ) ;
#34804=CARTESIAN_POINT ( 'NONE',  ( 101.4791666666666430, -7.950000000000001066, 2.130196079827424427 ) ) ;
#34818=EDGE_LOOP ( 'NONE', ( #49664, #123870, #28504, #29263 ) ) ;
#34821=CARTESIAN_POINT ( 'NONE',  ( 128.0995968585647802, -6.109999999999997655, -1.637169565754160283 ) ) ;
#34835=CARTESIAN_POINT ( 'NONE',  ( 122.3545968585647472, -1.637169565754161615, 6.110000000000000320 ) ) ;
#34848=CARTESIAN_POINT ( 'NONE',  ( 116.4329301918981088, 1.637169565754156508, 6.110000000000000320 ) ) ;
#34853=( GEOMETRIC_REPRESENTATION_CONTEXT ( 3 ) GLOBAL_UNCERTAINTY_ASSIGNED_CONTEXT ( ( #88254 ) ) GLOBAL_UNIT_ASSIGNED_CONTEXT ( ( #118250, #20360, #42882 ) ) REPRESENTATION_CONTEXT ( 'NONE', 'WORKASPACE' ) );
#34864=CARTESIAN_POINT ( 'NONE',  ( 31.84959685856478373, 6.109999999999996767, 1.637169565754163836 ) ) ;
#34866=CARTESIAN_POINT ( 'NONE',  ( 84.99999999999998579, 0.000000000000000000, -7.950000000000000178 ) ) ;
#34896=CARTESIAN_POINT ( 'NONE',  ( 51.09959685856478728, -6.109999999999997655, -1.637169565754160283 ) ) ;
#34929=CARTESIAN_POINT ( 'NONE',  ( 106.6620968585647802, -5.291415217122919401, 3.054999999999998384 ) ) ;
#34931=( BOUNDED_CURVE ( )  B_SPLINE_CURVE ( 2, ( #43435, #65931, #132622, #2017, #10770, #109397, #90516, #55038, #123155, #68089, #78217, #99206, #23068 ),
 .UNSPECIFIED., .F., .T. ) 
 B_SPLINE_CURVE_WITH_KNOTS ( ( 3, 2, 2, 2, 2, 2, 3 ),
 ( 0.1166666666666666685, 0.1194444444444444503, 0.1222222222222222182, 0.1250000000000000000, 0.1277777777777777679, 0.1305555555555555636, 0.1333333333333333315 ),
 .UNSPECIFIED. ) 
 CURVE ( )  GEOMETRIC_REPRESENTATION_ITEM ( )  RATIONAL_B_SPLINE_CURVE ( ( 1.000000000000000000, 0.9659258262890683122, 1.000000000000000000, 0.9659258262890683122, 1.000000000000000000, 0.9659258262890683122, 1.000000000000000000, 0.9659258262890683122, 1.000000000000000000, 0.9659258262890683122, 1.000000000000000000, 0.9659258262890683122, 1.000000000000000000 ) ) 
 REPRESENTATION_ITEM ( '' )  );
#34940=AXIS2_PLACEMENT_3D ( 'NONE', #72970, #117126, #106232 ) ;
#34997=CARTESIAN_POINT ( 'NONE',  ( 126.2920968585647614, -5.291415217122921177, 3.054999999999999272 ) ) ;
#35007=CARTESIAN_POINT ( 'NONE',  ( 50.53752705046289861, -9.735942053221456900E-16, 7.949999999999998401 ) ) ;
#35014=CARTESIAN_POINT ( 'NONE',  ( 48.83333333333332860, -6.884901960086287964, 3.974999999999998312 ) ) ;
#35024=CARTESIAN_POINT ( 'NONE',  ( 35.00043019189810423, -3.055000000000002380, 5.291415217122920289 ) ) ;
#35046=CARTESIAN_POINT ( 'NONE',  ( 55.91209685856478018, 5.291415217122921177, -3.054999999999994831 ) ) ;
#35077=CARTESIAN_POINT ( 'NONE',  ( 76.47459685856476597, 1.637169565754164280, -6.109999999999996767 ) ) ;
#35084=CARTESIAN_POINT ( 'NONE',  ( 121.7500000000000000, -9.735942053221458872E-16, 7.950000000000000178 ) ) ;
#35095=AXIS2_PLACEMENT_3D ( 'NONE', #108557, #65128, #33231 ) ;
#35103=CARTESIAN_POINT ( 'NONE',  ( 25.81293019189810778, -1.637169565754159617, -6.110000000000001208 ) ) ;
#35134=EDGE_CURVE ( 'NONE', #122112, #75931, #73926, .T. ) ;
#35143=CARTESIAN_POINT ( 'NONE',  ( 65.26669371712957002, -7.949999999999998401, 2.130196079827423983 ) ) ;
#35154=CARTESIAN_POINT ( 'NONE',  ( 57.51626352523144448, -4.472830434245839371, 4.472830434245839371 ) ) ;
#35168=CYLINDRICAL_SURFACE ( 'NONE', #138782, 7.950000000000000178 ) ;
#35176=COLOUR_RGB ( '', 0.72549020, 0.75294118, 0.79215686) ;
#35179=CARTESIAN_POINT ( 'NONE',  ( 77.95419371712955581, 6.884901960086283523, 3.975000000000002753 ) ) ;
#35184=CARTESIAN_POINT ( 'NONE',  ( 72.60416666666665719, 2.130196079827422206, 7.950000000000001954 ) ) ;
#35196=CARTESIAN_POINT ( 'NONE',  ( 68.25043019189810423, 3.055000000000002824, -5.291415217122919401 ) ) ;
#35207=CARTESIAN_POINT ( 'NONE',  ( 86.45833333333332860, 3.974999999999997424, 6.884901960086288852 ) ) ;
#35217=CARTESIAN_POINT ( 'NONE',  ( 54.97959685856476852, 6.109999999999999432, 1.637169565754164280 ) ) ;
#35223=CARTESIAN_POINT ( 'NONE',  ( 53.64583333333331439, 2.130196079827356037, -7.950000000000043698 ) ) ;
#35226=EDGE_CURVE ( 'NONE', #20647, #82847, #9987, .T. ) ;
#35250=CARTESIAN_POINT ( 'NONE',  ( 99.66209685856478018, -5.291415217122919401, 3.054999999999997939 ) ) ;
#35281=CARTESIAN_POINT ( 'NONE',  ( 52.20876352523143282, -7.482591942790329030E-16, 6.110000000000001208 ) ) ;
#35285=CARTESIAN_POINT ( 'NONE',  ( 88.08376352523144703, -6.110000000000001208, -3.741295971395164515E-16 ) ) ;
#35295=CARTESIAN_POINT ( 'NONE',  ( 126.9329301918981088, 1.637169565754156730, 6.110000000000001208 ) ) ;
#35323=VECTOR ( 'NONE', #61411, 1000.000000000000000 ) ;
#35350=CARTESIAN_POINT ( 'NONE',  ( 105.2250270504628986, 5.819803920172573086, -5.819803920172572198 ) ) ;
#35371=CARTESIAN_POINT ( 'NONE',  ( 92.89626352523143282, 4.472830434245840259, -4.472830434245839371 ) ) ;
#35389=CARTESIAN_POINT ( 'NONE',  ( 102.1625270504628844, 7.949999999999998401, 1.460391307983218338E-15 ) ) ;
#35396=CARTESIAN_POINT ( 'NONE',  ( 83.12543019189810423, 5.291415217122919401, 3.055000000000002824 ) ) ;
#35407=CARTESIAN_POINT ( 'NONE',  ( 103.0833333333333286, 6.884901960086290629, -3.974999999999994316 ) ) ;
#35411=CARTESIAN_POINT ( 'NONE',  ( 88.87043019189810877, -3.055000000000001492, 5.291415217122917625 ) ) ;
#35417=AXIS2_PLACEMENT_3D ( 'NONE', #50338, #130037, #118425 ) ;
#35423=FACE_BOUND ( 'NONE', #107494, .T. ) ;
#35447=ORIENTED_EDGE ( 'NONE', *, *, #21569, .F. ) ;
#35460=CARTESIAN_POINT ( 'NONE',  ( 122.3545968585647614, -1.637169565754161615, 6.110000000000000320 ) ) ;
#35496=CARTESIAN_POINT ( 'NONE',  ( 82.16209685856479439, -5.291415217122919401, 3.054999999999998384 ) ) ;
#35499=CARTESIAN_POINT ( 'NONE',  ( 97.78752705046289861, 0.000000000000000000, -7.949999999999998401 ) ) ;
#35510=EDGE_CURVE ( 'NONE', #66568, #91210, #58334, .T. ) ;
#35548=CARTESIAN_POINT ( 'NONE',  ( 92.00000000000000000, 0.000000000000000000, -7.950000000000000178 ) ) ;
#35554=CARTESIAN_POINT ( 'NONE',  ( 0.000000000000000000, 0.000000000000000000, 0.000000000000000000 ) ) ;
#35555=CARTESIAN_POINT ( 'NONE',  ( 14.11365817810131240, 9.243498355973924774, 2.206088284637460983 ) ) ;
#35556=ORIENTED_EDGE ( 'NONE', *, *, #89113, .T. ) ;
#35561=CARTESIAN_POINT ( 'NONE',  ( 126.0875899665068403, 5.292509191841936023, -5.124245105880927298 ) ) ;
#35568=CARTESIAN_POINT ( 'NONE',  ( 26.99999999999999645, 5.837062628940091535, 2.500239961634333596 ) ) ;
#35575=CARTESIAN_POINT ( 'NONE',  ( 113.8962635252314328, 4.472830434245840259, -4.472830434245839371 ) ) ;
#35579=CARTESIAN_POINT ( 'NONE',  ( 100.1666666666666714, 6.884901960086285300, 3.975000000000003642 ) ) ;
#35585=CARTESIAN_POINT ( 'NONE',  ( 115.4120968585647944, 5.291415217122921177, -3.054999999999994831 ) ) ;
#35601=CARTESIAN_POINT ( 'NONE',  ( 34.62043019189811588, 3.055000000000001936, -5.291415217122916737 ) ) ;
#35609=CARTESIAN_POINT ( 'NONE',  ( 0.000000000000000000, 0.000000000000000000, 0.000000000000000000 ) ) ;
#35627=CARTESIAN_POINT ( 'NONE',  ( 40.89126352523144448, -4.472830434245838482, -4.472830434245838482 ) ) ;
#35666=ORIENTED_EDGE ( 'NONE', *, *, #107835, .T. ) ;
#35667=CARTESIAN_POINT ( 'NONE',  ( 110.0162635252314374, -4.472830434245839371, 4.472830434245839371 ) ) ;
#35682=CARTESIAN_POINT ( 'NONE',  ( 120.1458333333333428, 2.130196079827394229, -7.950000000000021494 ) ) ;
#35716=CARTESIAN_POINT ( 'NONE',  ( 124.2291666666666714, 7.950000000000001954, -2.130196079827421762 ) ) ;
#35732=CARTESIAN_POINT ( 'NONE',  ( 125.1254301918981184, 5.291415217122919401, 3.055000000000002824 ) ) ;
#35741=CARTESIAN_POINT ( 'NONE',  ( 48.78752705046289151, 0.000000000000000000, -7.949999999999998401 ) ) ;
#35747=CARTESIAN_POINT ( 'NONE',  ( 42.27083333333331439, -7.949999999999999289, -2.130196079827426203 ) ) ;
#35754=CARTESIAN_POINT ( 'NONE',  ( 41.85459685856477563, -1.637169565754161615, 6.110000000000000320 ) ) ;
#35768=CARTESIAN_POINT ( 'NONE',  ( 38.72502705046289151, 5.819803920172573974, -5.819803920172573086 ) ) ;
#35774=CARTESIAN_POINT ( 'NONE',  ( 55.18293019189810877, -1.637169565754158951, -6.109999999999998543 ) ) ;
#35801=CARTESIAN_POINT ( 'NONE',  ( 72.09959685856479439, -6.109999999999997655, -1.637169565754160283 ) ) ;
#35803=( BOUNDED_CURVE ( )  B_SPLINE_CURVE ( 2, ( #6579, #105225, #114658, #71197, #115345, #18179, #49462, #82777, #103771, #93650, #139322, #137879, #95775 ),
 .UNSPECIFIED., .F., .T. ) 
 B_SPLINE_CURVE_WITH_KNOTS ( ( 3, 2, 2, 2, 2, 2, 3 ),
 ( 0.4333333333333333481, 0.4361111111111111160, 0.4388888888888888840, 0.4416666666666666519, 0.4444444444444444198, 0.4472222222222222432, 0.4500000000000000111 ),
 .UNSPECIFIED. ) 
 CURVE ( )  GEOMETRIC_REPRESENTATION_ITEM ( )  RATIONAL_B_SPLINE_CURVE ( ( 1.000000000000000000, 0.9659258262890683122, 1.000000000000000000, 0.9659258262890683122, 1.000000000000000000, 0.9659258262890683122, 1.000000000000000000, 0.9659258262890683122, 1.000000000000000000, 0.9659258262890683122, 1.000000000000000000, 0.9659258262890683122, 1.000000000000000000 ) ) 
 REPRESENTATION_ITEM ( '' )  );
#35823=CARTESIAN_POINT ( 'NONE',  ( 31.06293019189809712, 1.637169565754157174, 6.110000000000002984 ) ) ;
#35826=( BOUNDED_CURVE ( )  B_SPLINE_CURVE ( 2, ( #68139, #78264, #69539, #670, #47796, #81120, #112316, #90564, #102157, #136188, #122446, #23111, #35499 ),
 .UNSPECIFIED., .F., .F. ) 
 B_SPLINE_CURVE_WITH_KNOTS ( ( 3, 2, 2, 2, 2, 2, 3 ),
 ( 0.2833333333333333259, 0.2861111111111110938, 0.2888888888888888618, 0.2916666666666666852, 0.2944444444444444531, 0.2972222222222222210, 0.2999999999999999889 ),
 .UNSPECIFIED. ) 
 CURVE ( )  GEOMETRIC_REPRESENTATION_ITEM ( )  RATIONAL_B_SPLINE_CURVE ( ( 1.000000000000000000, 0.9659258262890683122, 1.000000000000000000, 0.9659258262890683122, 1.000000000000000000, 0.9659258262890683122, 1.000000000000000000, 0.9659258262890683122, 1.000000000000000000, 0.9659258262890683122, 1.000000000000000000, 0.9659258262890683122, 1.000000000000000000 ) ) 
 REPRESENTATION_ITEM ( '' )  );
#35855=CARTESIAN_POINT ( 'NONE',  ( 28.70833333333332149, -3.974999999999999201, -6.884901960086287964 ) ) ;
#35867=CARTESIAN_POINT ( 'NONE',  ( 25.60725813788241112, -3.175000000000001155, -5.499261314031188341 ) ) ;
#35877=CARTESIAN_POINT ( 'NONE',  ( 57.22459685856476597, -1.637169565754161171, 6.109999999999998543 ) ) ;
#35899=CARTESIAN_POINT ( 'NONE',  ( 76.35002705046288440, -5.819803920172572198, -5.819803920172572198 ) ) ;
#35904=CARTESIAN_POINT ( 'NONE',  ( 77.70833333333332860, -3.974999999999999201, -6.884901960086287964 ) ) ;
#35914=CARTESIAN_POINT ( 'NONE',  ( 66.06293019189810423, 1.637169565754157174, 6.110000000000002984 ) ) ;
#35922=CARTESIAN_POINT ( 'NONE',  ( 85.72916666666665719, 7.950000000000001954, -2.130196079827421762 ) ) ;
#35931=CARTESIAN_POINT ( 'NONE',  ( 56.00043019189809712, -3.055000000000002380, 5.291415217122920289 ) ) ;
#35938=CARTESIAN_POINT ( 'NONE',  ( 53.93750000000000000, 5.819803920172574863, -5.819803920172573086 ) ) ;
#35944=ORIENTED_EDGE ( 'NONE', *, *, #13676, .F. ) ;
#35948=CARTESIAN_POINT ( 'NONE',  ( 112.2250270504628702, 5.819803920172573974, -5.819803920172573086 ) ) ;
#35961=CARTESIAN_POINT ( 'NONE',  ( 100.8287635252314516, 0.000000000000000000, -6.109999999999998543 ) ) ;
#35981=CARTESIAN_POINT ( 'NONE',  ( 52.35459685856476852, -1.637169565754161615, 6.110000000000000320 ) ) ;
#35986=CARTESIAN_POINT ( 'NONE',  ( 91.43793019189810423, -6.110000000000001208, 1.637169565754158951 ) ) ;
#36000=CARTESIAN_POINT ( 'NONE',  ( 127.9537635252314658, -6.109999999999999432, -3.741295971395163529E-16 ) ) ;
#36034=CARTESIAN_POINT ( 'NONE',  ( 8.899418659112473762, 8.548380951428034891, 4.146088043936330791 ) ) ;
#36056=CARTESIAN_POINT ( 'NONE',  ( 104.4958603837962272, -3.974999999999998312, -6.884901960086286188 ) ) ;
#36070=CARTESIAN_POINT ( 'NONE',  ( 97.85459685856477563, -1.637169565754161615, 6.110000000000000320 ) ) ;
#36094=CARTESIAN_POINT ( 'NONE',  ( 87.79209685856477563, -5.291415217122921177, 3.054999999999999272 ) ) ;
#36105=CARTESIAN_POINT ( 'NONE',  ( 77.05793019189810877, 6.110000000000000320, -1.637169565754156064 ) ) ;
#36134=CARTESIAN_POINT ( 'NONE',  ( 127.0000000000000000, 0.000000000000000000, 0.000000000000000000 ) ) ;
#36145=ORIENTED_EDGE ( 'NONE', *, *, #104833, .T. ) ;
#36151=CARTESIAN_POINT ( 'NONE',  ( 115.5004301918981042, -3.055000000000002380, 5.291415217122920289 ) ) ;
#36159=EDGE_CURVE ( 'NONE', #2613, #123729, #21610, .T. ) ;
#36170=CARTESIAN_POINT ( 'NONE',  ( 114.3124999999999858, 5.819803920172571310, 5.819803920172576639 ) ) ;
#36177=VERTEX_POINT ( 'NONE', #141228 ) ;
#36193=ORIENTED_EDGE ( 'NONE', *, *, #69297, .F. ) ;
#36208=CARTESIAN_POINT ( 'NONE',  ( 105.7083333333333286, -3.974999999999999201, -6.884901960086287964 ) ) ;
#36214=VECTOR ( 'NONE', #93849, 1000.000000000000000 ) ;
#36233=CARTESIAN_POINT ( 'NONE',  ( 88.50000000000000000, 0.000000000000000000, -7.950000000000000178 ) ) ;
#36249=CARTESIAN_POINT ( 'NONE',  ( 27.00000000000001066, 4.895760287860418281, 5.464752967159129504 ) ) ;
#36256=CARTESIAN_POINT ( 'NONE',  ( 113.1670968585647756, -3.055000000000000160, -5.291415217122921177 ) ) ;
#36266=CARTESIAN_POINT ( 'NONE',  ( 107.8287635252314516, 0.000000000000000000, -6.109999999999998543 ) ) ;
#36279=CARTESIAN_POINT ( 'NONE',  ( 27.76626352523143737, 4.472830434245839371, -4.472830434245838482 ) ) ;
#36312=CARTESIAN_POINT ( 'NONE',  ( 40.30793019189810877, -6.109999999999998543, 1.637169565754158507 ) ) ;
#36348=CARTESIAN_POINT ( 'NONE',  ( 114.8287635252314516, 0.000000000000000000, -6.109999999999999432 ) ) ;
#36386=CARTESIAN_POINT ( 'NONE',  ( 125.7291446111226350, -5.312392442408975235, 5.610871146360816297 ) ) ;
#36392=CARTESIAN_POINT ( 'NONE',  ( 119.2708333333333144, -7.949999999999999289, -2.130196079827426203 ) ) ;
#36404=CARTESIAN_POINT ( 'NONE',  ( 115.7920968585647756, -5.291415217122921177, 3.054999999999999272 ) ) ;
#36415=CARTESIAN_POINT ( 'NONE',  ( 46.74586038379622011, 3.974999999999996980, 6.884901960086287964 ) ) ;
#36421=CARTESIAN_POINT ( 'NONE',  ( 39.64583333333332860, 2.130196079827431976, -7.949999999999999289 ) ) ;
#36430=CARTESIAN_POINT ( 'NONE',  ( 128.3912635252314374, -4.472830434245839371, -4.472830434245839371 ) ) ;
#36452=CARTESIAN_POINT ( 'NONE',  ( 61.59959685856478018, -6.109999999999997655, -1.637169565754160283 ) ) ;
#36461=( BOUNDED_CURVE ( )  B_SPLINE_CURVE ( 2, ( #120131, #99103, #32463, #120871, #55645, #52754, #88272, #141196, #78110, #122289, #131055, #111426, #108538 ),
 .UNSPECIFIED., .F., .F. ) 
 B_SPLINE_CURVE_WITH_KNOTS ( ( 3, 2, 2, 2, 2, 2, 3 ),
 ( 0.8000000000000000444, 0.8027777777777778123, 0.8055555555555555802, 0.8083333333333333481, 0.8111111111111111160, 0.8138888888888888840, 0.8166666666666666519 ),
 .UNSPECIFIED. ) 
 CURVE ( )  GEOMETRIC_REPRESENTATION_ITEM ( )  RATIONAL_B_SPLINE_CURVE ( ( 1.000000000000000000, 0.9659258262890683122, 1.000000000000000000, 0.9659258262890683122, 1.000000000000000000, 0.9659258262890683122, 1.000000000000000000, 0.9659258262890683122, 1.000000000000000000, 0.9659258262890683122, 1.000000000000000000, 0.9659258262890683122, 1.000000000000000000 ) ) 
 REPRESENTATION_ITEM ( '' )  );
#36478=CARTESIAN_POINT ( 'NONE',  ( 62.62043019189811588, 3.055000000000001936, -5.291415217122916737 ) ) ;
#36503=CARTESIAN_POINT ( 'NONE',  ( 29.14583333333332504, 2.130196079827431976, -7.949999999999998401 ) ) ;
#36513=CARTESIAN_POINT ( 'NONE',  ( 120.2458603837962272, 3.974999999999996980, 6.884901960086287964 ) ) ;
#36550=CARTESIAN_POINT ( 'NONE',  ( 60.57876352523145158, -7.482591942790327058E-16, 6.109999999999999432 ) ) ;
#36569=CARTESIAN_POINT ( 'NONE',  ( 79.55836038379622721, -7.949999999999997513, -2.130196079827425759 ) ) ;
#36573=CARTESIAN_POINT ( 'NONE',  ( 61.95833333333332149, 3.974999999999997424, 6.884901960086288852 ) ) ;
#36581=CARTESIAN_POINT ( 'NONE',  ( 68.54209685856477563, 5.291415217122923842, -3.054999999999996163 ) ) ;
#36594=CARTESIAN_POINT ( 'NONE',  ( 0.000000000000000000, 0.000000000000000000, 0.000000000000000000 ) ) ;
#36607=DIRECTION ( 'NONE',  ( 0.000000000000000000, 0.000000000000000000, 1.000000000000000000 ) ) ;
#36634=CARTESIAN_POINT ( 'NONE',  ( 95.57876352523145158, -7.482591942790325086E-16, 6.109999999999998543 ) ) ;
#36646=CARTESIAN_POINT ( 'NONE',  ( 68.66666666666665719, 6.884901960086285300, 3.975000000000003642 ) ) ;
#36658=CARTESIAN_POINT ( 'NONE',  ( 58.04209685856477563, 5.291415217122923842, -3.054999999999996163 ) ) ;
#36674=CARTESIAN_POINT ( 'NONE',  ( 127.3704301918981088, -3.055000000000001936, 5.291415217122918513 ) ) ;
#36708=CARTESIAN_POINT ( 'NONE',  ( 10.03137119346127726, 8.432637487761468265, 4.375000000000001776 ) ) ;
#36729=ORIENTED_EDGE ( 'NONE', *, *, #7958, .T. ) ;
#36732=CARTESIAN_POINT ( 'NONE',  ( 121.2666937171295700, -7.949999999999998401, 2.130196079827423983 ) ) ;
#36737=CARTESIAN_POINT ( 'NONE',  ( 102.6000270504628844, 5.819803920172570422, 5.819803920172574863 ) ) ;
#36752=CARTESIAN_POINT ( 'NONE',  ( 95.37543019189810423, -5.291415217122920289, -3.055000000000001492 ) ) ;
#36772=CARTESIAN_POINT ( 'NONE',  ( 81.95876352523143282, 0.000000000000000000, -6.110000000000001208 ) ) ;
#36785=CARTESIAN_POINT ( 'NONE',  ( 76.32876352523145158, 0.000000000000000000, -6.109999999999998543 ) ) ;
#36839=CARTESIAN_POINT ( 'NONE',  ( 117.2504301918981042, 3.055000000000002824, -5.291415217122919401 ) ) ;
#36856=CARTESIAN_POINT ( 'NONE',  ( 114.1666666666666714, 6.884901960086285300, 3.975000000000003642 ) ) ;
#36896=CARTESIAN_POINT ( 'NONE',  ( 105.4166666666666572, -6.884901960086287076, -3.975000000000000977 ) ) ;
#36903=CARTESIAN_POINT ( 'NONE',  ( 127.1000270504628986, 5.819803920172570422, 5.819803920172574863 ) ) ;
#36920=CARTESIAN_POINT ( 'NONE',  ( 91.56250000000000000, -5.819803920172572198, -5.819803920172573086 ) ) ;
#36926=DIRECTION ( 'NONE',  ( -1.000000000000000000, -0.000000000000000000, -0.000000000000000000 ) ) ;
#36947=CARTESIAN_POINT ( 'NONE',  ( 109.5212635252314612, -4.472830434245839371, -4.472830434245840259 ) ) ;
#36958=CARTESIAN_POINT ( 'NONE',  ( 101.9954301918981230, 5.291415217122916737, 3.055000000000001936 ) ) ;
#37006=CARTESIAN_POINT ( 'NONE',  ( 38.84959685856477307, 6.109999999999996767, 1.637169565754163836 ) ) ;
#37009=( BOUNDED_CURVE ( )  B_SPLINE_CURVE ( 2, ( #95358, #140996, #38849, #127269, #41702, #115648, #84511, #61361, #117098, #27970, #72240, #105505, #6171 ),
 .UNSPECIFIED., .F., .T. ) 
 B_SPLINE_CURVE_WITH_KNOTS ( ( 3, 2, 2, 2, 2, 2, 3 ),
 ( 0.5666666666666666519, 0.5694444444444444198, 0.5722222222222221877, 0.5749999999999999556, 0.5777777777777777235, 0.5805555555555556024, 0.5833333333333333703 ),
 .UNSPECIFIED. ) 
 CURVE ( )  GEOMETRIC_REPRESENTATION_ITEM ( )  RATIONAL_B_SPLINE_CURVE ( ( 1.000000000000000000, 0.9659258262890683122, 1.000000000000000000, 0.9659258262890683122, 1.000000000000000000, 0.9659258262890683122, 1.000000000000000000, 0.9659258262890683122, 1.000000000000000000, 0.9659258262890683122, 1.000000000000000000, 0.9659258262890683122, 1.000000000000000000 ) ) 
 REPRESENTATION_ITEM ( '' )  );
#37013=B_SPLINE_CURVE_WITH_KNOTS ( 'NONE', 3,
 ( #42069, #43479, #86283, #130507, #31186, #669, #87691, #121026, #75401, #120278, #32619, #20994, #10125, #143492, #131927, #10816, #65979, #110136, #77559, #44213, #9375, #88428, #34047, #132668, #44960, #89137, #121728, #53651, #119576, #20273, #92666, #134800, #69538, #100721, #114433, #135498 ),
 .UNSPECIFIED., .F., .F.,
 ( 4, 2, 2, 2, 2, 2, 2, 2, 2, 2, 2, 2, 2, 2, 2, 2, 2, 4 ),
 ( 0.02080955487772951848, 0.02167635536089138754, 0.02254315584405326006, 0.02340995632721513259, 0.02427675681037700164, 0.02514355729353887070, 0.02557695753511981043, 0.02601035777670074670, 0.02687715825986262269, 0.02774395874302449522, 0.02861075922618637468, 0.02947755970934824721, 0.03034436019251012667, 0.03121116067567199920, 0.03207796115883387866, 0.03294476164199575813, 0.03381156212515763065, 0.03467836260831951012 ),
 .UNSPECIFIED. ) ;
#37046=CARTESIAN_POINT ( 'NONE',  ( 105.6412635252314658, 4.472830434245837594, 4.472830434245841147 ) ) ;
#37092=CARTESIAN_POINT ( 'NONE',  ( 116.6458333333333428, 2.130196079827431976, -7.949999999999999289 ) ) ;
#37107=CARTESIAN_POINT ( 'NONE',  ( 113.0212635252314186, -4.472830434245839371, -4.472830434245840259 ) ) ;
#37117=CARTESIAN_POINT ( 'NONE',  ( 36.10002705046289151, 5.819803920172570422, 5.819803920172574863 ) ) ;
#37122=CARTESIAN_POINT ( 'NONE',  ( 40.37499999999999289, 7.950000000000000178, 1.460391307983218535E-15 ) ) ;
#37130=DIRECTION ( 'NONE',  ( -1.000000000000000000, -0.000000000000000000, -0.000000000000000000 ) ) ;
#37137=CARTESIAN_POINT ( 'NONE',  ( 32.37543019189810423, -5.291415217122920289, -3.055000000000001492 ) ) ;
#37159=CARTESIAN_POINT ( 'NONE',  ( 50.66209685856478018, -5.291415217122919401, 3.054999999999997939 ) ) ;
#37163=ORIENTED_EDGE ( 'NONE', *, *, #82817, .F. ) ;
#37188=CARTESIAN_POINT ( 'NONE',  ( 70.64126352523145158, 4.472830434245835818, 4.472830434245840259 ) ) ;
#37218=CARTESIAN_POINT ( 'NONE',  ( 42.22502705046289861, 5.819803920172573974, -5.819803920172573086 ) ) ;
#37227=AXIS2_PLACEMENT_3D ( 'NONE', #109836, #85941, #73646 ) ;
#37261=CARTESIAN_POINT ( 'NONE',  ( 65.99586038379622721, -3.974999999999998312, -6.884901960086286188 ) ) ;
#37273=CARTESIAN_POINT ( 'NONE',  ( 46.28709685856477307, 3.054999999999997939, 5.291415217122920289 ) ) ;
#37295=CARTESIAN_POINT ( 'NONE',  ( 118.1041666666666430, 2.130196079827479050, 7.949999999999969091 ) ) ;
#37296=CARTESIAN_POINT ( 'NONE',  ( 79.85002705046289861, -5.819803920172572198, -5.819803920172572198 ) ) ;
#37300=CARTESIAN_POINT ( 'NONE',  ( 65.31250000000000000, 5.819803920172571310, 5.819803920172575751 ) ) ;
#37312=CARTESIAN_POINT ( 'NONE',  ( 54.39626352523144703, 4.472830434245840259, -4.472830434245839371 ) ) ;
#37346=FACE_OUTER_BOUND ( 'NONE', #49973, .T. ) ;
#37368=CARTESIAN_POINT ( 'NONE',  ( 89.89126352523143737, -4.472830434245838482, -4.472830434245838482 ) ) ;
#37391=CARTESIAN_POINT ( 'NONE',  ( 42.00043019189809712, -3.055000000000002380, 5.291415217122920289 ) ) ;
#37449=CARTESIAN_POINT ( 'NONE',  ( 77.49543019189810877, 5.291415217122917625, 3.055000000000002380 ) ) ;
#37473=CARTESIAN_POINT ( 'NONE',  ( 122.2875270504628844, 0.000000000000000000, -7.949999999999998401 ) ) ;
#37478=CARTESIAN_POINT ( 'NONE',  ( 99.39169371712955581, 2.130196079827421762, 7.950000000000001066 ) ) ;
#37493=EDGE_LOOP ( 'NONE', ( #33483, #93890, #86813, #128708 ) ) ;
#37494=CARTESIAN_POINT ( 'NONE',  ( 80.93793019189807580, -6.110000000000001208, 1.637169565754158951 ) ) ;
#37519=CARTESIAN_POINT ( 'NONE',  ( 84.58376352523144703, -6.110000000000001208, -3.741295971395164515E-16 ) ) ;
#37531=CARTESIAN_POINT ( 'NONE',  ( 73.12043019189812298, 3.055000000000001936, -5.291415217122916737 ) ) ;
#37573=CARTESIAN_POINT ( 'NONE',  ( 70.58376352523143282, -6.110000000000001208, -3.741295971395164515E-16 ) ) ;
#37578=CARTESIAN_POINT ( 'NONE',  ( 107.3337635252314470, 6.110000000000001208, 1.122388791418549305E-15 ) ) ;
#37608=CARTESIAN_POINT ( 'NONE',  ( 14.11270276996059181, -9.243106346249332361, -2.207712314992021696 ) ) ;
#37651=CARTESIAN_POINT ( 'NONE',  ( 106.1458333333333144, 2.130196079827412436, -7.950000000000009059 ) ) ;
#37652=CARTESIAN_POINT ( 'NONE',  ( 126.8083603837962272, 7.949999999999997513, 2.130196079827431088 ) ) ;
#37667=CARTESIAN_POINT ( 'NONE',  ( 94.33333333333332860, -6.884901960086287964, 3.974999999999998312 ) ) ;
#37676=FACE_OUTER_BOUND ( 'NONE', #42936, .T. ) ;
#37681=CARTESIAN_POINT ( 'NONE',  ( 125.5563301804876772, -2.994143682145710805, -7.321028783668758422 ) ) ;
#37693=CARTESIAN_POINT ( 'NONE',  ( 109.6670968585647756, -3.055000000000000160, -5.291415217122921177 ) ) ;
#37703=CARTESIAN_POINT ( 'NONE',  ( 100.6829301918981230, -1.637169565754158951, -6.109999999999998543 ) ) ;
#37750=CARTESIAN_POINT ( 'NONE',  ( 34.91209685856478018, 5.291415217122921177, -3.054999999999994831 ) ) ;
#37785=CARTESIAN_POINT ( 'NONE',  ( 96.89126352523143737, -4.472830434245839371, -4.472830434245839371 ) ) ;
#37814=VERTEX_POINT ( 'NONE', #123753 ) ;
#37839=CARTESIAN_POINT ( 'NONE',  ( 118.1041666666666714, 2.130196079827422206, 7.950000000000001954 ) ) ;
#37852=CARTESIAN_POINT ( 'NONE',  ( 116.2295968585647756, -6.110000000000000320, -1.637169565754161393 ) ) ;
#37854=LINE ( 'NONE', #82089, #90428 ) ;
#37861=CARTESIAN_POINT ( 'NONE',  ( 38.14169371712954870, -2.130196079827424871, -7.949999999999999289 ) ) ;
#37868=CARTESIAN_POINT ( 'NONE',  ( 38.77083333333331439, -7.949999999999999289, -2.130196079827426203 ) ) ;
#37878=CARTESIAN_POINT ( 'NONE',  ( 25.81293019189810778, -1.637169565754159617, -6.110000000000001208 ) ) ;
#37898=CARTESIAN_POINT ( 'NONE',  ( 44.09959685856477307, -6.109999999999997655, -1.637169565754160283 ) ) ;
#37926=CARTESIAN_POINT ( 'NONE',  ( 63.49543019189811588, 5.291415217122916737, 3.055000000000001936 ) ) ;
#37937=CARTESIAN_POINT ( 'NONE',  ( 102.0625000000000000, -5.819803920172573086, -5.819803920172573974 ) ) ;
#37970=CARTESIAN_POINT ( 'NONE',  ( 108.4791666666666714, -7.950000000000000178, 2.130196079827424427 ) ) ;
#38005=CARTESIAN_POINT ( 'NONE',  ( 48.03709685856477307, -3.054999999999999272, -5.291415217122919401 ) ) ;
#38015=DIRECTION ( 'NONE',  ( -1.000000000000000000, -0.000000000000000000, -0.000000000000000000 ) ) ;
#38026=CARTESIAN_POINT ( 'NONE',  ( 64.24586038379621300, 3.974999999999996980, 6.884901960086287964 ) ) ;
#38032=CARTESIAN_POINT ( 'NONE',  ( 63.56249999999999289, -5.819803920172572198, -5.819803920172573086 ) ) ;
#38040=CARTESIAN_POINT ( 'NONE',  ( 57.02126352523143993, -4.472830434245839371, -4.472830434245840259 ) ) ;
#38049=CARTESIAN_POINT ( 'NONE',  ( 100.9958603837962272, -3.974999999999998312, -6.884901960086286188 ) ) ;
#38075=CARTESIAN_POINT ( 'NONE',  ( 62.49586038379623432, -3.974999999999998312, -6.884901960086286188 ) ) ;
#38092=CARTESIAN_POINT ( 'NONE',  ( 97.91209685856478018, 5.291415217122921177, -3.054999999999994831 ) ) ;
#38116=CARTESIAN_POINT ( 'NONE',  ( 47.54209685856476852, 5.291415217122923842, -3.054999999999996163 ) ) ;
#38162=CARTESIAN_POINT ( 'NONE',  ( 95.01669371712955581, 7.950000000000000178, -2.130196079827421318 ) ) ;
#38167=CARTESIAN_POINT ( 'NONE',  ( 70.34959685856478018, 6.109999999999997655, 1.637169565754163836 ) ) ;
#38178=( BOUNDED_CURVE ( )  B_SPLINE_CURVE ( 2, ( #128502, #6657, #81450, #84306, #138669, #69870, #72005, #83580, #48804, #40092, #27741, #50941, #136499 ),
 .UNSPECIFIED., .F., .T. ) 
 B_SPLINE_CURVE_WITH_KNOTS ( ( 3, 2, 2, 2, 2, 2, 3 ),
 ( 0.8666666666666668073, 0.8694444444444445752, 0.8722222222222223431, 0.8750000000000001110, 0.8777777777777778789, 0.8805555555555556468, 0.8833333333333334147 ),
 .UNSPECIFIED. ) 
 CURVE ( )  GEOMETRIC_REPRESENTATION_ITEM ( )  RATIONAL_B_SPLINE_CURVE ( ( 0.9999999999999986677, 0.9659258262890696445, 1.000000000000000000, 0.9659258262890683122, 1.000000000000000000, 0.9659258262890683122, 1.000000000000000000, 0.9659258262890683122, 1.000000000000000000, 0.9659258262890683122, 1.000000000000000000, 0.9659258262890669799, 1.000000000000001332 ) ) 
 REPRESENTATION_ITEM ( '' )  );
#38190=AXIS2_PLACEMENT_3D ( 'NONE', #85240, #74402, #118589 ) ;
#38192=CARTESIAN_POINT ( 'NONE',  ( 91.22502705046289861, 5.819803920172573086, -5.819803920172572198 ) ) ;
#38207=CARTESIAN_POINT ( 'NONE',  ( 84.00043019189810423, -3.055000000000002380, 5.291415217122920289 ) ) ;
#38213=CARTESIAN_POINT ( 'NONE',  ( 118.7875270504628986, 0.000000000000000000, -7.949999999999998401 ) ) ;
#38223=CARTESIAN_POINT ( 'NONE',  ( 79.91709685856476142, 3.054999999999998828, 5.291415217122922066 ) ) ;
#38276=CARTESIAN_POINT ( 'NONE',  ( 72.62543019189810423, 5.291415217122919401, 3.055000000000002824 ) ) ;
#38280=CARTESIAN_POINT ( 'NONE',  ( 95.35416666666665719, -2.130196079827425759, -7.950000000000000178 ) ) ;
#38281=AXIS2_PLACEMENT_3D ( 'NONE', #61339, #28684, #60616 ) ;
#38284=CARTESIAN_POINT ( 'NONE',  ( 111.4170968585647614, 3.054999999999998828, 5.291415217122922066 ) ) ;
#38332=CARTESIAN_POINT ( 'NONE',  ( 74.20833333333331439, -3.974999999999999201, -6.884901960086287964 ) ) ;
#38333=CARTESIAN_POINT ( 'NONE',  ( 0.000000000000000000, 9.735942053221458872E-16, -7.950000000000000178 ) ) ;
#38350=CARTESIAN_POINT ( 'NONE',  ( 30.39126352523144448, -4.472830434245839371, -4.472830434245839371 ) ) ;
#38363=EDGE_CURVE ( 'NONE', #96695, #49146, #62316, .T. ) ;
#38365=CARTESIAN_POINT ( 'NONE',  ( 92.14583333333332860, 2.130196079827431976, -7.949999999999999289 ) ) ;
#38371=CARTESIAN_POINT ( 'NONE',  ( 30.41252705046289151, -7.949999999999998401, -4.867971026610728450E-16 ) ) ;
#38376=CARTESIAN_POINT ( 'NONE',  ( 126.7939054748679411, 4.575466593308011198, 4.853590263963833529 ) ) ;
#38390=CARTESIAN_POINT ( 'NONE',  ( 114.7712635252314186, 4.472830434245839371, 4.472830434245842035 ) ) ;
#38399=CARTESIAN_POINT ( 'NONE',  ( 104.9120968585647802, 5.291415217122921177, -3.054999999999994831 ) ) ;
#38415=LINE ( 'NONE', #67691, #10906 ) ;
#38433=CARTESIAN_POINT ( 'NONE',  ( 27.00000000000001421, 3.441786896390103934, 7.166352137582786774 ) ) ;
#38451=CARTESIAN_POINT ( 'NONE',  ( 40.59959685856477307, -6.109999999999997655, -1.637169565754160283 ) ) ;
#38464=EDGE_CURVE ( 'NONE', #46474, #82404, #33323, .T. ) ;
#38485=CARTESIAN_POINT ( 'NONE',  ( 98.05793019189812298, 6.110000000000001208, -1.637169565754156286 ) ) ;
#38527=CARTESIAN_POINT ( 'NONE',  ( 29.53752705046289151, -9.735942053221456900E-16, 7.949999999999998401 ) ) ;
#38530=VERTEX_POINT ( 'NONE', #95751 ) ;
#38534=CARTESIAN_POINT ( 'NONE',  ( 124.0833333333333428, 6.884901960086290629, -3.974999999999994316 ) ) ;
#38547=CARTESIAN_POINT ( 'NONE',  ( 110.2504301918981042, 3.055000000000002824, -5.291415217122919401 ) ) ;
#38555=CARTESIAN_POINT ( 'NONE',  ( 33.76669371712955581, -7.949999999999999289, 2.130196079827424427 ) ) ;
#38560=CARTESIAN_POINT ( 'NONE',  ( 32.64583333333332860, 2.130196079827431976, -7.949999999999999289 ) ) ;
#38570=CARTESIAN_POINT ( 'NONE',  ( 33.10459685856476852, 1.637169565754164946, -6.109999999999999432 ) ) ;
#38581=CARTESIAN_POINT ( 'NONE',  ( 58.62543019189810423, 5.291415217122919401, 3.055000000000002824 ) ) ;
#38591=CARTESIAN_POINT ( 'NONE',  ( 47.59959685856478018, -6.109999999999997655, -1.637169565754160283 ) ) ;
#38623=CARTESIAN_POINT ( 'NONE',  ( 70.05793019189810877, 6.110000000000000320, -1.637169565754156064 ) ) ;
#38668=CARTESIAN_POINT ( 'NONE',  ( 109.5000000000000000, 0.000000000000000000, -7.950000000000000178 ) ) ;
#38700=CARTESIAN_POINT ( 'NONE',  ( 51.09959685856477307, -6.109999999999998543, -1.637169565754160727 ) ) ;
#38723=CARTESIAN_POINT ( 'NONE',  ( 64.97502705046288440, -5.819803920172572198, 5.819803920172572198 ) ) ;
#38728=( BOUNDED_CURVE ( )  B_SPLINE_CURVE ( 2, ( #21312, #65570, #109739, #10409, #54669, #132241, #121323, #32933, #19866, #140241, #85130, #8943, #30026 ),
 .UNSPECIFIED., .F., .T. ) 
 B_SPLINE_CURVE_WITH_KNOTS ( ( 3, 2, 2, 2, 2, 2, 3 ),
 ( 0.8333333333333333703, 0.8361111111111111382, 0.8388888888888889062, 0.8416666666666666741, 0.8444444444444444420, 0.8472222222222222099, 0.8499999999999999778 ),
 .UNSPECIFIED. ) 
 CURVE ( )  GEOMETRIC_REPRESENTATION_ITEM ( )  RATIONAL_B_SPLINE_CURVE ( ( 1.000000000000000000, 0.9659258262890683122, 1.000000000000000000, 0.9659258262890683122, 1.000000000000000000, 0.9659258262890683122, 1.000000000000000000, 0.9659258262890683122, 1.000000000000000000, 0.9659258262890683122, 1.000000000000000000, 0.9659258262890683122, 1.000000000000000000 ) ) 
 REPRESENTATION_ITEM ( '' )  );
#38729=CARTESIAN_POINT ( 'NONE',  ( 66.33333333333332860, -6.884901960086287964, 3.974999999999998312 ) ) ;
#38735=CARTESIAN_POINT ( 'NONE',  ( 127.2530914712157113, -1.701477371937629046, -6.349999999999998757 ) ) ;
#38737=CARTESIAN_POINT ( 'NONE',  ( 55.41709685856477563, 3.054999999999998828, 5.291415217122922066 ) ) ;
#38739=CYLINDRICAL_SURFACE ( 'NONE', #143195, 9.500000000000001776 ) ;
#38755=ADVANCED_FACE ( 'NONE', ( #34091 ), #13009, .T. ) ;
#38775=CARTESIAN_POINT ( 'NONE',  ( 61.03752705046289151, -9.735942053221456900E-16, 7.949999999999998401 ) ) ;
#38784=DIRECTION ( 'NONE',  ( -1.000000000000000000, -0.000000000000000000, -0.000000000000000000 ) ) ;
#38793=CARTESIAN_POINT ( 'NONE',  ( 91.78709685856478018, 3.054999999999997495, 5.291415217122919401 ) ) ;
#38818=CARTESIAN_POINT ( 'NONE',  ( 41.56293019189810423, 1.637169565754157174, 6.110000000000002984 ) ) ;
#38830=CARTESIAN_POINT ( 'NONE',  ( 10.32500000000000107, -9.500000000000001776, 0.000000000000000000 ) ) ;
#38832=ORIENTED_EDGE ( 'NONE', *, *, #10608, .F. ) ;
#38839=PRODUCT_DEFINITION_SHAPE ( 'NONE', 'NONE',  #14658 ) ;
#38849=CARTESIAN_POINT ( 'NONE',  ( 67.20833333333332860, -3.974999999999999201, -6.884901960086287964 ) ) ;
#38867=CARTESIAN_POINT ( 'NONE',  ( 78.95376352523145158, -6.109999999999999432, -3.741295971395163529E-16 ) ) ;
#38868=CARTESIAN_POINT ( 'NONE',  ( 73.72502705046288440, 5.819803920172573974, -5.819803920172573086 ) ) ;
#38887=CARTESIAN_POINT ( 'NONE',  ( 120.6833603837968667, -2.130196079835385170, 7.949999999995403854 ) ) ;
#38892=CARTESIAN_POINT ( 'NONE',  ( 90.05836038379621300, -7.949999999999997513, -2.130196079827425759 ) ) ;
#38906=CARTESIAN_POINT ( 'NONE',  ( 87.79209685856477563, -5.291415217122921177, 3.054999999999999272 ) ) ;
#38924=CARTESIAN_POINT ( 'NONE',  ( 58.89583333333332149, -2.130196079827427091, 7.949999999999998401 ) ) ;
#38927=CARTESIAN_POINT ( 'NONE',  ( 74.66709685856476142, -3.055000000000000160, -5.291415217122921177 ) ) ;
#38943=CARTESIAN_POINT ( 'NONE',  ( 34.05836038379622721, -7.949999999999996625, -2.130196079827426203 ) ) ;
#38954=CARTESIAN_POINT ( 'NONE',  ( 52.87086038379622011, 6.884901960086289741, -3.974999999999993427 ) ) ;
#38982=CARTESIAN_POINT ( 'NONE',  ( 76.70876352523144703, -7.482591942790329030E-16, 6.110000000000001208 ) ) ;
#38990=CARTESIAN_POINT ( 'NONE',  ( 105.4379301918981042, -6.110000000000001208, 1.637169565754158951 ) ) ;
#38992=FACE_OUTER_BOUND ( 'NONE', #5025, .T. ) ;
#39012=CARTESIAN_POINT ( 'NONE',  ( 114.0208333333333144, 7.949999999999998401, 2.130196079827431532 ) ) ;
#39026=CYLINDRICAL_SURFACE ( 'NONE', #92765, 7.950000000000000178 ) ;
#39056=CARTESIAN_POINT ( 'NONE',  ( 117.7666937171295416, -7.949999999999999289, 2.130196079827424427 ) ) ;
#39070=CARTESIAN_POINT ( 'NONE',  ( 84.70833333333332860, -3.974999999999999201, -6.884901960086287964 ) ) ;
#39077=CARTESIAN_POINT ( 'NONE',  ( 30.70419371712955581, -6.884901960086285300, -3.975000000000000089 ) ) ;
#39100=CARTESIAN_POINT ( 'NONE',  ( 99.02126352523144703, -4.472830434245839371, -4.472830434245840259 ) ) ;
#39111=CARTESIAN_POINT ( 'NONE',  ( 104.0370968585647802, -3.054999999999998828, -5.291415217122919401 ) ) ;
#39143=CARTESIAN_POINT ( 'NONE',  ( 114.6829301918981088, -1.637169565754158951, -6.109999999999998543 ) ) ;
#39164=CARTESIAN_POINT ( 'NONE',  ( 29.37043019189811233, -3.055000000000001492, 5.291415217122917625 ) ) ;
#39199=CARTESIAN_POINT ( 'NONE',  ( 105.2037635252314516, 6.109999999999999432, 1.122388791418549108E-15 ) ) ;
#39228=EDGE_CURVE ( 'NONE', #94937, #106661, #72284, .T. ) ;
#39258=CARTESIAN_POINT ( 'NONE',  ( 109.3541666666666714, -2.130196079827425315, -7.950000000000001066 ) ) ;
#39271=CARTESIAN_POINT ( 'NONE',  ( 116.3754301918981042, -5.291415217122920289, -3.055000000000001492 ) ) ;
#39280=CARTESIAN_POINT ( 'NONE',  ( 39.30836038379621300, 7.949999999999997513, 2.130196079827431088 ) ) ;
#39285=CARTESIAN_POINT ( 'NONE',  ( 32.06249999999999289, -5.819803920172572198, -5.819803920172573086 ) ) ;
#39294=CARTESIAN_POINT ( 'NONE',  ( 29.60459685856477563, 1.637169565754164946, -6.109999999999999432 ) ) ;
#39308=CARTESIAN_POINT ( 'NONE',  ( 63.85416666666665719, -2.130196079827425759, -7.950000000000000178 ) ) ;
#39310=CARTESIAN_POINT ( 'NONE',  ( 50.75043019189810423, 3.055000000000002824, -5.291415217122919401 ) ) ;
#39318=CARTESIAN_POINT ( 'NONE',  ( 52.84959685856479439, 6.109999999999996767, 1.637169565754163836 ) ) ;
#39326=VECTOR ( 'NONE', #129637, 1000.000000000000000 ) ;
#39353=CARTESIAN_POINT ( 'NONE',  ( 67.87043019189812298, -3.055000000000001492, 5.291415217122917625 ) ) ;
#39376=EDGE_CURVE ( 'NONE', #128706, #20835, #126010, .T. ) ;
#39407=CARTESIAN_POINT ( 'NONE',  ( 103.0375270504628986, -9.735942053221456900E-16, 7.949999999999998401 ) ) ;
#39428=CARTESIAN_POINT ( 'NONE',  ( 42.64126352523145158, 4.472830434245837594, 4.472830434245841147 ) ) ;
#39455=CARTESIAN_POINT ( 'NONE',  ( 63.51669371712956291, 7.950000000000001066, -2.130196079827421318 ) ) ;
#39460=CARTESIAN_POINT ( 'NONE',  ( 62.25000000000000000, -9.735942053221458872E-16, 7.950000000000000178 ) ) ;
#39467=CARTESIAN_POINT ( 'NONE',  ( 59.20876352523143993, -7.482591942790329030E-16, 6.110000000000001208 ) ) ;
#39515=CARTESIAN_POINT ( 'NONE',  ( 110.0375270504628986, -9.735942053221456900E-16, 7.949999999999998401 ) ) ;
#39520=EDGE_LOOP ( 'NONE', ( #16817, #114596, #100515, #131491, #63965, #102052, #37163, #17945, #118788, #69591, #57437, #39857, #123204, #79300, #140216, #130887, #107822, #43226, #134048, #91395, #3964, #135300, #70008, #118662, #109119, #67990, #84114, #129438, #40287, #41830, #128402, #46327, #76254, #96716, #106671, #60283, #70495, #112274, #83080, #97884, #32263, #109024, #15943, #70674, #12079, #57448, #101541, #125506, #23258, #35447, #127873, #96328, #33409, #61096, #13433, #50280, #2381, #31998, #8970, #137266, #131930, #15536, #107820, #34408, #75955, #128409, #8342 ) ) ;
#39524=CARTESIAN_POINT ( 'NONE',  ( 90.62043019189810877, 3.055000000000001936, -5.291415217122916737 ) ) ;
#39526=CARTESIAN_POINT ( 'NONE',  ( 127.0000000000000000, 0.000000000000000000, 0.000000000000000000 ) ) ;
#39551=CARTESIAN_POINT ( 'NONE',  ( 40.54209685856477563, 5.291415217122923842, -3.054999999999996163 ) ) ;
#39601=CARTESIAN_POINT ( 'NONE',  ( 77.05793019189810877, 6.110000000000001208, -1.637169565754156286 ) ) ;
#39603=CARTESIAN_POINT ( 'NONE',  ( 81.49999999999998579, 0.000000000000000000, -7.950000000000000178 ) ) ;
#39632=CARTESIAN_POINT ( 'NONE',  ( 97.20419371712955581, -6.884901960086285300, -3.975000000000000089 ) ) ;
#39645=CARTESIAN_POINT ( 'NONE',  ( 46.89169371712956291, 2.130196079827421762, 7.950000000000000178 ) ) ;
#39648=CARTESIAN_POINT ( 'NONE',  ( 84.58376352523144703, -6.110000000000001208, -3.741295971395164515E-16 ) ) ;
#39663=CARTESIAN_POINT ( 'NONE',  ( 59.04166666666665719, -3.975000000000002753, 6.884901960086286188 ) ) ;
#39667=CARTESIAN_POINT ( 'NONE',  ( 69.85459685856476142, -1.637169565754161615, 6.110000000000000320 ) ) ;
#39703=LINE ( 'NONE', #50555, #6523 ) ;
#39726=CARTESIAN_POINT ( 'NONE',  ( 68.83376352523143282, 6.110000000000001208, 1.122388791418549305E-15 ) ) ;
#39729=CARTESIAN_POINT ( 'NONE',  ( 104.7087635252314328, -7.482591942790329030E-16, 6.110000000000001208 ) ) ;
#39747=CARTESIAN_POINT ( 'NONE',  ( 114.5583603837962272, -7.949999999999996625, -2.130196079827426203 ) ) ;
#39758=EDGE_CURVE ( 'NONE', #46491, #20610, #41394, .T. ) ;
#39799=CARTESIAN_POINT ( 'NONE',  ( 126.3708603837962130, 6.884901960086289741, -3.974999999999993427 ) ) ;
#39818=CARTESIAN_POINT ( 'NONE',  ( 78.29166666666665719, 3.975000000000003642, -6.884901960086285300 ) ) ;
#39844=CARTESIAN_POINT ( 'NONE',  ( 98.14626352523144703, -4.472830434245840259, 4.472830434245839371 ) ) ;
#39853=CARTESIAN_POINT ( 'NONE',  ( 90.76626352523146579, 4.472830434245839371, -4.472830434245838482 ) ) ;
#39857=ORIENTED_EDGE ( 'NONE', *, *, #2876, .F. ) ;
#39878=CARTESIAN_POINT ( 'NONE',  ( 110.3079301918981088, -6.109999999999998543, 1.637169565754158507 ) ) ;
#39942=CARTESIAN_POINT ( 'NONE',  ( 105.0579301918981230, 6.110000000000001208, -1.637169565754156286 ) ) ;
#39993=CARTESIAN_POINT ( 'NONE',  ( 107.8958333333333144, -2.130196079827427091, 7.949999999999999289 ) ) ;
#40005=CARTESIAN_POINT ( 'NONE',  ( 107.7712635252314186, 4.472830434245839371, 4.472830434245842035 ) ) ;
#40006=ORIENTED_EDGE ( 'NONE', *, *, #79132, .T. ) ;
#40015=CARTESIAN_POINT ( 'NONE',  ( 35.95419371712956291, 6.884901960086283523, 3.975000000000002753 ) ) ;
#40021=CARTESIAN_POINT ( 'NONE',  ( 126.2920968585647614, -5.291415217122921177, 3.054999999999999272 ) ) ;
#40033=CARTESIAN_POINT ( 'NONE',  ( 124.3079301918981230, -6.109999999999998543, 1.637169565754158063 ) ) ;
#40041=FILL_AREA_STYLE ('',( #74062 ) ) ;
#40044=CARTESIAN_POINT ( 'NONE',  ( 45.06293019189811844, 1.637169565754157174, 6.110000000000002984 ) ) ;
#40051=CARTESIAN_POINT ( 'NONE',  ( 49.05793019189810877, 6.110000000000000320, -1.637169565754156064 ) ) ;
#40063=CARTESIAN_POINT ( 'NONE',  ( 45.28752705046289151, 0.000000000000000000, -7.949999999999998401 ) ) ;
#40065=CARTESIAN_POINT ( 'NONE',  ( 150.3000000000000114, 0.000000000000000000, 6.349999999999997868 ) ) ;
#40082=CARTESIAN_POINT ( 'NONE',  ( 52.26626352523145158, 4.472830434245838482, -4.472830434245837594 ) ) ;
#40092=CARTESIAN_POINT ( 'NONE',  ( 34.68749999999999289, -5.819803920172573974, 5.819803920172573086 ) ) ;
#40160=CARTESIAN_POINT ( 'NONE',  ( 43.37043019189810877, -3.055000000000001936, 5.291415217122918513 ) ) ;
#40184=CARTESIAN_POINT ( 'NONE',  ( 66.87086038379622721, 6.884901960086289741, -3.974999999999993427 ) ) ;
#40189=CARTESIAN_POINT ( 'NONE',  ( 52.18749999999999289, -5.819803920172573086, 5.819803920172572198 ) ) ;
#40197=CARTESIAN_POINT ( 'NONE',  ( 52.35459685856476852, -1.637169565754161615, 6.110000000000000320 ) ) ;
#40209=CARTESIAN_POINT ( 'NONE',  ( 100.5583603837962272, -7.949999999999996625, -2.130196079827426203 ) ) ;
#40219=CARTESIAN_POINT ( 'NONE',  ( 77.20376352523145158, 6.109999999999998543, 1.122388791418548911E-15 ) ) ;
#40246=CARTESIAN_POINT ( 'NONE',  ( 84.05793019189810877, 6.110000000000000320, -1.637169565754156064 ) ) ;
#40266=CARTESIAN_POINT ( 'NONE',  ( 123.3083603837962130, 7.949999999999996625, 2.130196079827431088 ) ) ;
#40274=CARTESIAN_POINT ( 'NONE',  ( 37.62543019189811133, 5.291415217122919401, 3.055000000000002824 ) ) ;
#40287=ORIENTED_EDGE ( 'NONE', *, *, #120905, .F. ) ;
#40323=CARTESIAN_POINT ( 'NONE',  ( 74.28709685856478018, 3.054999999999997939, 5.291415217122920289 ) ) ;
#40346=CARTESIAN_POINT ( 'NONE',  ( 94.14169371712957002, -2.130196079827424871, -7.949999999999999289 ) ) ;
#40364=CARTESIAN_POINT ( 'NONE',  ( 89.25043019189810423, 3.055000000000002824, -5.291415217122919401 ) ) ;
#40381=VERTEX_POINT ( 'NONE', #123091 ) ;
#40382=CARTESIAN_POINT ( 'NONE',  ( 73.35459685856476142, -1.637169565754161615, 6.110000000000000320 ) ) ;
#40401=DIRECTION ( 'NONE',  ( 0.000000000000000000, 0.000000000000000000, 1.000000000000000000 ) ) ;
#40421=CARTESIAN_POINT ( 'NONE',  ( 26.99999999999998579, -7.850927237173508821, -1.251176053402193178 ) ) ;
#40423=DIRECTION ( 'NONE',  ( -1.000000000000000000, -0.000000000000000000, -0.000000000000000000 ) ) ;
#40424=CARTESIAN_POINT ( 'NONE',  ( 50.14583333333332149, 2.130196079827356037, -7.950000000000043698 ) ) ;
#40433=CARTESIAN_POINT ( 'NONE',  ( 72.33376352523143282, 6.110000000000001208, 1.122388791418549305E-15 ) ) ;
#40441=CARTESIAN_POINT ( 'NONE',  ( 110.8337635252314470, 6.110000000000001208, 1.122388791418549305E-15 ) ) ;
#40442=( BOUNDED_CURVE ( )  B_SPLINE_CURVE ( 2, ( #110446, #79327, #122770, #69132, #56858, #121339, #90891, #23457, #67726, #135120, #113311, #77170, #35084 ),
 .UNSPECIFIED., .F., .T. ) 
 B_SPLINE_CURVE_WITH_KNOTS ( ( 3, 2, 2, 2, 2, 2, 3 ),
 ( 0.03333333333333336063, 0.03611111111111113547, 0.03888888888888892420, 0.04166666666666669905, 0.04444444444444448084, 0.04722222222222226262, 0.05000000000000004441 ),
 .UNSPECIFIED. ) 
 CURVE ( )  GEOMETRIC_REPRESENTATION_ITEM ( )  RATIONAL_B_SPLINE_CURVE ( ( 0.9999999999999996669, 0.9659258262890686453, 1.000000000000000000, 0.9659258262890683122, 1.000000000000000000, 0.9659258262890683122, 1.000000000000000000, 0.9659258262890683122, 1.000000000000000000, 0.9659258262890683122, 1.000000000000000000, 0.9659258262890677571, 1.000000000000000444 ) ) 
 REPRESENTATION_ITEM ( '' )  );
#40444=AXIS2_PLACEMENT_3D ( 'NONE', #118400, #16967, #85070 ) ;
#40454=AXIS2_PLACEMENT_3D ( 'NONE', #17459, #81328, #126238 ) ;
#40468=CIRCLE ( 'NONE', #38190, 6.349999999999997868 ) ;
#40486=CARTESIAN_POINT ( 'NONE',  ( 27.12543019189810067, 5.291415217122919401, 3.055000000000002824 ) ) ;
#40502=CARTESIAN_POINT ( 'NONE',  ( 92.82919371712955581, -3.975000000000001865, 6.884901960086284411 ) ) ;
#40503=CARTESIAN_POINT ( 'NONE',  ( 121.7041937171295700, -6.884901960086285300, -3.975000000000000089 ) ) ;
#40504=CARTESIAN_POINT ( 'NONE',  ( 48.93336038379622721, 2.130196079827431532, -7.949999999999996625 ) ) ;
#40515=CARTESIAN_POINT ( 'NONE',  ( 80.62500000000000000, -7.950000000000000178, -4.867971026610729436E-16 ) ) ;
#40519=CARTESIAN_POINT ( 'NONE',  ( 91.80836038379622721, 7.949999999999996625, 2.130196079827431088 ) ) ;
#40540=CARTESIAN_POINT ( 'NONE',  ( 106.3129301918981042, -1.637169565754159617, -6.110000000000001208 ) ) ;
#40549=CARTESIAN_POINT ( 'NONE',  ( 95.87043019189810877, -3.055000000000001492, 5.291415217122917625 ) ) ;
#40588=CARTESIAN_POINT ( 'NONE',  ( 36.43750000000000000, 5.819803920172574863, -5.819803920172573086 ) ) ;
#40599=CARTESIAN_POINT ( 'NONE',  ( 28.20376352523144803, 6.109999999999998543, 1.122388791418548911E-15 ) ) ;
#40636=CARTESIAN_POINT ( 'NONE',  ( 89.01626352523143737, -4.472830434245839371, 4.472830434245839371 ) ) ;
#40638=LINE ( 'NONE', #118146, #123122 ) ;
#40682=CARTESIAN_POINT ( 'NONE',  ( 107.3124999999999858, 5.819803920172571310, 5.819803920172575751 ) ) ;
#40693=CARTESIAN_POINT ( 'NONE',  ( 106.1670968585647756, -3.055000000000000160, -5.291415217122921177 ) ) ;
#40701=CARTESIAN_POINT ( 'NONE',  ( 0.000000000000000000, 0.000000000000000000, 7.950000000000000178 ) ) ;
#40709=CARTESIAN_POINT ( 'NONE',  ( 30.02083333333332860, 7.949999999999999289, 2.130196079827431532 ) ) ;
#40719=CARTESIAN_POINT ( 'NONE',  ( 123.8704301918981230, -3.055000000000001492, 5.291415217122917625 ) ) ;
#40726=SURFACE_SIDE_STYLE ('',( #62480 ) ) ;
#40730=CARTESIAN_POINT ( 'NONE',  ( 41.70876352523143993, -7.482591942790329030E-16, 6.110000000000001208 ) ) ;
#40738=CARTESIAN_POINT ( 'NONE',  ( 34.76626352523145158, 4.472830434245839371, -4.472830434245838482 ) ) ;
#40755=DIRECTION ( 'NONE',  ( -1.000000000000000000, -0.000000000000000000, -0.000000000000000000 ) ) ;
#40771=CARTESIAN_POINT ( 'NONE',  ( 61.16209685856478728, -5.291415217122919401, 3.054999999999997939 ) ) ;
#40802=CARTESIAN_POINT ( 'NONE',  ( 123.7245968585647660, -1.637169565754161171, 6.109999999999998543 ) ) ;
#40838=CARTESIAN_POINT ( 'NONE',  ( 38.55793019189810877, 6.110000000000001208, -1.637169565754156286 ) ) ;
#40852=CARTESIAN_POINT ( 'NONE',  ( 81.79166666666667140, 3.975000000000003642, -6.884901960086285300 ) ) ;
#40866=CARTESIAN_POINT ( 'NONE',  ( 65.55836038379622721, -7.949999999999997513, -2.130196079827425759 ) ) ;
#40872=CARTESIAN_POINT ( 'NONE',  ( 59.33333333333333570, -6.884901960086287964, 3.974999999999998312 ) ) ;
#40881=CARTESIAN_POINT ( 'NONE',  ( 45.50043019189810423, -3.055000000000002380, 5.291415217122920289 ) ) ;
#40903=CARTESIAN_POINT ( 'NONE',  ( 66.26626352523145158, 4.472830434245839371, -4.472830434245838482 ) ) ;
#40936=CARTESIAN_POINT ( 'NONE',  ( 83.62043019189812298, 3.055000000000001936, -5.291415217122916737 ) ) ;
#40956=CARTESIAN_POINT ( 'NONE',  ( 31.79209685856476852, -5.291415217122921177, 3.054999999999999272 ) ) ;
#40958=CARTESIAN_POINT ( 'NONE',  ( 46.50000000000000000, 0.000000000000000000, -7.950000000000000178 ) ) ;
#41006=CARTESIAN_POINT ( 'NONE',  ( 65.24543019189810877, -5.291415217122919401, -3.055000000000000604 ) ) ;
#41029=EDGE_CURVE ( 'NONE', #128763, #91210, #51067, .T. ) ;
#41030=CARTESIAN_POINT ( 'NONE',  ( 92.53752705046289861, -9.735942053221456900E-16, 7.949999999999998401 ) ) ;
#41047=CARTESIAN_POINT ( 'NONE',  ( 73.50043019189811844, -3.055000000000002380, 5.291415217122920289 ) ) ;
#41054=CARTESIAN_POINT ( 'NONE',  ( 118.2041937171295700, -6.884901960086285300, -3.975000000000000089 ) ) ;
#41061=CARTESIAN_POINT ( 'NONE',  ( 59.91666666666665719, -6.884901960086287076, -3.975000000000000977 ) ) ;
#41065=AXIS2_PLACEMENT_3D ( 'NONE', #14672, #37130, #58953 ) ;
#41066=CARTESIAN_POINT ( 'NONE',  ( 77.14626352523143282, -4.472830434245840259, 4.472830434245839371 ) ) ;
#41093=ORIENTED_EDGE ( 'NONE', *, *, #138994, .F. ) ;
#41121=CARTESIAN_POINT ( 'NONE',  ( 62.27126352523142572, 4.472830434245838482, 4.472830434245842035 ) ) ;
#41127=CARTESIAN_POINT ( 'NONE',  ( 95.95876352523144703, 0.000000000000000000, -6.110000000000001208 ) ) ;
#41166=CARTESIAN_POINT ( 'NONE',  ( 30.91709685856476497, 3.054999999999998828, 5.291415217122922066 ) ) ;
#41170=CARTESIAN_POINT ( 'NONE',  ( 111.7875270504628986, 0.000000000000000000, -7.949999999999998401 ) ) ;
#41184=CARTESIAN_POINT ( 'NONE',  ( 119.8083603837962272, 7.949999999999997513, 2.130196079827431088 ) ) ;
#41217=CARTESIAN_POINT ( 'NONE',  ( 40.08333333333332860, 6.884901960086290629, -3.974999999999994316 ) ) ;
#41226=CARTESIAN_POINT ( 'NONE',  ( 103.5420968585647756, 5.291415217122923842, -3.054999999999996163 ) ) ;
#41234=CARTESIAN_POINT ( 'NONE',  ( 94.26626352523143737, 4.472830434245839371, -4.472830434245838482 ) ) ;
#41282=( BOUNDED_CURVE ( )  B_SPLINE_CURVE ( 2, ( #6451, #20209, #65921, #64455, #33304, #107923, #110086, #43424, #19520, #31134, #44146, #75351, #142733 ),
 .UNSPECIFIED., .F., .T. ) 
 B_SPLINE_CURVE_WITH_KNOTS ( ( 3, 2, 2, 2, 2, 2, 3 ),
 ( 0.6666666666666666297, 0.6694444444444443976, 0.6722222222222222765, 0.6750000000000000444, 0.6777777777777779233, 0.6805555555555556912, 0.6833333333333334592 ),
 .UNSPECIFIED. ) 
 CURVE ( )  GEOMETRIC_REPRESENTATION_ITEM ( )  RATIONAL_B_SPLINE_CURVE ( ( 1.000000000000000000, 0.9659258262890683122, 1.000000000000000000, 0.9659258262890683122, 1.000000000000000000, 0.9659258262890683122, 1.000000000000000000, 0.9659258262890683122, 1.000000000000000000, 0.9659258262890683122, 1.000000000000000000, 0.9659258262890669799, 1.000000000000001332 ) ) 
 REPRESENTATION_ITEM ( '' )  );
#41284=CARTESIAN_POINT ( 'NONE',  ( 28.64126352523144092, 4.472830434245835818, 4.472830434245840259 ) ) ;
#41295=ADVANCED_FACE ( 'NONE', ( #88644 ), #90879, .T. ) ;
#41316=CARTESIAN_POINT ( 'NONE',  ( 92.95376352523145158, -6.109999999999999432, -3.741295971395163529E-16 ) ) ;
#41339=AXIS2_PLACEMENT_3D ( 'NONE', #100481, #80875, #112071 ) ;
#41357=CARTESIAN_POINT ( 'NONE',  ( 47.95833333333332860, 3.974999999999997424, 6.884901960086288852 ) ) ;
#41371=CARTESIAN_POINT ( 'NONE',  ( 113.2916666666666714, 3.975000000000003642, -6.884901960086285300 ) ) ;
#41387=CARTESIAN_POINT ( 'NONE',  ( 103.1045968585647756, 1.637169565754164946, -6.109999999999999432 ) ) ;
#41394=LINE ( 'NONE', #85602, #135662 ) ;
#41401=CARTESIAN_POINT ( 'NONE',  ( 127.0212635252314328, -4.472830434245839371, -4.472830434245840259 ) ) ;
#41411=CARTESIAN_POINT ( 'NONE',  ( 120.3704301918981230, -3.055000000000001492, 5.291415217122917625 ) ) ;
#41412=B_SPLINE_CURVE_WITH_KNOTS ( 'NONE', 3,
 ( #113547, #36708, #57077, #92506, #36034, #103379, #134630, #24414, #136733, #78099, #78809, #70117, #13509, #22947, #14250, #58534, #112156, #102703, #12807, #67211, #57790, #111410, #101976, #2642, #1208, #80954, #133896, #45490, #89667, #34587, #46941, #123023, #23701, #125152 ),
 .UNSPECIFIED., .F., .F.,
 ( 4, 2, 2, 2, 2, 2, 2, 2, 2, 2, 2, 2, 2, 2, 2, 2, 4 ),
 ( 0.000000000000000000, 0.0008672315150799628312, 0.001734463030159925662, 0.002601694545239888277, 0.003468926060319849156, 0.004336157575399808735, 0.005203389090479769614, 0.006070620605559729627, 0.006937852120639688772, 0.007805083635719650519, 0.008672315150799608796, 0.009539546665879569676, 0.01040677818095952882, 0.01127400969603948970, 0.01214124121111944711, 0.01300847272619940452, 0.01387570424127936193 ),
 .UNSPECIFIED. ) ;
#41417=CARTESIAN_POINT ( 'NONE',  ( 71.24586038379622721, 3.974999999999996980, 6.884901960086287964 ) ) ;
#41422=CARTESIAN_POINT ( 'NONE',  ( 50.31293019189810423, -1.637169565754159617, -6.110000000000001208 ) ) ;
#41430=CARTESIAN_POINT ( 'NONE',  ( 41.62043019189810877, 3.055000000000001936, -5.291415217122916737 ) ) ;
#41455=CARTESIAN_POINT ( 'NONE',  ( 54.45376352523144448, -6.109999999999998543, -3.741295971395162543E-16 ) ) ;
#41494=CARTESIAN_POINT ( 'NONE',  ( 115.5579301918981088, 6.110000000000001208, -1.637169565754156286 ) ) ;
#41512=CARTESIAN_POINT ( 'NONE',  ( 0.000000000000000000, 0.000000000000000000, 0.000000000000000000 ) ) ;
#41526=CARTESIAN_POINT ( 'NONE',  ( 37.39126352523143737, -4.472830434245839371, -4.472830434245839371 ) ) ;
#41547=CARTESIAN_POINT ( 'NONE',  ( 82.22916666666665719, 7.950000000000001954, -2.130196079827421762 ) ) ;
#41559=CARTESIAN_POINT ( 'NONE',  ( 58.99586038379622721, -3.974999999999998312, -6.884901960086286188 ) ) ;
#41565=CARTESIAN_POINT ( 'NONE',  ( 54.22916666666666430, 7.950000000000001954, -2.130196079827421762 ) ) ;
#41575=CARTESIAN_POINT ( 'NONE',  ( 46.95876352523143993, 0.000000000000000000, -6.110000000000001208 ) ) ;
#41583=CARTESIAN_POINT ( 'NONE',  ( 80.87086038379622721, 6.884901960086289741, -3.974999999999993427 ) ) ;
#41592=CARTESIAN_POINT ( 'NONE',  ( 83.56293019189811844, 1.637169565754157174, 6.110000000000002984 ) ) ;
#41605=CARTESIAN_POINT ( 'NONE',  ( 69.76626352523143737, 4.472830434245839371, -4.472830434245838482 ) ) ;
#41612=CARTESIAN_POINT ( 'NONE',  ( 0.000000000000000000, 0.000000000000000000, 0.000000000000000000 ) ) ;
#41625=FACE_OUTER_BOUND ( 'NONE', #109939, .T. ) ;
#41632=CARTESIAN_POINT ( 'NONE',  ( 81.43293019189810877, 1.637169565754156508, 6.110000000000000320 ) ) ;
#41655=CARTESIAN_POINT ( 'NONE',  ( 122.7250270504628844, 5.819803920172573974, -5.819803920172573086 ) ) ;
#41663=CARTESIAN_POINT ( 'NONE',  ( 36.02126352523143282, -4.472830434245838482, -4.472830434245840259 ) ) ;
#41702=CARTESIAN_POINT ( 'NONE',  ( 66.91666666666667140, -6.884901960086287076, -3.975000000000000977 ) ) ;
#41721=CARTESIAN_POINT ( 'NONE',  ( 61.16209685856478728, -5.291415217122919401, 3.054999999999998384 ) ) ;
#41739=CARTESIAN_POINT ( 'NONE',  ( 106.7291666666666572, 7.950000000000001954, -2.130196079827421762 ) ) ;
#41749=CARTESIAN_POINT ( 'NONE',  ( 84.07919371712955581, 3.975000000000002753, -6.884901960086283523 ) ) ;
#41764=CARTESIAN_POINT ( 'NONE',  ( 78.75043019189810423, 3.055000000000002824, -5.291415217122919401 ) ) ;
#41783=CARTESIAN_POINT ( 'NONE',  ( 60.20833333333333570, -3.974999999999999201, -6.884901960086287964 ) ) ;
#41787=CARTESIAN_POINT ( 'NONE',  ( 70.72959685856477563, -6.110000000000000320, -1.637169565754161393 ) ) ;
#41814=ORIENTED_EDGE ( 'NONE', *, *, #54368, .T. ) ;
#41825=CARTESIAN_POINT ( 'NONE',  ( 58.12086038379622721, -6.884901960086286188, 3.974999999999997424 ) ) ;
#41830=ORIENTED_EDGE ( 'NONE', *, *, #139933, .F. ) ;
#41841=CARTESIAN_POINT ( 'NONE',  ( 64.02126352523143282, -4.472830434245838482, -4.472830434245840259 ) ) ;
#41850=CARTESIAN_POINT ( 'NONE',  ( 102.5212635252314328, -4.472830434245838482, -4.472830434245840259 ) ) ;
#41869=CARTESIAN_POINT ( 'NONE',  ( 124.1620968585647944, -5.291415217122919401, 3.054999999999997939 ) ) ;
#41886=CARTESIAN_POINT ( 'NONE',  ( 38.91666666666665719, -6.884901960086287076, -3.975000000000000977 ) ) ;
#41901=CARTESIAN_POINT ( 'NONE',  ( 29.45876352523143993, 0.000000000000000000, -6.110000000000001208 ) ) ;
#41924=CARTESIAN_POINT ( 'NONE',  ( 110.0375270504628986, -9.735942053221456900E-16, 7.949999999999998401 ) ) ;
#41940=DIRECTION ( 'NONE',  ( -1.000000000000000000, -0.000000000000000000, -0.000000000000000000 ) ) ;
#41949=CARTESIAN_POINT ( 'NONE',  ( 93.31249999999998579, 5.819803920172571310, 5.819803920172576639 ) ) ;
#41962=CARTESIAN_POINT ( 'NONE',  ( 101.7920968585647756, -5.291415217122921177, 3.054999999999999272 ) ) ;
#41969=CARTESIAN_POINT ( 'NONE',  ( 48.39583333333332860, -2.130196079827427091, 7.949999999999998401 ) ) ;
#41974=CARTESIAN_POINT ( 'NONE',  ( 98.05793019189812298, 6.110000000000000320, -1.637169565754156064 ) ) ;
#41981=CARTESIAN_POINT ( 'NONE',  ( 115.9166666666666714, -6.884901960086287076, -3.975000000000000977 ) ) ;
#42030=CARTESIAN_POINT ( 'NONE',  ( 28.78709685856477307, 3.054999999999997495, 5.291415217122919401 ) ) ;
#42068=CARTESIAN_POINT ( 'NONE',  ( 88.28709685856478018, 3.054999999999997939, 5.291415217122920289 ) ) ;
#42069=CARTESIAN_POINT ( 'NONE',  ( 10.32500000000000107, -8.432637487761466488, -4.375000000000001776 ) ) ;
#42078=VECTOR ( 'NONE', #52576, 1000.000000000000000 ) ;
#42099=ORIENTED_EDGE ( 'NONE', *, *, #52154, .T. ) ;
#42111=CARTESIAN_POINT ( 'NONE',  ( 46.50000000000000000, 0.000000000000000000, -7.950000000000000178 ) ) ;
#42122=CARTESIAN_POINT ( 'NONE',  ( 113.5833333333333428, 6.884901960086290629, -3.974999999999994316 ) ) ;
#42136=CARTESIAN_POINT ( 'NONE',  ( 104.5629301918981184, 1.637169565754157174, 6.110000000000002984 ) ) ;
#42149=CARTESIAN_POINT ( 'NONE',  ( 27.54166666666665719, -3.975000000000002753, 6.884901960086286188 ) ) ;
#42159=CARTESIAN_POINT ( 'NONE',  ( 123.4329301918981088, 1.637169565754156508, 6.110000000000000320 ) ) ;
#42164=CARTESIAN_POINT ( 'NONE',  ( 69.93336038379619879, 2.130196079827431532, -7.949999999999996625 ) ) ;
#42168=CARTESIAN_POINT ( 'NONE',  ( 50.45876352523143282, 0.000000000000000000, -6.110000000000001208 ) ) ;
#42174=CARTESIAN_POINT ( 'NONE',  ( 66.28752705046289861, 0.000000000000000000, -7.949999999999998401 ) ) ;
#42175=( BOUNDED_CURVE ( )  B_SPLINE_CURVE ( 2, ( #68181, #143543, #98605, #21770, #43519, #121773, #87741, #23163, #12308, #45001, #1411, #45696, #89865 ),
 .UNSPECIFIED., .F., .T. ) 
 B_SPLINE_CURVE_WITH_KNOTS ( ( 3, 2, 2, 2, 2, 2, 3 ),
 ( 0.1499999999999999944, 0.1527777777777777901, 0.1555555555555555580, 0.1583333333333333259, 0.1611111111111111216, 0.1638888888888888895, 0.1666666666666666574 ),
 .UNSPECIFIED. ) 
 CURVE ( )  GEOMETRIC_REPRESENTATION_ITEM ( )  RATIONAL_B_SPLINE_CURVE ( ( 1.000000000000000000, 0.9659258262890683122, 1.000000000000000000, 0.9659258262890683122, 1.000000000000000000, 0.9659258262890683122, 1.000000000000000000, 0.9659258262890683122, 1.000000000000000000, 0.9659258262890683122, 1.000000000000000000, 0.9659258262890683122, 1.000000000000000000 ) ) 
 REPRESENTATION_ITEM ( '' )  );
#42176=CARTESIAN_POINT ( 'NONE',  ( 36.66209685856478018, -5.291415217122919401, 3.054999999999997939 ) ) ;
#42205=CARTESIAN_POINT ( 'NONE',  ( 58.24543019189810877, -5.291415217122918513, -3.055000000000000160 ) ) ;
#42244=CARTESIAN_POINT ( 'NONE',  ( 124.7454301918981230, -5.291415217122919401, -3.055000000000000604 ) ) ;
#42285=CARTESIAN_POINT ( 'NONE',  ( 36.07876352523144448, -7.482591942790327058E-16, 6.109999999999999432 ) ) ;
#42313=CARTESIAN_POINT ( 'NONE',  ( 59.28752705046289151, 0.000000000000000000, -7.949999999999998401 ) ) ;
#42318=CARTESIAN_POINT ( 'NONE',  ( 58.16666666666665719, 6.884901960086285300, 3.975000000000003642 ) ) ;
#42324=CARTESIAN_POINT ( 'NONE',  ( 46.81293019189811133, -1.637169565754159617, -6.110000000000001208 ) ) ;
#42337=ADVANCED_FACE ( 'NONE', ( #61819 ), #105976, .T. ) ;
#42341=CARTESIAN_POINT ( 'NONE',  ( 84.14626352523144703, -4.472830434245840259, 4.472830434245838482 ) ) ;
#42349=CARTESIAN_POINT ( 'NONE',  ( 88.16252705046289861, 7.949999999999998401, 1.460391307983218338E-15 ) ) ;
#42350=CARTESIAN_POINT ( 'NONE',  ( 63.78709685856477307, 3.054999999999997495, 5.291415217122919401 ) ) ;
#42381=CARTESIAN_POINT ( 'NONE',  ( 87.70376352523146579, 6.109999999999998543, 1.122388791418548911E-15 ) ) ;
#42412=CARTESIAN_POINT ( 'NONE',  ( 37.04209685856476852, 5.291415217122923842, -3.054999999999996163 ) ) ;
#42428=CARTESIAN_POINT ( 'NONE',  ( 115.1416937171295558, -2.130196079827424871, -7.949999999999998401 ) ) ;
#42469=CARTESIAN_POINT ( 'NONE',  ( 65.39126352523145158, -4.472830434245839371, -4.472830434245839371 ) ) ;
#42492=CARTESIAN_POINT ( 'NONE',  ( 83.49586038379622721, -3.974999999999998312, -6.884901960086286188 ) ) ;
#42505=CARTESIAN_POINT ( 'NONE',  ( 79.77126352523144703, 4.472830434245839371, 4.472830434245842035 ) ) ;
#42525=CARTESIAN_POINT ( 'NONE',  ( 60.52126352523143282, -4.472830434245839371, -4.472830434245840259 ) ) ;
#42529=FACE_OUTER_BOUND ( 'NONE', #127335, .T. ) ;
#42558=CARTESIAN_POINT ( 'NONE',  ( 109.2870968585647944, 3.054999999999997495, 5.291415217122919401 ) ) ;
#42566=EDGE_CURVE ( 'NONE', #133461, #98838, #93355, .T. ) ;
#42578=CARTESIAN_POINT ( 'NONE',  ( 51.45833333333332860, 3.974999999999997424, 6.884901960086288852 ) ) ;
#42586=CARTESIAN_POINT ( 'NONE',  ( 62.70876352523143993, -7.482591942790329030E-16, 6.110000000000001208 ) ) ;
#42592=CARTESIAN_POINT ( 'NONE',  ( 97.56293019189810423, 1.637169565754157174, 6.110000000000002984 ) ) ;
#42601=CARTESIAN_POINT ( 'NONE',  ( 77.22502705046287019, 5.819803920172573974, -5.819803920172573086 ) ) ;
#42607=CARTESIAN_POINT ( 'NONE',  ( 118.3287635252314658, 0.000000000000000000, -6.109999999999998543 ) ) ;
#42626=CARTESIAN_POINT ( 'NONE',  ( 0.000000000000000000, 0.000000000000000000, 0.000000000000000000 ) ) ;
#42635=CARTESIAN_POINT ( 'NONE',  ( 27.85459685856477208, -1.637169565754161615, 6.110000000000000320 ) ) ;
#42645=CARTESIAN_POINT ( 'NONE',  ( 0.000000000000000000, 0.000000000000000000, 0.000000000000000000 ) ) ;
#42653=CARTESIAN_POINT ( 'NONE',  ( 93.99586038379622721, -3.974999999999998312, -6.884901960086286188 ) ) ;
#42654=CARTESIAN_POINT ( 'NONE',  ( 116.7458603837962272, 3.974999999999996980, 6.884901960086287964 ) ) ;
#42694=CARTESIAN_POINT ( 'NONE',  ( 91.58376352523144703, -6.110000000000001208, -3.741295971395164515E-16 ) ) ;
#42704=CARTESIAN_POINT ( 'NONE',  ( 92.22459685856479439, -1.637169565754160949, 6.109999999999997655 ) ) ;
#42734=EDGE_CURVE ( 'NONE', #31006, #40381, #59540, .T. ) ;
#42738=CARTESIAN_POINT ( 'NONE',  ( 119.5624999999999858, -5.819803920172573086, -5.819803920172573974 ) ) ;
#42785=CARTESIAN_POINT ( 'NONE',  ( 95.57876352523145158, -7.482591942790327058E-16, 6.109999999999999432 ) ) ;
#42810=ORIENTED_EDGE ( 'NONE', *, *, #12340, .F. ) ;
#42834=CARTESIAN_POINT ( 'NONE',  ( 98.27083333333332860, -7.949999999999999289, -2.130196079827426203 ) ) ;
#42841=CARTESIAN_POINT ( 'NONE',  ( 90.10416666666668561, 2.130196079827460398, 7.949999999999981526 ) ) ;
#42856=CARTESIAN_POINT ( 'NONE',  ( 29.53752705046289151, -9.735942053221456900E-16, 7.949999999999998401 ) ) ;
#42864=CARTESIAN_POINT ( 'NONE',  ( 25.35416666666666430, -2.130196079827425315, -7.950000000000001066 ) ) ;
#42877=CARTESIAN_POINT ( 'NONE',  ( 121.2454301918981230, -5.291415217122918513, -3.055000000000000160 ) ) ;
#42882=( NAMED_UNIT ( * ) SI_UNIT ( $, .STERADIAN. ) SOLID_ANGLE_UNIT ( ) );
#42886=CARTESIAN_POINT ( 'NONE',  ( 43.60459685856476852, 1.637169565754164946, -6.109999999999999432 ) ) ;
#42893=CARTESIAN_POINT ( 'NONE',  ( 37.53709685856478018, -3.054999999999998828, -5.291415217122919401 ) ) ;
#42919=CARTESIAN_POINT ( 'NONE',  ( 59.55793019189811588, 6.110000000000000320, -1.637169565754156064 ) ) ;
#42928=FACE_OUTER_BOUND ( 'NONE', #6768, .T. ) ;
#42936=EDGE_LOOP ( 'NONE', ( #31021, #72614, #90313, #130181 ) ) ;
#42942=DIRECTION ( 'NONE',  ( 0.000000000000000000, 0.000000000000000000, -1.000000000000000000 ) ) ;
#42955=CARTESIAN_POINT ( 'NONE',  ( 119.0579301918981230, 6.110000000000001208, -1.637169565754156286 ) ) ;
#42964=CARTESIAN_POINT ( 'NONE',  ( 75.03752705046288440, -9.735942053221456900E-16, 7.949999999999998401 ) ) ;
#42993=CARTESIAN_POINT ( 'NONE',  ( 33.01626352523145158, -4.472830434245839371, 4.472830434245839371 ) ) ;
#43015=CARTESIAN_POINT ( 'NONE',  ( 54.91252705046288440, -7.949999999999998401, -4.867971026610728450E-16 ) ) ;
#43021=CARTESIAN_POINT ( 'NONE',  ( 59.04166666666665719, -3.975000000000002753, 6.884901960086286188 ) ) ;
#43024=EDGE_CURVE ( 'NONE', #75139, #53682, #93808, .T. ) ;
#43033=CARTESIAN_POINT ( 'NONE',  ( 44.33376352523143993, 6.110000000000001208, 1.122388791418549305E-15 ) ) ;
#43049=CARTESIAN_POINT ( 'NONE',  ( 85.45876352523143282, 0.000000000000000000, -6.110000000000001208 ) ) ;
#43061=CARTESIAN_POINT ( 'NONE',  ( 71.66209685856478018, -5.291415217122919401, 3.054999999999997939 ) ) ;
#43071=ORIENTED_EDGE ( 'NONE', *, *, #10376, .T. ) ;
#43083=CARTESIAN_POINT ( 'NONE',  ( 50.68336038379622721, -2.130196079827426203, 7.949999999999996625 ) ) ;
#43088=CARTESIAN_POINT ( 'NONE',  ( 80.12043019189810877, 3.055000000000001936, -5.291415217122916737 ) ) ;
#43092=ORIENTED_EDGE ( 'NONE', *, *, #111440, .T. ) ;
#43112=CARTESIAN_POINT ( 'NONE',  ( 39.81293019189809712, -1.637169565754159617, -6.110000000000001208 ) ) ;
#43164=CARTESIAN_POINT ( 'NONE',  ( 66.12043019189812298, 3.055000000000002380, -5.291415217122917625 ) ) ;
#43189=CARTESIAN_POINT ( 'NONE',  ( 82.18336038379619879, -2.130196079827426203, 7.949999999999997513 ) ) ;
#43195=CARTESIAN_POINT ( 'NONE',  ( 84.41666666666667140, -6.884901960086287076, -3.975000000000000977 ) ) ;
#43206=CARTESIAN_POINT ( 'NONE',  ( 74.66709685856476142, -3.055000000000000160, -5.291415217122921177 ) ) ;
#43225=CARTESIAN_POINT ( 'NONE',  ( 66.79209685856477563, -5.291415217122921177, 3.054999999999999272 ) ) ;
#43226=ORIENTED_EDGE ( 'NONE', *, *, #117113, .F. ) ;
#43261=CARTESIAN_POINT ( 'NONE',  ( 115.8495968585647802, 6.109999999999996767, 1.637169565754163836 ) ) ;
#43281=CARTESIAN_POINT ( 'NONE',  ( 67.66709685856477563, -3.055000000000000160, -5.291415217122921177 ) ) ;
#43287=CARTESIAN_POINT ( 'NONE',  ( 99.89626352523141861, 4.472830434245840259, -4.472830434245838482 ) ) ;
#43299=CARTESIAN_POINT ( 'NONE',  ( 122.1204301918981230, 3.055000000000001936, -5.291415217122916737 ) ) ;
#43316=CARTESIAN_POINT ( 'NONE',  ( 39.49999999999999289, 0.000000000000000000, -7.950000000000000178 ) ) ;
#43326=CARTESIAN_POINT ( 'NONE',  ( 31.79209685856476852, -5.291415217122921177, 3.054999999999999272 ) ) ;
#43346=CARTESIAN_POINT ( 'NONE',  ( 93.12086038379622721, -6.884901960086286188, 3.974999999999997424 ) ) ;
#43348=CARTESIAN_POINT ( 'NONE',  ( 111.2041937171295558, -6.884901960086285300, -3.975000000000000089 ) ) ;
#43375=DIRECTION ( 'NONE',  ( -1.000000000000000000, -0.000000000000000000, -0.000000000000000000 ) ) ;
#43386=CARTESIAN_POINT ( 'NONE',  ( 91.29209685856477563, -5.291415217122921177, 3.054999999999999272 ) ) ;
#43397=CARTESIAN_POINT ( 'NONE',  ( 85.66209685856478018, -5.291415217122919401, 3.054999999999997939 ) ) ;
#43401=CARTESIAN_POINT ( 'NONE',  ( 116.3541666666666998, -2.130196079827387567, -7.950000000000023270 ) ) ;
#43409=FACE_OUTER_BOUND ( 'NONE', #71471, .T. ) ;
#43419=ORIENTED_EDGE ( 'NONE', *, *, #125135, .F. ) ;
#43424=CARTESIAN_POINT ( 'NONE',  ( 55.97916666666666430, -7.950000000000000178, 2.130196079827424427 ) ) ;
#43435=CARTESIAN_POINT ( 'NONE',  ( 117.0375270504628986, -9.735942053221456900E-16, 7.949999999999998401 ) ) ;
#43478=CARTESIAN_POINT ( 'NONE',  ( 93.39126352523143737, -4.472830434245839371, -4.472830434245839371 ) ) ;
#43479=CARTESIAN_POINT ( 'NONE',  ( 10.03605673236671869, -8.432637487761464712, -4.375000000000002665 ) ) ;
#43519=CARTESIAN_POINT ( 'NONE',  ( 110.6666666666666572, 6.884901960086285300, 3.975000000000003642 ) ) ;
#43524=CARTESIAN_POINT ( 'NONE',  ( 105.1250000000000000, -7.950000000000000178, -4.867971026610729436E-16 ) ) ;
#43547=CARTESIAN_POINT ( 'NONE',  ( 26.91252705046288796, -7.949999999999998401, -4.867971026610728450E-16 ) ) ;
#43551=CARTESIAN_POINT ( 'NONE',  ( 121.4795968585647614, 6.109999999999999432, 1.637169565754164280 ) ) ;
#43561=CARTESIAN_POINT ( 'NONE',  ( 115.2662635252314374, 4.472830434245839371, -4.472830434245838482 ) ) ;
#43569=CARTESIAN_POINT ( 'NONE',  ( 34.70876352523143282, -7.482591942790329030E-16, 6.110000000000001208 ) ) ;
#43576=CARTESIAN_POINT ( 'NONE',  ( 38.70376352523144448, 6.109999999999998543, 1.122388791418548911E-15 ) ) ;
#43595=DIRECTION ( 'NONE',  ( 0.000000000000000000, 0.000000000000000000, 1.000000000000000000 ) ) ;
#43603=CARTESIAN_POINT ( 'NONE',  ( 49.49543019189811588, 5.291415217122916737, 3.055000000000001936 ) ) ;
#43645=CARTESIAN_POINT ( 'NONE',  ( 116.5787635252314516, -7.482591942790327058E-16, 6.109999999999999432 ) ) ;
#43651=CARTESIAN_POINT ( 'NONE',  ( 66.57919371712955581, 3.975000000000002753, -6.884901960086283523 ) ) ;
#43656=( BOUNDED_CURVE ( )  B_SPLINE_CURVE ( 2, ( #76423, #131508, #132244, #74277, #88733, #32190, #85845, #65573, #32935, #99558, #31481, #43083, #43781 ),
 .UNSPECIFIED., .F., .T. ) 
 B_SPLINE_CURVE_WITH_KNOTS ( ( 3, 2, 2, 2, 2, 2, 3 ),
 ( 0.7333333333333332815, 0.7361111111111111605, 0.7388888888888889284, 0.7416666666666666963, 0.7444444444444444642, 0.7472222222222222321, 0.7500000000000000000 ),
 .UNSPECIFIED. ) 
 CURVE ( )  GEOMETRIC_REPRESENTATION_ITEM ( )  RATIONAL_B_SPLINE_CURVE ( ( 1.000000000000000000, 0.9659258262890683122, 1.000000000000000000, 0.9659258262890683122, 1.000000000000000000, 0.9659258262890683122, 1.000000000000000000, 0.9659258262890683122, 1.000000000000000000, 0.9659258262890683122, 1.000000000000000000, 0.9659258262890683122, 1.000000000000000000 ) ) 
 REPRESENTATION_ITEM ( '' )  );
#43687=CARTESIAN_POINT ( 'NONE',  ( 37.68293019189810167, -1.637169565754159173, -6.109999999999999432 ) ) ;
#43693=CARTESIAN_POINT ( 'NONE',  ( 125.9791666666666572, -7.950000000000001066, 2.130196079827424427 ) ) ;
#43705=CARTESIAN_POINT ( 'NONE',  ( 120.6045968585647614, 1.637169565754164946, -6.109999999999999432 ) ) ;
#43714=CARTESIAN_POINT ( 'NONE',  ( 52.57919371712956291, 3.975000000000002753, -6.884901960086283523 ) ) ;
#43719=CARTESIAN_POINT ( 'NONE',  ( 41.24999999999999289, -9.735942053221458872E-16, 7.950000000000000178 ) ) ;
#43726=CARTESIAN_POINT ( 'NONE',  ( 45.79209685856476852, -5.291415217122921177, 3.054999999999999272 ) ) ;
#43744=CARTESIAN_POINT ( 'NONE',  ( 77.87543019189810423, -5.291415217122920289, -3.055000000000001492 ) ) ;
#43755=CARTESIAN_POINT ( 'NONE',  ( 67.14126352523145158, 4.472830434245836706, 4.472830434245840259 ) ) ;
#43781=CARTESIAN_POINT ( 'NONE',  ( 50.53752705046289861, -9.735942053221456900E-16, 7.949999999999998401 ) ) ;
#43789=CARTESIAN_POINT ( 'NONE',  ( 79.82876352523145158, 0.000000000000000000, -6.109999999999998543 ) ) ;
#43809=EDGE_LOOP ( 'NONE', ( #44951, #83109, #99205, #126001, #99260 ) ) ;
#43816=CARTESIAN_POINT ( 'NONE',  ( 89.32919371712955581, -3.975000000000001865, 6.884901960086284411 ) ) ;
#43873=CARTESIAN_POINT ( 'NONE',  ( 63.20376352523145158, 6.109999999999999432, 1.122388791418549108E-15 ) ) ;
#43874=DIRECTION ( 'NONE',  ( -1.000000000000000000, -0.000000000000000000, -0.000000000000000000 ) ) ;
#43900=CARTESIAN_POINT ( 'NONE',  ( 86.99586038379622721, -3.974999999999998312, -6.884901960086286188 ) ) ;
#43904=CARTESIAN_POINT ( 'NONE',  ( 70.70833333333332860, -3.974999999999999201, -6.884901960086287964 ) ) ;
#43915=CARTESIAN_POINT ( 'NONE',  ( 72.04209685856477563, 5.291415217122923842, -3.054999999999996163 ) ) ;
#43924=CARTESIAN_POINT ( 'NONE',  ( 127.0000000000000568, 1.764297610274628392, 6.170334904552290389 ) ) ;
#43932=CARTESIAN_POINT ( 'NONE',  ( 66.64626352523144703, -4.472830434245840259, 4.472830434245839371 ) ) ;
#43936=CARTESIAN_POINT ( 'NONE',  ( 124.7666937171295274, -7.949999999999998401, 2.130196079827423983 ) ) ;
#43963=CARTESIAN_POINT ( 'NONE',  ( 114.9745968585647802, 1.637169565754164280, -6.109999999999996767 ) ) ;
#43976=CARTESIAN_POINT ( 'NONE',  ( 37.60416666666665719, 2.130196079827498146, 7.949999999999958433 ) ) ;
#43990=CARTESIAN_POINT ( 'NONE',  ( 63.72959685856477563, -6.110000000000000320, -1.637169565754161393 ) ) ;
#43996=CARTESIAN_POINT ( 'NONE',  ( 100.4795968585647614, 6.109999999999999432, 1.637169565754164280 ) ) ;
#44008=CARTESIAN_POINT ( 'NONE',  ( 10.32500000000000107, -9.500000000000001776, -4.375000000000001776 ) ) ;
#44012=CARTESIAN_POINT ( 'NONE',  ( 122.4120968585647802, 5.291415217122921177, -3.054999999999994831 ) ) ;
#44033=CARTESIAN_POINT ( 'NONE',  ( 58.60416666666665719, 2.130196079827422206, 7.950000000000001954 ) ) ;
#44061=EDGE_LOOP ( 'NONE', ( #121102, #121151 ) ) ;
#44064=CARTESIAN_POINT ( 'NONE',  ( 116.1625270504628986, 7.949999999999998401, 1.460391307983218338E-15 ) ) ;
#44107=CARTESIAN_POINT ( 'NONE',  ( 91.14626352523144703, -4.472830434245840259, 4.472830434245839371 ) ) ;
#44116=CARTESIAN_POINT ( 'NONE',  ( 82.30793019189809456, -6.109999999999998543, 1.637169565754158063 ) ) ;
#44146=CARTESIAN_POINT ( 'NONE',  ( 55.54166666666665719, -3.975000000000002753, 6.884901960086286188 ) ) ;
#44150=AXIS2_PLACEMENT_3D ( 'NONE', #27784, #138712, #83631 ) ;
#44154=CARTESIAN_POINT ( 'NONE',  ( 118.5416666666666714, -3.975000000000002753, 6.884901960086286188 ) ) ;
#44173=CARTESIAN_POINT ( 'NONE',  ( 123.0837635252314470, -6.110000000000001208, -3.741295971395164515E-16 ) ) ;
#44197=CARTESIAN_POINT ( 'NONE',  ( 106.9750270504628986, -5.819803920172573086, 5.819803920172573086 ) ) ;
#44211=CARTESIAN_POINT ( 'NONE',  ( 86.97459685856479439, 1.637169565754164280, -6.109999999999997655 ) ) ;
#44213=CARTESIAN_POINT ( 'NONE',  ( 5.950517365466079234, -9.499761739870839605, 0.3008884456578363453 ) ) ;
#44262=CARTESIAN_POINT ( 'NONE',  ( 100.6041666666666430, 2.130196079827422206, 7.950000000000001954 ) ) ;
#44268=DIRECTION ( 'NONE',  ( 0.000000000000000000, 0.000000000000000000, -1.000000000000000000 ) ) ;
#44291=CARTESIAN_POINT ( 'NONE',  ( 125.1254301918981184, 5.291415217122919401, 3.055000000000002824 ) ) ;
#44301=CARTESIAN_POINT ( 'NONE',  ( 113.3704301918981230, -3.055000000000001492, 5.291415217122917625 ) ) ;
#44310=CARTESIAN_POINT ( 'NONE',  ( 36.02126352523142572, -4.472830434245839371, -4.472830434245840259 ) ) ;
#44311=EDGE_CURVE ( 'NONE', #82006, #33848, #109780, .T. ) ;
#44316=EDGE_CURVE ( 'NONE', #83402, #121702, #74350, .T. ) ;
#44320=CARTESIAN_POINT ( 'NONE',  ( 34.03709685856478018, -3.054999999999998828, -5.291415217122919401 ) ) ;
#44331=CARTESIAN_POINT ( 'NONE',  ( 78.68336038379622721, -2.130196079827426203, 7.949999999999996625 ) ) ;
#44341=DIRECTION ( 'NONE',  ( -1.000000000000000000, -0.000000000000000000, -0.000000000000000000 ) ) ;
#44352=CARTESIAN_POINT ( 'NONE',  ( 45.26626352523144448, 4.472830434245838482, -4.472830434245837594 ) ) ;
#44394=CARTESIAN_POINT ( 'NONE',  ( 108.4120968585647944, 5.291415217122922066, -3.054999999999995275 ) ) ;
#44417=VERTEX_POINT ( 'NONE', #110481 ) ;
#44438=CARTESIAN_POINT ( 'NONE',  ( 28.20376352523144803, 6.109999999999999432, 1.122388791418549108E-15 ) ) ;
#44451=DIRECTION ( 'NONE',  ( 0.000000000000000000, 0.000000000000000000, 1.000000000000000000 ) ) ;
#44453=CARTESIAN_POINT ( 'NONE',  ( 124.6879301918981042, 6.110000000000002984, -1.637169565754156730 ) ) ;
#44462=CARTESIAN_POINT ( 'NONE',  ( 51.70419371712956291, -6.884901960086285300, -3.975000000000000089 ) ) ;
#44467=CARTESIAN_POINT ( 'NONE',  ( 47.22916666666665719, 7.950000000000001954, -2.130196079827421762 ) ) ;
#44477=CARTESIAN_POINT ( 'NONE',  ( 38.64626352523144703, -4.472830434245840259, 4.472830434245839371 ) ) ;
#44486=( GEOMETRIC_REPRESENTATION_CONTEXT ( 3 ) GLOBAL_UNCERTAINTY_ASSIGNED_CONTEXT ( ( #124435 ) ) GLOBAL_UNIT_ASSIGNED_CONTEXT ( ( #114529, #132222, #47894 ) ) REPRESENTATION_CONTEXT ( 'NONE', 'WORKASPACE' ) );
#44488=CARTESIAN_POINT ( 'NONE',  ( 81.45419371712955581, 6.884901960086283523, 3.975000000000002753 ) ) ;
#44497=CARTESIAN_POINT ( 'NONE',  ( 86.77126352523143282, 4.472830434245838482, 4.472830434245842035 ) ) ;
#44506=CARTESIAN_POINT ( 'NONE',  ( 61.45376352523145158, -6.109999999999998543, -3.741295971395162543E-16 ) ) ;
#44539=CARTESIAN_POINT ( 'NONE',  ( 78.95376352523145158, -6.109999999999998543, -3.741295971395162543E-16 ) ) ;
#44566=CARTESIAN_POINT ( 'NONE',  ( 25.22959685856476497, -6.110000000000000320, -1.637169565754161393 ) ) ;
#44577=EDGE_LOOP ( 'NONE', ( #81197, #117918, #110046, #119005 ) ) ;
#44610=DIRECTION ( 'NONE',  ( -1.000000000000000000, -0.000000000000000000, -0.000000000000000000 ) ) ;
#44623=CARTESIAN_POINT ( 'NONE',  ( 54.89126352523145158, -4.472830434245839371, -4.472830434245839371 ) ) ;
#44650=CARTESIAN_POINT ( 'NONE',  ( 81.30836038379624142, 7.949999999999997513, 2.130196079827431088 ) ) ;
#44654=CARTESIAN_POINT ( 'NONE',  ( 74.35416666666664298, -2.130196079827425315, -7.950000000000001066 ) ) ;
#44664=CARTESIAN_POINT ( 'NONE',  ( 61.97959685856476852, 6.109999999999999432, 1.637169565754164280 ) ) ;
#44685=CARTESIAN_POINT ( 'NONE',  ( 65.62543019189810423, 5.291415217122919401, 3.055000000000002824 ) ) ;
#44687=EDGE_CURVE ( 'NONE', #133905, #24699, #89161, .T. ) ;
#44721=CARTESIAN_POINT ( 'NONE',  ( 102.8704301918981230, -3.055000000000001492, 5.291415217122917625 ) ) ;
#44745=CARTESIAN_POINT ( 'NONE',  ( 56.14626352523143993, -4.472830434245840259, 4.472830434245838482 ) ) ;
#44751=CARTESIAN_POINT ( 'NONE',  ( 87.64626352523143282, -4.472830434245840259, 4.472830434245838482 ) ) ;
#44769=CARTESIAN_POINT ( 'NONE',  ( 119.7870968585647802, 3.054999999999997495, 5.291415217122919401 ) ) ;
#44821=CARTESIAN_POINT ( 'NONE',  ( 113.9750270504628986, -5.819803920172572198, 5.819803920172572198 ) ) ;
#44837=CARTESIAN_POINT ( 'NONE',  ( 104.2712635252314470, 4.472830434245839371, 4.472830434245842035 ) ) ;
#44857=ORIENTED_EDGE ( 'NONE', *, *, #52381, .T. ) ;
#44861=CARTESIAN_POINT ( 'NONE',  ( 92.60459685856478984, 1.637169565754164946, -6.109999999999999432 ) ) ;
#44874=FACE_OUTER_BOUND ( 'NONE', #84428, .T. ) ;
#44876=CARTESIAN_POINT ( 'NONE',  ( 82.59959685856478018, -6.109999999999997655, -1.637169565754160283 ) ) ;
#44908=CARTESIAN_POINT ( 'NONE',  ( 27.00000000000000355, 0.000000000000000000, 0.000000000000000000 ) ) ;
#44944=ORIENTED_EDGE ( 'NONE', *, *, #44316, .F. ) ;
#44951=ORIENTED_EDGE ( 'NONE', *, *, #141743, .F. ) ;
#44959=CARTESIAN_POINT ( 'NONE',  ( 85.66209685856478018, -5.291415217122919401, 3.054999999999998384 ) ) ;
#44960=CARTESIAN_POINT ( 'NONE',  ( 6.538661199317437500, -9.242530024995444293, 2.210267608354182123 ) ) ;
#45001=CARTESIAN_POINT ( 'NONE',  ( 109.9375000000000000, 5.819803920172574863, -5.819803920172573086 ) ) ;
#45006=CARTESIAN_POINT ( 'NONE',  ( 99.00000000000000000, 0.000000000000000000, -7.950000000000000178 ) ) ;
#45030=CARTESIAN_POINT ( 'NONE',  ( 119.4379301918981042, -6.110000000000001208, 1.637169565754158951 ) ) ;
#45039=CARTESIAN_POINT ( 'NONE',  ( 113.8079301918981230, -6.109999999999998543, 1.637169565754158063 ) ) ;
#45047=CARTESIAN_POINT ( 'NONE',  ( 38.93793019189809002, -6.110000000000001208, 1.637169565754158951 ) ) ;
#45052=ADVANCED_FACE ( 'NONE', ( #104789 ), #82348, .F. ) ;
#45059=CARTESIAN_POINT ( 'NONE',  ( 29.07876352523144803, -7.482591942790325086E-16, 6.109999999999998543 ) ) ;
#45074=FACE_OUTER_BOUND ( 'NONE', #89963, .T. ) ;
#45085=ADVANCED_FACE ( 'NONE', ( #72215 ), #29359, .T. ) ;
#45086=CARTESIAN_POINT ( 'NONE',  ( 43.22459685856478728, -1.637169565754160949, 6.109999999999997655 ) ) ;
#45117=CARTESIAN_POINT ( 'NONE',  ( 112.3495968585647802, 6.109999999999997655, 1.637169565754163836 ) ) ;
#45129=CARTESIAN_POINT ( 'NONE',  ( 120.2916666666666714, 3.975000000000003642, -6.884901960086285300 ) ) ;
#45154=CARTESIAN_POINT ( 'NONE',  ( 20.65000000000000213, 0.000000000000000000, 9.500000000000000000 ) ) ;
#45158=CARTESIAN_POINT ( 'NONE',  ( 31.99543019189811233, 5.291415217122917625, 3.055000000000002380 ) ) ;
#45163=CARTESIAN_POINT ( 'NONE',  ( 124.9583333333333428, 3.974999999999997424, 6.884901960086288852 ) ) ;
#45174=CARTESIAN_POINT ( 'NONE',  ( 121.7712635252314328, 4.472830434245839371, 4.472830434245842035 ) ) ;
#45179=CARTESIAN_POINT ( 'NONE',  ( 78.58333333333334281, 6.884901960086290629, -3.974999999999994316 ) ) ;
#45184=CARTESIAN_POINT ( 'NONE',  ( 45.72502705046288440, 5.819803920172573086, -5.819803920172572198 ) ) ;
#45189=CARTESIAN_POINT ( 'NONE',  ( 44.31249999999999289, 5.819803920172571310, 5.819803920172575751 ) ) ;
#45193=ORIENTED_EDGE ( 'NONE', *, *, #13700, .T. ) ;
#45198=CARTESIAN_POINT ( 'NONE',  ( 38.79209685856477563, -5.291415217122921177, 3.054999999999999272 ) ) ;
#45203=DIRECTION ( 'NONE',  ( -1.000000000000000000, -0.000000000000000000, -0.000000000000000000 ) ) ;
#45223=CARTESIAN_POINT ( 'NONE',  ( 56.20376352523144448, 6.109999999999998543, 1.122388791418548911E-15 ) ) ;
#45253=CARTESIAN_POINT ( 'NONE',  ( 74.72459685856478018, -1.637169565754160949, 6.109999999999997655 ) ) ;
#45276=CARTESIAN_POINT ( 'NONE',  ( 25.37543019189810067, -5.291415217122920289, -3.055000000000001492 ) ) ;
#45296=EDGE_LOOP ( 'NONE', ( #104481, #99434, #68240, #71179 ) ) ;
#45327=CARTESIAN_POINT ( 'NONE',  ( 54.30793019189810167, -6.109999999999999432, 1.637169565754158507 ) ) ;
#45352=CARTESIAN_POINT ( 'NONE',  ( 74.16252705046288440, 7.949999999999998401, 1.460391307983218338E-15 ) ) ;
#45357=CARTESIAN_POINT ( 'NONE',  ( 73.18749999999995737, -5.819803920172573086, 5.819803920172572198 ) ) ;
#45367=CARTESIAN_POINT ( 'NONE',  ( 65.77126352523144703, 4.472830434245839371, 4.472830434245842035 ) ) ;
#45371=DIRECTION ( 'NONE',  ( -1.000000000000000000, -0.000000000000000000, -0.000000000000000000 ) ) ;
#45384=CARTESIAN_POINT ( 'NONE',  ( 63.72959685856477563, -6.110000000000000320, -1.637169565754161393 ) ) ;
#45415=CARTESIAN_POINT ( 'NONE',  ( 105.4954301918981230, 5.291415217122916737, 3.055000000000001936 ) ) ;
#45440=CARTESIAN_POINT ( 'NONE',  ( 54.83376352523143282, 6.110000000000001208, 1.122388791418549305E-15 ) ) ;
#45446=CARTESIAN_POINT ( 'NONE',  ( 91.00043019189810423, -3.055000000000002380, 5.291415217122920289 ) ) ;
#45450=ORIENTED_EDGE ( 'NONE', *, *, #125407, .F. ) ;
#45485=CARTESIAN_POINT ( 'NONE',  ( 58.31249999999998579, 5.819803920172571310, 5.819803920172576639 ) ) ;
#45490=CARTESIAN_POINT ( 'NONE',  ( 8.124863741626466407, 8.711972394638584305, -3.792219164446597013 ) ) ;
#45515=CARTESIAN_POINT ( 'NONE',  ( 104.0583603837962272, -7.949999999999997513, -2.130196079827425759 ) ) ;
#45533=CARTESIAN_POINT ( 'NONE',  ( 90.70876352523143282, -7.482591942790329030E-16, 6.110000000000001208 ) ) ;
#45560=CARTESIAN_POINT ( 'NONE',  ( 96.39626352523144703, 4.472830434245840259, -4.472830434245839371 ) ) ;
#45572=CARTESIAN_POINT ( 'NONE',  ( 90.62043019189810877, 3.055000000000001936, -5.291415217122916737 ) ) ;
#45587=ORIENTED_EDGE ( 'NONE', *, *, #39228, .T. ) ;
#45597=CARTESIAN_POINT ( 'NONE',  ( 55.93336038379622011, 2.130196079827431532, -7.949999999999996625 ) ) ;
#45613=ORIENTED_EDGE ( 'NONE', *, *, #54848, .T. ) ;
#45620=CARTESIAN_POINT ( 'NONE',  ( 116.6670968585647756, -3.055000000000000160, -5.291415217122921177 ) ) ;
#45648=CARTESIAN_POINT ( 'NONE',  ( 82.74543019189812298, -5.291415217122919401, -3.055000000000000604 ) ) ;
#45696=CARTESIAN_POINT ( 'NONE',  ( 109.6458333333333286, 2.130196079827431976, -7.949999999999998401 ) ) ;
#45700=CARTESIAN_POINT ( 'NONE',  ( 106.0000000000000000, 0.000000000000000000, -7.950000000000000178 ) ) ;
#45727=CARTESIAN_POINT ( 'NONE',  ( 118.7087635252314328, -7.482591942790329030E-16, 6.110000000000001208 ) ) ;
#45732=CARTESIAN_POINT ( 'NONE',  ( 100.6041666666666572, 2.130196079827384459, 7.950000000000025047 ) ) ;
#45736=CARTESIAN_POINT ( 'NONE',  ( 114.6829301918980946, -1.637169565754158951, -6.109999999999998543 ) ) ;
#45744=CARTESIAN_POINT ( 'NONE',  ( 35.29209685856476852, -5.291415217122921177, 3.054999999999999272 ) ) ;
#45754=CARTESIAN_POINT ( 'NONE',  ( 28.05793019189811233, 6.110000000000000320, -1.637169565754156064 ) ) ;
#45784=CARTESIAN_POINT ( 'NONE',  ( 48.32876352523145158, 0.000000000000000000, -6.109999999999998543 ) ) ;
#45791=( BOUNDED_CURVE ( )  B_SPLINE_CURVE ( 2, ( #124227, #1688, #13298, #48826, #103181, #79348, #123547, #27049, #113331, #37218, #24211, #114749, #124934 ),
 .UNSPECIFIED., .F., .F. ) 
 B_SPLINE_CURVE_WITH_KNOTS ( ( 3, 2, 2, 2, 2, 2, 3 ),
 ( 0.8166666666666666519, 0.8194444444444444198, 0.8222222222222221877, 0.8249999999999999556, 0.8277777777777777235, 0.8305555555555556024, 0.8333333333333333703 ),
 .UNSPECIFIED. ) 
 CURVE ( )  GEOMETRIC_REPRESENTATION_ITEM ( )  RATIONAL_B_SPLINE_CURVE ( ( 1.000000000000000000, 0.9659258262890683122, 1.000000000000000000, 0.9659258262890683122, 1.000000000000000000, 0.9659258262890683122, 1.000000000000000000, 0.9659258262890683122, 1.000000000000000000, 0.9659258262890683122, 1.000000000000000000, 0.9659258262890683122, 1.000000000000000000 ) ) 
 REPRESENTATION_ITEM ( '' )  );
#45811=CARTESIAN_POINT ( 'NONE',  ( 113.0787635252314516, -7.482591942790327058E-16, 6.109999999999999432 ) ) ;
#45825=CARTESIAN_POINT ( 'NONE',  ( 1.500000000000000000, 0.000000000000000000, 0.000000000000000000 ) ) ;
#45873=CARTESIAN_POINT ( 'NONE',  ( 117.5420968585647756, 5.291415217122923842, -3.054999999999996163 ) ) ;
#45884=CARTESIAN_POINT ( 'NONE',  ( 45.14169371712955581, -2.130196079827424871, -7.949999999999999289 ) ) ;
#45890=CARTESIAN_POINT ( 'NONE',  ( 46.35416666666666430, -2.130196079827425315, -7.950000000000001066 ) ) ;
#45896=CARTESIAN_POINT ( 'NONE',  ( 41.56293019189811133, 1.637169565754157174, 6.110000000000002984 ) ) ;
#45908=CARTESIAN_POINT ( 'NONE',  ( 40.03752705046288440, -9.735942053221456900E-16, 7.949999999999998401 ) ) ;
#45917=CARTESIAN_POINT ( 'NONE',  ( 59.55793019189812298, 6.110000000000000320, -1.637169565754156064 ) ) ;
#45948=CARTESIAN_POINT ( 'NONE',  ( 75.59959685856478018, -6.109999999999997655, -1.637169565754160283 ) ) ;
#45977=CARTESIAN_POINT ( 'NONE',  ( 25.52126352523142927, -4.472830434245838482, -4.472830434245840259 ) ) ;
#46022=ORIENTED_EDGE ( 'NONE', *, *, #61238, .T. ) ;
#46028=CARTESIAN_POINT ( 'NONE',  ( 56.49543019189812298, 5.291415217122917625, 3.055000000000002380 ) ) ;
#46057=CARTESIAN_POINT ( 'NONE',  ( 78.68336038379622721, -2.130196079827426203, 7.949999999999997513 ) ) ;
#46062=CARTESIAN_POINT ( 'NONE',  ( 75.37500000000000000, 7.950000000000000178, 1.460391307983218535E-15 ) ) ;
#46072=CARTESIAN_POINT ( 'NONE',  ( 70.43793019189810423, -6.110000000000001208, 1.637169565754158951 ) ) ;
#46092=CARTESIAN_POINT ( 'NONE',  ( 54.39626352523144703, 4.472830434245840259, -4.472830434245839371 ) ) ;
#46097=CARTESIAN_POINT ( 'NONE',  ( 54.66666666666667140, 6.884901960086285300, 3.975000000000003642 ) ) ;
#46121=CARTESIAN_POINT ( 'NONE',  ( 102.5787635252314658, -7.482591942790325086E-16, 6.109999999999998543 ) ) ;
#46147=VECTOR ( 'NONE', #57191, 1000.000000000000000 ) ;
#46151=CARTESIAN_POINT ( 'NONE',  ( 51.04209685856476852, 5.291415217122923842, -3.054999999999996163 ) ) ;
#46153=EDGE_CURVE ( 'NONE', #10128, #143125, #102691, .T. ) ;
#46158=CARTESIAN_POINT ( 'NONE',  ( 89.25043019189810423, 3.055000000000002824, -5.291415217122919401 ) ) ;
#46218=VERTEX_POINT ( 'NONE', #83074 ) ;
#46228=CARTESIAN_POINT ( 'NONE',  ( 98.66252705046289861, 7.949999999999998401, 1.460391307983218338E-15 ) ) ;
#46243=CARTESIAN_POINT ( 'NONE',  ( 97.12543019189810423, 5.291415217122919401, 3.055000000000002824 ) ) ;
#46272=CARTESIAN_POINT ( 'NONE',  ( 85.89626352523144703, 4.472830434245840259, -4.472830434245839371 ) ) ;
#46286=CARTESIAN_POINT ( 'NONE',  ( 84.93293019189812298, 1.637169565754156508, 6.110000000000000320 ) ) ;
#46297=ADVANCED_FACE ( 'NONE', ( #50449 ), #106211, .T. ) ;
#46327=ORIENTED_EDGE ( 'NONE', *, *, #23886, .F. ) ;
#46328=DIRECTION ( 'NONE',  ( -1.000000000000000000, -0.000000000000000000, -0.000000000000000000 ) ) ;
#46340=CARTESIAN_POINT ( 'NONE',  ( 121.9170968585647756, 3.054999999999998828, 5.291415217122922066 ) ) ;
#46376=CARTESIAN_POINT ( 'NONE',  ( 81.28709685856478018, 3.054999999999997939, 5.291415217122920289 ) ) ;
#46381=ORIENTED_EDGE ( 'NONE', *, *, #106117, .F. ) ;
#46427=CARTESIAN_POINT ( 'NONE',  ( 96.37500000000000000, 7.950000000000000178, 1.460391307983218535E-15 ) ) ;
#46435=CARTESIAN_POINT ( 'NONE',  ( 13.61855308952199195, 9.051029200191091917, 2.893811631854878996 ) ) ;
#46450=CARTESIAN_POINT ( 'NONE',  ( 26.45376352523144803, -6.109999999999998543, -3.741295971395162543E-16 ) ) ;
#46454=CARTESIAN_POINT ( 'NONE',  ( 109.0837635252314470, -6.110000000000001208, -3.741295971395164515E-16 ) ) ;
#46462=CARTESIAN_POINT ( 'NONE',  ( 110.0162635252314374, -4.472830434245839371, 4.472830434245839371 ) ) ;
#46474=VERTEX_POINT ( 'NONE', #110500 ) ;
#46482=CARTESIAN_POINT ( 'NONE',  ( 32.87043019189811588, -3.055000000000001492, 5.291415217122917625 ) ) ;
#46491=VERTEX_POINT ( 'NONE', #80775 ) ;
#46520=CARTESIAN_POINT ( 'NONE',  ( 51.24543019189811588, -5.291415217122918513, -3.055000000000000160 ) ) ;
#46553=CARTESIAN_POINT ( 'NONE',  ( 112.9329301918981230, 1.637169565754156730, 6.110000000000001208 ) ) ;
#46567=CARTESIAN_POINT ( 'NONE',  ( 121.1666666666666714, 6.884901960086285300, 3.975000000000003642 ) ) ;
#46585=EDGE_CURVE ( 'NONE', #77789, #128763, #14784, .T. ) ;
#46605=CARTESIAN_POINT ( 'NONE',  ( 123.9375000000000142, 5.819803920172573974, -5.819803920172572198 ) ) ;
#46620=CARTESIAN_POINT ( 'NONE',  ( 125.2712635252314470, 4.472830434245839371, 4.472830434245842035 ) ) ;
#46625=CARTESIAN_POINT ( 'NONE',  ( 104.9333603837962272, 2.130196079827431532, -7.949999999999996625 ) ) ;
#46632=CARTESIAN_POINT ( 'NONE',  ( 48.49586038379622011, -3.974999999999998312, -6.884901960086286188 ) ) ;
#46638=CARTESIAN_POINT ( 'NONE',  ( 44.60416666666665719, 2.130196079827422206, 7.950000000000001954 ) ) ;
#46645=CARTESIAN_POINT ( 'NONE',  ( 40.68793019189811133, 6.110000000000002984, -1.637169565754156730 ) ) ;
#46652=FACE_OUTER_BOUND ( 'NONE', #114053, .T. ) ;
#46664=CARTESIAN_POINT ( 'NONE',  ( 56.05793019189811588, 6.110000000000000320, -1.637169565754156064 ) ) ;
#46691=CARTESIAN_POINT ( 'NONE',  ( 20.65000000000000213, 0.000000000000000000, 0.000000000000000000 ) ) ;
#46692=VECTOR ( 'NONE', #19826, 1000.000000000000000 ) ;
#46701=CARTESIAN_POINT ( 'NONE',  ( 73.55793019189812298, 6.110000000000000320, -1.637169565754156064 ) ) ;
#46713=CARTESIAN_POINT ( 'NONE',  ( 0.000000000000000000, 0.000000000000000000, 0.000000000000000000 ) ) ;
#46727=CARTESIAN_POINT ( 'NONE',  ( 28.72959685856476852, -6.110000000000000320, -1.637169565754161393 ) ) ;
#46735=CARTESIAN_POINT ( 'NONE',  ( 119.2250270504628986, 5.819803920172573974, -5.819803920172573086 ) ) ;
#46765=CARTESIAN_POINT ( 'NONE',  ( 66.28752705046289861, 0.000000000000000000, -7.949999999999998401 ) ) ;
#46774=CARTESIAN_POINT ( 'NONE',  ( 53.28709685856478018, 3.054999999999997939, 5.291415217122920289 ) ) ;
#46801=CARTESIAN_POINT ( 'NONE',  ( 70.66252705046288440, 7.949999999999998401, 1.460391307983218338E-15 ) ) ;
#46805=CARTESIAN_POINT ( 'NONE',  ( 77.12500000000000000, -7.950000000000000178, -4.867971026610729436E-16 ) ) ;
#46813=VECTOR ( 'NONE', #1119, 1000.000000000000000 ) ;
#46815=CARTESIAN_POINT ( 'NONE',  ( 68.10459685856474721, 1.637169565754164946, -6.109999999999999432 ) ) ;
#46832=CARTESIAN_POINT ( 'NONE',  ( 52.35459685856476852, -1.637169565754161615, 6.110000000000000320 ) ) ;
#46841=CARTESIAN_POINT ( 'NONE',  ( 55.10416666666665719, 2.130196079827498146, 7.949999999999958433 ) ) ;
#46851=CARTESIAN_POINT ( 'NONE',  ( 112.8083603837962272, 7.949999999999996625, 2.130196079827431088 ) ) ;
#46868=CARTESIAN_POINT ( 'NONE',  ( 99.51626352523145158, -4.472830434245838482, 4.472830434245838482 ) ) ;
#46887=CARTESIAN_POINT ( 'NONE',  ( 27.49586038379622721, -3.974999999999998312, -6.884901960086286188 ) ) ;
#46894=CARTESIAN_POINT ( 'NONE',  ( 87.77083333333331439, -7.949999999999998401, -2.130196079827426203 ) ) ;
#46899=EDGE_CURVE ( 'NONE', #54290, #49146, #73764, .T. ) ;
#46900=CARTESIAN_POINT ( 'NONE',  ( 55.56293019189809712, 1.637169565754157174, 6.110000000000002984 ) ) ;
#46905=CARTESIAN_POINT ( 'NONE',  ( 94.93793019189810423, -6.110000000000001208, 1.637169565754158951 ) ) ;
#46916=CARTESIAN_POINT ( 'NONE',  ( 125.7662635252314658, 4.472830434245839371, -4.472830434245839371 ) ) ;
#46941=CARTESIAN_POINT ( 'NONE',  ( 9.176104866590083731, 8.505782047251113198, -4.231528338128802247 ) ) ;
#46966=CARTESIAN_POINT ( 'NONE',  ( 100.8500270504628986, -5.819803920172572198, -5.819803920172572198 ) ) ;
#46986=CARTESIAN_POINT ( 'NONE',  ( 90.41709685856477563, 3.054999999999998828, 5.291415217122922066 ) ) ;
#47004=CARTESIAN_POINT ( 'NONE',  ( 102.4541937171295700, 6.884901960086283523, 3.975000000000002753 ) ) ;
#47011=CARTESIAN_POINT ( 'NONE',  ( 78.89626352523143282, 4.472830434245840259, -4.472830434245839371 ) ) ;
#47025=CARTESIAN_POINT ( 'NONE',  ( 78.37043019189812298, -3.055000000000001492, 5.291415217122917625 ) ) ;
#47040=DIRECTION ( 'NONE',  ( -0.000000000000000000, 0.000000000000000000, 1.000000000000000000 ) ) ;
#47076=CARTESIAN_POINT ( 'NONE',  ( 95.20833333333334281, -3.974999999999999201, -6.884901960086287964 ) ) ;
#47080=CARTESIAN_POINT ( 'NONE',  ( 118.4170968585647756, 3.054999999999998828, 5.291415217122922066 ) ) ;
#47135=CARTESIAN_POINT ( 'NONE',  ( 104.2500000000000000, -9.735942053221458872E-16, 7.950000000000000178 ) ) ;
#47159=CARTESIAN_POINT ( 'NONE',  ( 95.35416666666665719, -2.130196079827425315, -7.950000000000001066 ) ) ;
#47167=CARTESIAN_POINT ( 'NONE',  ( 10.32500000000000107, 8.432637487761466488, -4.375000000000001776 ) ) ;
#47180=CARTESIAN_POINT ( 'NONE',  ( 86.70419371712955581, -6.884901960086285300, -3.975000000000000089 ) ) ;
#47184=CARTESIAN_POINT ( 'NONE',  ( 111.4170968585647614, 3.054999999999998828, 5.291415217122922066 ) ) ;
#47194=CARTESIAN_POINT ( 'NONE',  ( 103.1620968585647802, -5.291415217122919401, 3.054999999999997939 ) ) ;
#47199=PRODUCT_DEFINITION_FORMATION_WITH_SPECIFIED_SOURCE ( 'ANY', '', #96739, .NOT_KNOWN. ) ;
#47209=CARTESIAN_POINT ( 'NONE',  ( 34.32876352523143737, 0.000000000000000000, -6.109999999999998543 ) ) ;
#47241=CARTESIAN_POINT ( 'NONE',  ( 38.99543019189812298, 5.291415217122916737, 3.055000000000001936 ) ) ;
#47275=CARTESIAN_POINT ( 'NONE',  ( 115.1204301918981230, 3.055000000000002380, -5.291415217122917625 ) ) ;
#47323=CARTESIAN_POINT ( 'NONE',  ( 119.8541666666666430, -2.130196079827425315, -7.950000000000001066 ) ) ;
#47338=CARTESIAN_POINT ( 'NONE',  ( 99.53752705046289861, -9.735942053221456900E-16, 7.949999999999998401 ) ) ;
#47339=CARTESIAN_POINT ( 'NONE',  ( 109.8129301918981042, -1.637169565754159617, -6.110000000000001208 ) ) ;
#47348=CARTESIAN_POINT ( 'NONE',  ( 50.97502705046287730, -5.819803920172572198, 5.819803920172572198 ) ) ;
#47355=CARTESIAN_POINT ( 'NONE',  ( 36.14583333333332149, 2.130196079827431976, -7.949999999999999289 ) ) ;
#47363=CARTESIAN_POINT ( 'NONE',  ( 42.58376352523143993, -6.110000000000001208, -3.741295971395164515E-16 ) ) ;
#47379=LINE ( 'NONE', #79283, #6939 ) ;
#47381=CARTESIAN_POINT ( 'NONE',  ( 61.01626352523143737, -4.472830434245839371, 4.472830434245839371 ) ) ;
#47382=CARTESIAN_POINT ( 'NONE',  ( 125.1041666666666572, 2.130196079827431532, 7.949999999999996625 ) ) ;
#47395=B_SPLINE_CURVE_WITH_KNOTS ( 'NONE', 3,
 ( #127450, #72411, #116580, #17265, #125324, #73105, #61527, #17943, #26715, #83990, #95527, #139793, #114434, #6337, #15102, #70958, #128191, #48467, #92667, #136906, #28869, #117263, #37608, #126050, #115113, #15783, #60079, #104248, #130330, #9948, #54221, #20820, #62942, #96222, #52735, #98408 ),
 .UNSPECIFIED., .F., .F.,
 ( 4, 2, 2, 2, 2, 2, 2, 2, 2, 2, 2, 2, 2, 2, 2, 2, 2, 4 ),
 ( 0.006941909043857026965, 0.007808636908474057142, 0.008675364773091087320, 0.009542092637708117497, 0.01040882050232514767, 0.01127554836694217785, 0.01214227623155920976, 0.01300900409617623821, 0.01387573196079327012, 0.01474245982541030030, 0.01560918769002733048, 0.01647591555464435892, 0.01734264341926139083, 0.01820937128387842274, 0.01907609914849545119, 0.01994282701311247963, 0.02037619094542100079, 0.02080955487772951848 ),
 .UNSPECIFIED. ) ;
#47409=CARTESIAN_POINT ( 'NONE',  ( 67.57876352523145158, -7.482591942790325086E-16, 6.109999999999998543 ) ) ;
#47456=CARTESIAN_POINT ( 'NONE',  ( 27.83333333333332149, -6.884901960086287964, 3.974999999999998312 ) ) ;
#47467=DIRECTION ( 'NONE',  ( -1.000000000000000000, -0.000000000000000000, -0.000000000000000000 ) ) ;
#47475=EDGE_CURVE ( 'NONE', #91561, #102725, #18846, .T. ) ;
#47484=CARTESIAN_POINT ( 'NONE',  ( 51.82876352523144448, 0.000000000000000000, -6.109999999999999432 ) ) ;
#47507=CARTESIAN_POINT ( 'NONE',  ( 77.22502705046287019, 5.819803920172573086, -5.819803920172572198 ) ) ;
#47512=CARTESIAN_POINT ( 'NONE',  ( 59.62500000000000000, -7.950000000000000178, -4.867971026610729436E-16 ) ) ;
#47522=CARTESIAN_POINT ( 'NONE',  ( 64.31293019189810423, -1.637169565754159617, -6.110000000000001208 ) ) ;
#47550=CARTESIAN_POINT ( 'NONE',  ( 73.28752705046288440, 0.000000000000000000, -7.949999999999998401 ) ) ;
#47566=CARTESIAN_POINT ( 'NONE',  ( 38.28752705046288440, 0.000000000000000000, -7.949999999999998401 ) ) ;
#47571=CARTESIAN_POINT ( 'NONE',  ( 102.7245968585647802, -1.637169565754160949, 6.109999999999997655 ) ) ;
#47594=CARTESIAN_POINT ( 'NONE',  ( 57.16709685856477563, -3.055000000000000160, -5.291415217122921177 ) ) ;
#47612=DIRECTION ( 'NONE',  ( -1.000000000000000000, -0.000000000000000000, -0.000000000000000000 ) ) ;
#47668=CARTESIAN_POINT ( 'NONE',  ( 104.6416937171295558, -2.130196079827424871, -7.949999999999999289 ) ) ;
#47683=CARTESIAN_POINT ( 'NONE',  ( 94.06293019189809002, 1.637169565754157174, 6.110000000000002984 ) ) ;
#47708=CARTESIAN_POINT ( 'NONE',  ( 83.41709685856477563, 3.054999999999998828, 5.291415217122922066 ) ) ;
#47716=CARTESIAN_POINT ( 'NONE',  ( 104.2500000000000000, -9.735942053221458872E-16, 7.950000000000000178 ) ) ;
#47719=CARTESIAN_POINT ( 'NONE',  ( 74.72459685856476597, -1.637169565754160949, 6.109999999999997655 ) ) ;
#47746=LINE ( 'NONE', #70910, #46147 ) ;
#47764=CARTESIAN_POINT ( 'NONE',  ( 122.9379301918981042, -6.110000000000001208, 1.637169565754158951 ) ) ;
#47768=DIRECTION ( 'NONE',  ( 0.000000000000000000, -0.000000000000000000, 1.000000000000000000 ) ) ;
#47796=CARTESIAN_POINT ( 'NONE',  ( 98.95419371712955581, 6.884901960086283523, 3.975000000000002753 ) ) ;
#47802=CARTESIAN_POINT ( 'NONE',  ( 0.000000000000000000, 0.000000000000000000, 0.000000000000000000 ) ) ;
#47834=CARTESIAN_POINT ( 'NONE',  ( 31.55793019189810522, 6.110000000000001208, -1.637169565754156286 ) ) ;
#47851=CARTESIAN_POINT ( 'NONE',  ( 89.66666666666667140, 6.884901960086285300, 3.975000000000003642 ) ) ;
#47856=CARTESIAN_POINT ( 'NONE',  ( 14.66377360979165267, 9.483362590305993933, -0.5803357009920233622 ) ) ;
#47858=DIRECTION ( 'NONE',  ( 0.000000000000000000, 0.000000000000000000, 1.000000000000000000 ) ) ;
#47861=CARTESIAN_POINT ( 'NONE',  ( 126.4318778290302276, 7.022613924927493478, 0.02362404962084689586 ) ) ;
#47873=CARTESIAN_POINT ( 'NONE',  ( 110.2504301918981042, 3.055000000000002824, -5.291415217122919401 ) ) ;
#47880=CARTESIAN_POINT ( 'NONE',  ( 0.000000000000000000, 0.000000000000000000, 0.000000000000000000 ) ) ;
#47881=CARTESIAN_POINT ( 'NONE',  ( 105.9329301918981088, 1.637169565754156508, 6.110000000000000320 ) ) ;
#47882=ORIENTED_EDGE ( 'NONE', *, *, #12340, .T. ) ;
#47894=( NAMED_UNIT ( * ) SI_UNIT ( $, .STERADIAN. ) SOLID_ANGLE_UNIT ( ) );
#47927=CARTESIAN_POINT ( 'NONE',  ( 42.34959685856478018, 6.109999999999996767, 1.637169565754163836 ) ) ;
#47931=CARTESIAN_POINT ( 'NONE',  ( 10.32500000000000107, -8.432637487761466488, -4.375000000000001776 ) ) ;
#47961=CARTESIAN_POINT ( 'NONE',  ( 99.22459685856479439, -1.637169565754161171, 6.109999999999998543 ) ) ;
#47974=ORIENTED_EDGE ( 'NONE', *, *, #31435, .T. ) ;
#47987=CARTESIAN_POINT ( 'NONE',  ( 112.1250000000000000, -7.950000000000000178, -4.867971026610729436E-16 ) ) ;
#48004=CARTESIAN_POINT ( 'NONE',  ( 120.8750000000000000, 7.950000000000000178, 1.460391307983218535E-15 ) ) ;
#48015=CARTESIAN_POINT ( 'NONE',  ( 114.1879301918980900, 6.110000000000002984, -1.637169565754156730 ) ) ;
#48024=CARTESIAN_POINT ( 'NONE',  ( 41.93336038379621300, 2.130196079827431532, -7.949999999999997513 ) ) ;
#48030=CARTESIAN_POINT ( 'NONE',  ( 33.52083333333333570, 7.949999999999999289, 2.130196079827431532 ) ) ;
#48039=CARTESIAN_POINT ( 'NONE',  ( 29.02126352523143282, -4.472830434245839371, -4.472830434245840259 ) ) ;
#48053=CARTESIAN_POINT ( 'NONE',  ( 45.41209685856478728, 5.291415217122921177, -3.054999999999994831 ) ) ;
#48080=CARTESIAN_POINT ( 'NONE',  ( 69.32876352523145158, 0.000000000000000000, -6.109999999999998543 ) ) ;
#48116=CARTESIAN_POINT ( 'NONE',  ( 119.0791937171295700, 3.975000000000002753, -6.884901960086283523 ) ) ;
#48129=CARTESIAN_POINT ( 'NONE',  ( 125.2500000000000000, -9.735942053221458872E-16, 7.950000000000000178 ) ) ;
#48144=CARTESIAN_POINT ( 'NONE',  ( 66.14169371712955581, -2.130196079827424871, -7.949999999999998401 ) ) ;
#48153=CARTESIAN_POINT ( 'NONE',  ( 47.01626352523143026, -4.472830434245839371, 4.472830434245839371 ) ) ;
#48161=DIRECTION ( 'NONE',  ( 0.000000000000000000, 0.000000000000000000, 1.000000000000000000 ) ) ;
#48168=CARTESIAN_POINT ( 'NONE',  ( 115.2875270504628986, 0.000000000000000000, -7.949999999999998401 ) ) ;
#48172=CARTESIAN_POINT ( 'NONE',  ( 77.80836038379621300, 7.949999999999997513, 2.130196079827431088 ) ) ;
#48177=CARTESIAN_POINT ( 'NONE',  ( 65.45833333333332860, 3.974999999999997424, 6.884901960086288852 ) ) ;
#48186=CARTESIAN_POINT ( 'NONE',  ( 52.79209685856476852, -5.291415217122921177, 3.054999999999999272 ) ) ;
#48213=CARTESIAN_POINT ( 'NONE',  ( 90.25000000000000000, -9.735942053221458872E-16, 7.950000000000000178 ) ) ;
#48232=CARTESIAN_POINT ( 'NONE',  ( 96.01626352523145158, -4.472830434245838482, 4.472830434245838482 ) ) ;
#48258=CARTESIAN_POINT ( 'NONE',  ( 45.50043019189810423, -3.055000000000002380, 5.291415217122920289 ) ) ;
#48272=CARTESIAN_POINT ( 'NONE',  ( 126.7870968585647944, 3.054999999999997939, 5.291415217122920289 ) ) ;
#48338=CARTESIAN_POINT ( 'NONE',  ( 100.4125270504628986, -7.949999999999998401, -4.867971026610728450E-16 ) ) ;
#48353=CARTESIAN_POINT ( 'NONE',  ( 93.91709685856477563, 3.054999999999998828, 5.291415217122922066 ) ) ;
#48372=CARTESIAN_POINT ( 'NONE',  ( 81.22959685856476142, -6.110000000000000320, -1.637169565754161393 ) ) ;
#48382=CARTESIAN_POINT ( 'NONE',  ( 76.91209685856479439, 5.291415217122921177, -3.054999999999994831 ) ) ;
#48408=EDGE_CURVE ( 'NONE', #24590, #31006, #94636, .T. ) ;
#48431=CARTESIAN_POINT ( 'NONE',  ( 71.02126352523144703, -4.472830434245838482, -4.472830434245840259 ) ) ;
#48435=EDGE_CURVE ( 'NONE', #82006, #96223, #76361, .T. ) ;
#48438=CARTESIAN_POINT ( 'NONE',  ( 108.7920968585647756, -5.291415217122921177, 3.054999999999999272 ) ) ;
#48441=PLANE ( 'NONE',  #54875 ) ;
#48467=CARTESIAN_POINT ( 'NONE',  ( 14.70008083135199684, -9.500037224963584492, -0.2878867768745749234 ) ) ;
#48487=DIRECTION ( 'NONE',  ( -1.000000000000000000, -0.000000000000000000, -0.000000000000000000 ) ) ;
#48504=CARTESIAN_POINT ( 'NONE',  ( 128.2666937171295274, -7.949999999999999289, 2.130196079827424427 ) ) ;
#48507=CARTESIAN_POINT ( 'NONE',  ( 47.91252705046289151, -7.949999999999998401, -4.867971026610728450E-16 ) ) ;
#48520=CARTESIAN_POINT ( 'NONE',  ( 91.27083333333334281, -7.949999999999999289, -2.130196079827426203 ) ) ;
#48527=CARTESIAN_POINT ( 'NONE',  ( 14.11343486808858216, 9.243406610528717593, -2.206469626207758772 ) ) ;
#48535=CARTESIAN_POINT ( 'NONE',  ( 126.4955769715163996, 6.892355196946173379, 1.023687185015854428 ) ) ;
#48550=CARTESIAN_POINT ( 'NONE',  ( 112.4379301918981184, -6.110000000000001208, 1.637169565754158951 ) ) ;
#48561=CARTESIAN_POINT ( 'NONE',  ( 106.6620968585647802, -5.291415217122919401, 3.054999999999997939 ) ) ;
#48573=( NAMED_UNIT ( * ) SI_UNIT ( $, .STERADIAN. ) SOLID_ANGLE_UNIT ( ) );
#48607=VECTOR ( 'NONE', #96106, 1000.000000000000000 ) ;
#48609=CARTESIAN_POINT ( 'NONE',  ( 35.05793019189810877, 6.110000000000000320, -1.637169565754156064 ) ) ;
#48650=CARTESIAN_POINT ( 'NONE',  ( 97.18293019189810877, -1.637169565754159173, -6.109999999999999432 ) ) ;
#48697=CARTESIAN_POINT ( 'NONE',  ( 123.3541666666666572, -2.130196079827425315, -7.950000000000001066 ) ) ;
#48711=CARTESIAN_POINT ( 'NONE',  ( 117.1045968585647898, 1.637169565754164946, -6.109999999999999432 ) ) ;
#48724=CARTESIAN_POINT ( 'NONE',  ( 34.35002705046288440, -5.819803920172572198, -5.819803920172572198 ) ) ;
#48729=CARTESIAN_POINT ( 'NONE',  ( 36.87499999999999289, 7.950000000000000178, 1.460391307983218535E-15 ) ) ;
#48743=CARTESIAN_POINT ( 'NONE',  ( 26.39626352523143282, 4.472830434245840259, -4.472830434245839371 ) ) ;
#48762=CARTESIAN_POINT ( 'NONE',  ( 44.39126352523143737, -4.472830434245839371, -4.472830434245839371 ) ) ;
#48765=EDGE_CURVE ( 'NONE', #46218, #33856, #123874, .T. ) ;
#48779=EDGE_CURVE ( 'NONE', #125681, #105597, #54878, .T. ) ;
#48793=CARTESIAN_POINT ( 'NONE',  ( 64.22459685856478018, -1.637169565754160949, 6.109999999999997655 ) ) ;
#48804=CARTESIAN_POINT ( 'NONE',  ( 34.83333333333332860, -6.884901960086287964, 3.974999999999998312 ) ) ;
#48821=CARTESIAN_POINT ( 'NONE',  ( 29.58333333333332149, 6.884901960086290629, -3.974999999999994316 ) ) ;
#48826=CARTESIAN_POINT ( 'NONE',  ( 43.10002705046289861, 5.819803920172570422, 5.819803920172575751 ) ) ;
#48872=CARTESIAN_POINT ( 'NONE',  ( 43.95376352523145158, -6.109999999999999432, -3.741295971395163529E-16 ) ) ;
#48889=DIRECTION ( 'NONE',  ( -1.000000000000000000, -0.000000000000000000, -0.000000000000000000 ) ) ;
#48897=CARTESIAN_POINT ( 'NONE',  ( 69.05836038379621300, -7.949999999999997513, -2.130196079827425759 ) ) ;
#48902=CARTESIAN_POINT ( 'NONE',  ( 68.37499999999998579, 7.950000000000000178, 1.460391307983218535E-15 ) ) ;
#48909=CARTESIAN_POINT ( 'NONE',  ( 33.22916666666665719, 7.950000000000001954, -2.130196079827421762 ) ) ;
#48914=CARTESIAN_POINT ( 'NONE',  ( 55.85459685856475431, -1.637169565754161615, 6.110000000000000320 ) ) ;
#48940=CARTESIAN_POINT ( 'NONE',  ( 72.70419371712955581, -6.884901960086285300, -3.975000000000000089 ) ) ;
#48967=CARTESIAN_POINT ( 'NONE',  ( 98.49543019189812298, 5.291415217122916737, 3.055000000000001936 ) ) ;
#48991=CARTESIAN_POINT ( 'NONE',  ( 42.14626352523143993, -4.472830434245840259, 4.472830434245838482 ) ) ;
#49011=VERTEX_POINT ( 'NONE', #41170 ) ;
#49039=CARTESIAN_POINT ( 'NONE',  ( 95.89169371712955581, 2.130196079827421762, 7.950000000000000178 ) ) ;
#49044=CARTESIAN_POINT ( 'NONE',  ( 72.24543019189810877, -5.291415217122919401, -3.055000000000000604 ) ) ;
#49048=CARTESIAN_POINT ( 'NONE',  ( 0.000000000000000000, 0.000000000000000000, 0.000000000000000000 ) ) ;
#49073=CARTESIAN_POINT ( 'NONE',  ( 91.51669371712957002, 7.950000000000001066, -2.130196079827421318 ) ) ;
#49091=CARTESIAN_POINT ( 'NONE',  ( 84.87543019189810423, -5.291415217122920289, -3.055000000000001492 ) ) ;
#49113=CARTESIAN_POINT ( 'NONE',  ( 80.50043019189810423, -3.055000000000002380, 5.291415217122920289 ) ) ;
#49146=VERTEX_POINT ( 'NONE', #133212 ) ;
#49158=CARTESIAN_POINT ( 'NONE',  ( 27.00000000000001421, -7.438727695536411666, -2.045697879312136980 ) ) ;
#49164=EDGE_CURVE ( 'NONE', #75310, #74997, #78105, .T. ) ;
#49170=CARTESIAN_POINT ( 'NONE',  ( 72.91709685856477563, 3.054999999999998828, 5.291415217122922066 ) ) ;
#49176=CARTESIAN_POINT ( 'NONE',  ( 108.0629301918980900, 1.637169565754157174, 6.110000000000002984 ) ) ;
#49192=ORIENTED_EDGE ( 'NONE', *, *, #26965, .F. ) ;
#49248=CARTESIAN_POINT ( 'NONE',  ( 32.72459685856478728, -1.637169565754161171, 6.109999999999998543 ) ) ;
#49267=CARTESIAN_POINT ( 'NONE',  ( 90.39583333333334281, -2.130196079827427091, 7.949999999999999289 ) ) ;
#49282=CARTESIAN_POINT ( 'NONE',  ( 126.5779968411016796, 6.505456897006314243, 2.228754984098625602 ) ) ;
#49294=CARTESIAN_POINT ( 'NONE',  ( 114.1879301918980900, 6.110000000000002984, -1.637169565754156730 ) ) ;
#49303=CARTESIAN_POINT ( 'NONE',  ( 107.2454301918981088, -5.291415217122918513, -3.055000000000000160 ) ) ;
#49356=CARTESIAN_POINT ( 'NONE',  ( 34.18293019189810167, -1.637169565754158951, -6.109999999999998543 ) ) ;
#49375=ORIENTED_EDGE ( 'NONE', *, *, #26786, .T. ) ;
#49394=CARTESIAN_POINT ( 'NONE',  ( 98.49543019189812298, 5.291415217122917625, 3.055000000000002380 ) ) ;
#49407=EDGE_CURVE ( 'NONE', #30975, #75310, #53476, .T. ) ;
#49436=CARTESIAN_POINT ( 'NONE',  ( 28.07919371712955225, 3.975000000000002753, -6.884901960086283523 ) ) ;
#49442=VERTEX_POINT ( 'NONE', #117821 ) ;
#49444=CARTESIAN_POINT ( 'NONE',  ( 119.1250000000000142, -7.950000000000000178, -4.867971026610729436E-16 ) ) ;
#49456=CARTESIAN_POINT ( 'NONE',  ( 114.9170968585647756, 3.054999999999998828, 5.291415217122922066 ) ) ;
#49462=CARTESIAN_POINT ( 'NONE',  ( 82.91252705046289861, -7.949999999999998401, -4.867971026610728450E-16 ) ) ;
#49467=CARTESIAN_POINT ( 'NONE',  ( 34.05836038379622721, -7.949999999999997513, -2.130196079827425759 ) ) ;
#49473=CARTESIAN_POINT ( 'NONE',  ( 38.62499999999999289, -7.950000000000000178, -4.867971026610729436E-16 ) ) ;
#49484=CARTESIAN_POINT ( 'NONE',  ( 128.8287635252314658, 0.000000000000000000, -6.109999999999998543 ) ) ;
#49494=CARTESIAN_POINT ( 'NONE',  ( 62.97916666666667140, -7.950000000000000178, 2.130196079827424427 ) ) ;
#49496=CARTESIAN_POINT ( 'NONE',  ( 51.04209685856476852, 5.291415217122923842, -3.054999999999996163 ) ) ;
#49507=CARTESIAN_POINT ( 'NONE',  ( 48.18293019189812298, -1.637169565754158951, -6.109999999999998543 ) ) ;
#49531=CARTESIAN_POINT ( 'NONE',  ( 61.74543019189811588, -5.291415217122918513, -3.055000000000000160 ) ) ;
#49576=VERTEX_POINT ( 'NONE', #69202 ) ;
#49607=CARTESIAN_POINT ( 'NONE',  ( 50.37043019189811588, -3.055000000000001936, 5.291415217122918513 ) ) ;
#49632=CARTESIAN_POINT ( 'NONE',  ( 104.4958603837962272, -3.974999999999998312, -6.884901960086286188 ) ) ;
#49633=CARTESIAN_POINT ( 'NONE',  ( 68.47502705046289861, -5.819803920172572198, 5.819803920172572198 ) ) ;
#49637=CARTESIAN_POINT ( 'NONE',  ( 61.22916666666665719, 7.950000000000001954, -2.130196079827421762 ) ) ;
#49646=DIRECTION ( 'NONE',  ( 0.000000000000000000, 0.000000000000000000, 1.000000000000000000 ) ) ;
#49647=CARTESIAN_POINT ( 'NONE',  ( 60.81293019189811133, -1.637169565754159617, -6.110000000000001208 ) ) ;
#49648=LINE ( 'NONE', #93826, #129313 ) ;
#49664=ORIENTED_EDGE ( 'NONE', *, *, #101176, .F. ) ;
#49696=CARTESIAN_POINT ( 'NONE',  ( 92.80793019189812298, -6.109999999999998543, 1.637169565754158507 ) ) ;
#49721=CARTESIAN_POINT ( 'NONE',  ( 44.47959685856476852, 6.109999999999999432, 1.637169565754164280 ) ) ;
#49761=DIRECTION ( 'NONE',  ( -1.000000000000000000, -0.000000000000000000, -0.000000000000000000 ) ) ;
#49772=CARTESIAN_POINT ( 'NONE',  ( 77.78709685856478018, 3.054999999999997939, 5.291415217122920289 ) ) ;
#49773=CARTESIAN_POINT ( 'NONE',  ( 74.16252705046288440, 7.949999999999998401, 1.460391307983218338E-15 ) ) ;
#49796=CARTESIAN_POINT ( 'NONE',  ( 90.20419371712957002, -6.884901960086285300, -3.975000000000000089 ) ) ;
#49813=CARTESIAN_POINT ( 'NONE',  ( 85.16709685856477563, -3.055000000000000160, -5.291415217122921177 ) ) ;
#49831=ADVANCED_FACE ( 'NONE', ( #76892 ), #131970, .T. ) ;
#49833=CARTESIAN_POINT ( 'NONE',  ( 77.72959685856477563, -6.110000000000000320, -1.637169565754161393 ) ) ;
#49845=CARTESIAN_POINT ( 'NONE',  ( 33.32919371712955581, -3.975000000000001865, 6.884901960086284411 ) ) ;
#49849=CARTESIAN_POINT ( 'NONE',  ( 65.45833333333332860, 3.974999999999997424, 6.884901960086288852 ) ) ;
#49854=CARTESIAN_POINT ( 'NONE',  ( 53.45419371712956291, 6.884901960086283523, 3.975000000000002753 ) ) ;
#49882=CARTESIAN_POINT ( 'NONE',  ( 74.08376352523143282, -6.110000000000001208, -3.741295971395164515E-16 ) ) ;
#49891=CARTESIAN_POINT ( 'NONE',  ( 108.5004301918981184, -3.055000000000002380, 5.291415217122920289 ) ) ;
#49895=CARTESIAN_POINT ( 'NONE',  ( 129.0581452878471680, 0.000000000000000000, -7.029999999999999361 ) ) ;
#49918=CARTESIAN_POINT ( 'NONE',  ( 90.78752705046288440, 0.000000000000000000, -7.949999999999998401 ) ) ;
#49936=CARTESIAN_POINT ( 'NONE',  ( 73.33333333333332860, -6.884901960086287964, 3.974999999999998312 ) ) ;
#49950=CARTESIAN_POINT ( 'NONE',  ( 118.3500270504628986, -5.819803920172572198, -5.819803920172572198 ) ) ;
#49964=ORIENTED_EDGE ( 'NONE', *, *, #16286, .F. ) ;
#49965=CARTESIAN_POINT ( 'NONE',  ( 83.10416666666668561, 2.130196079827422206, 7.950000000000001954 ) ) ;
#49973=EDGE_LOOP ( 'NONE', ( #13790, #84954, #103102, #110712 ) ) ;
#49990=CARTESIAN_POINT ( 'NONE',  ( 99.45876352523144703, 0.000000000000000000, -6.110000000000001208 ) ) ;
#49997=CARTESIAN_POINT ( 'NONE',  ( 75.81250000000000000, 5.819803920172571310, 5.819803920172576639 ) ) ;
#50000=CARTESIAN_POINT ( 'NONE',  ( 101.4120968585647802, 5.291415217122921177, -3.054999999999994831 ) ) ;
#50025=CARTESIAN_POINT ( 'NONE',  ( 111.1829301918981230, -1.637169565754158951, -6.109999999999998543 ) ) ;
#50047=CARTESIAN_POINT ( 'NONE',  ( 37.24543019189811588, -5.291415217122918513, -3.055000000000000160 ) ) ;
#50076=CARTESIAN_POINT ( 'NONE',  ( 150.3000000000000114, 0.000000000000000000, 0.000000000000000000 ) ) ;
#50085=CARTESIAN_POINT ( 'NONE',  ( 103.5995968585647802, -6.109999999999998543, -1.637169565754160727 ) ) ;
#50126=CARTESIAN_POINT ( 'NONE',  ( 28.51669371712955581, 7.950000000000000178, -2.130196079827421318 ) ) ;
#50130=CARTESIAN_POINT ( 'NONE',  ( 110.8125000000000000, 5.819803920172571310, 5.819803920172575751 ) ) ;
#50143=CARTESIAN_POINT ( 'NONE',  ( 110.6879301918981184, 6.110000000000002984, -1.637169565754156730 ) ) ;
#50153=CARTESIAN_POINT ( 'NONE',  ( 42.51669371712955581, 7.950000000000001066, -2.130196079827421318 ) ) ;
#50159=CARTESIAN_POINT ( 'NONE',  ( 32.79166666666666430, 3.975000000000003642, -6.884901960086285300 ) ) ;
#50164=DIRECTION ( 'NONE',  ( 0.000000000000000000, 0.000000000000000000, 1.000000000000000000 ) ) ;
#50170=CARTESIAN_POINT ( 'NONE',  ( 25.37543019189810067, -5.291415217122920289, -3.055000000000001492 ) ) ;
#50183=CARTESIAN_POINT ( 'NONE',  ( 53.08376352523143282, -6.110000000000001208, -3.741295971395164515E-16 ) ) ;
#50193=CARTESIAN_POINT ( 'NONE',  ( 49.49543019189811588, 5.291415217122916737, 3.055000000000001936 ) ) ;
#50204=PRODUCT_DEFINITION_CONTEXT ( 'detailed design', #23477, 'design' ) ;
#50221=CARTESIAN_POINT ( 'NONE',  ( 63.93293019189812298, 1.637169565754156508, 6.110000000000000320 ) ) ;
#50280=ORIENTED_EDGE ( 'NONE', *, *, #39228, .F. ) ;
#50299=CARTESIAN_POINT ( 'NONE',  ( 48.62043019189811588, 3.055000000000002380, -5.291415217122917625 ) ) ;
#50319=CARTESIAN_POINT ( 'NONE',  ( 62.20419371712955581, -6.884901960086285300, -3.975000000000000089 ) ) ;
#50324=CARTESIAN_POINT ( 'NONE',  ( 63.70833333333332860, -3.974999999999999201, -6.884901960086287964 ) ) ;
#50332=CARTESIAN_POINT ( 'NONE',  ( 58.47959685856477563, 6.109999999999999432, 1.637169565754164280 ) ) ;
#50338=CARTESIAN_POINT ( 'NONE',  ( 0.000000000000000000, 0.000000000000000000, 0.000000000000000000 ) ) ;
#50344=CARTESIAN_POINT ( 'NONE',  ( 101.2875270504628986, 0.000000000000000000, -7.949999999999998401 ) ) ;
#50345=ORIENTED_EDGE ( 'NONE', *, *, #73856, .F. ) ;
#50347=LINE ( 'NONE', #7522, #18267 ) ;
#50359=CARTESIAN_POINT ( 'NONE',  ( 110.9125270504628986, -7.949999999999998401, -4.867971026610728450E-16 ) ) ;
#50387=CARTESIAN_POINT ( 'NONE',  ( 91.34959685856478018, 6.109999999999996767, 1.637169565754163836 ) ) ;
#50405=DIRECTION ( 'NONE',  ( 0.000000000000000000, 0.000000000000000000, 1.000000000000000000 ) ) ;
#50415=CARTESIAN_POINT ( 'NONE',  ( 41.85459685856476852, -1.637169565754161615, 6.110000000000000320 ) ) ;
#50449=FACE_OUTER_BOUND ( 'NONE', #45296, .T. ) ;
#50453=CARTESIAN_POINT ( 'NONE',  ( 96.37500000000000000, 7.950000000000000178, 1.460391307983218535E-15 ) ) ;
#50465=CARTESIAN_POINT ( 'NONE',  ( 75.16209685856478018, -5.291415217122919401, 3.054999999999998384 ) ) ;
#50488=CARTESIAN_POINT ( 'NONE',  ( 94.57919371712955581, 3.975000000000002753, -6.884901960086283523 ) ) ;
#50501=CARTESIAN_POINT ( 'NONE',  ( 82.68793019189809002, 6.110000000000002984, -1.637169565754156730 ) ) ;
#50509=CARTESIAN_POINT ( 'NONE',  ( 117.3291937171295558, -3.975000000000001865, 6.884901960086284411 ) ) ;
#50516=CARTESIAN_POINT ( 'NONE',  ( 58.75000000000000000, -9.735942053221458872E-16, 7.950000000000000178 ) ) ;
#50521=CARTESIAN_POINT ( 'NONE',  ( 70.00043019189810423, -3.055000000000002380, 5.291415217122920289 ) ) ;
#50555=CARTESIAN_POINT ( 'NONE',  ( 0.000000000000000000, 0.000000000000000000, 7.950000000000000178 ) ) ;
#50575=CARTESIAN_POINT ( 'NONE',  ( 76.41709685856476142, 3.054999999999998828, 5.291415217122922066 ) ) ;
#50581=CARTESIAN_POINT ( 'NONE',  ( 104.8545968585647756, -1.637169565754161615, 6.110000000000000320 ) ) ;
#50609=( BOUNDED_CURVE ( )  B_SPLINE_CURVE ( 2, ( #26946, #80637, #112533, #5163, #101649, #58209, #13191, #114656, #71195, #69786, #57467, #46625, #90804 ),
 .UNSPECIFIED., .F., .T. ) 
 B_SPLINE_CURVE_WITH_KNOTS ( ( 3, 2, 2, 2, 2, 2, 3 ),
 ( 0.2166666666666666741, 0.2194444444444444420, 0.2222222222222222099, 0.2250000000000000056, 0.2277777777777777735, 0.2305555555555555691, 0.2333333333333333370 ),
 .UNSPECIFIED. ) 
 CURVE ( )  GEOMETRIC_REPRESENTATION_ITEM ( )  RATIONAL_B_SPLINE_CURVE ( ( 1.000000000000000000, 0.9659258262890683122, 1.000000000000000000, 0.9659258262890683122, 1.000000000000000000, 0.9659258262890683122, 1.000000000000000000, 0.9659258262890683122, 1.000000000000000000, 0.9659258262890683122, 1.000000000000000000, 0.9659258262890683122, 1.000000000000000000 ) ) 
 REPRESENTATION_ITEM ( '' )  );
#50638=ORIENTED_EDGE ( 'NONE', *, *, #61521, .T. ) ;
#50644=CARTESIAN_POINT ( 'NONE',  ( 123.8916937171295416, 2.130196079827421762, 7.950000000000001066 ) ) ;
#50657=CARTESIAN_POINT ( 'NONE',  ( 87.18749999999998579, -5.819803920172573086, 5.819803920172572198 ) ) ;
#50677=VECTOR ( 'NONE', #133865, 1000.000000000000000 ) ;
#50688=CARTESIAN_POINT ( 'NONE',  ( 98.29209685856477563, -5.291415217122921177, 3.054999999999999272 ) ) ;
#50700=CARTESIAN_POINT ( 'NONE',  ( 91.05793019189812298, 6.110000000000000320, -1.637169565754156064 ) ) ;
#50727=CARTESIAN_POINT ( 'NONE',  ( 112.6412635252314658, 4.472830434245835818, 4.472830434245840259 ) ) ;
#50745=ORIENTED_EDGE ( 'NONE', *, *, #15485, .F. ) ;
#50751=CARTESIAN_POINT ( 'NONE',  ( 30.53709685856477307, -3.054999999999998828, -5.291415217122919401 ) ) ;
#50786=CARTESIAN_POINT ( 'NONE',  ( 100.2454301918981230, -5.291415217122919401, -3.055000000000000604 ) ) ;
#50792=EDGE_LOOP ( 'NONE', ( #131013, #113991, #65935, #10044 ) ) ;
#50838=CARTESIAN_POINT ( 'NONE',  ( 112.2708333333333144, -7.949999999999999289, -2.130196079827426203 ) ) ;
#50849=CARTESIAN_POINT ( 'NONE',  ( 102.0837635252314328, -6.110000000000001208, -3.741295971395164515E-16 ) ) ;
#50858=CARTESIAN_POINT ( 'NONE',  ( 36.24586038379622011, 3.974999999999996980, 6.884901960086287964 ) ) ;
#50865=CARTESIAN_POINT ( 'NONE',  ( 25.64583333333332504, 2.130196079827431976, -7.949999999999999289 ) ) ;
#50876=CARTESIAN_POINT ( 'NONE',  ( 25.95876352523143638, 0.000000000000000000, -6.110000000000001208 ) ) ;
#50885=( BOUNDED_CURVE ( )  B_SPLINE_CURVE ( 2, ( #81816, #38280, #47076, #102116, #82499, #101383, #81084, #13642, #79694, #92631, #123876, #2028, #2778 ),
 .UNSPECIFIED., .F., .T. ) 
 B_SPLINE_CURVE_WITH_KNOTS ( ( 3, 2, 2, 2, 2, 2, 3 ),
 ( 0.2999999999999999889, 0.3027777777777777568, 0.3055555555555555802, 0.3083333333333333481, 0.3111111111111111160, 0.3138888888888888840, 0.3166666666666666519 ),
 .UNSPECIFIED. ) 
 CURVE ( )  GEOMETRIC_REPRESENTATION_ITEM ( )  RATIONAL_B_SPLINE_CURVE ( ( 1.000000000000000000, 0.9659258262890683122, 1.000000000000000000, 0.9659258262890683122, 1.000000000000000000, 0.9659258262890683122, 1.000000000000000000, 0.9659258262890683122, 1.000000000000000000, 0.9659258262890683122, 1.000000000000000000, 0.9659258262890683122, 1.000000000000000000 ) ) 
 REPRESENTATION_ITEM ( '' )  );
#50890=CARTESIAN_POINT ( 'NONE',  ( 46.37543019189810423, -5.291415217122920289, -3.055000000000001492 ) ) ;
#50897=AXIS2_PLACEMENT_3D ( 'NONE', #99114, #88285, #143358 ) ;
#50900=CARTESIAN_POINT ( 'NONE',  ( 51.68293019189811588, -1.637169565754158951, -6.109999999999998543 ) ) ;
#50930=DIRECTION ( 'NONE',  ( -1.000000000000000000, -0.000000000000000000, -0.000000000000000000 ) ) ;
#50933=CARTESIAN_POINT ( 'NONE',  ( 57.95376352523144448, -6.109999999999998543, -3.741295971395162543E-16 ) ) ;
#50941=CARTESIAN_POINT ( 'NONE',  ( 34.39583333333332860, -2.130196079827351596, 7.950000000000043698 ) ) ;
#50943=CARTESIAN_POINT ( 'NONE',  ( 102.2083333333333286, -3.974999999999999201, -6.884901960086287964 ) ) ;
#50953=ORIENTED_EDGE ( 'NONE', *, *, #59774, .T. ) ;
#50973=CARTESIAN_POINT ( 'NONE',  ( 108.6250000000000000, -7.950000000000000178, -4.867971026610729436E-16 ) ) ;
#51007=CARTESIAN_POINT ( 'NONE',  ( 46.57876352523145158, -7.482591942790327058E-16, 6.109999999999999432 ) ) ;
#51013=AXIS2_PLACEMENT_3D ( 'NONE', #59771, #48889, #69217 ) ;
#51018=DIRECTION ( 'NONE',  ( -1.000000000000000000, -0.000000000000000000, -0.000000000000000000 ) ) ;
#51020=CARTESIAN_POINT ( 'NONE',  ( 82.08333333333334281, 6.884901960086290629, -3.974999999999994316 ) ) ;
#51030=CARTESIAN_POINT ( 'NONE',  ( 67.74586038379622721, 3.974999999999996980, 6.884901960086287964 ) ) ;
#51036=CARTESIAN_POINT ( 'NONE',  ( 53.64583333333332860, 2.130196079827431976, -7.949999999999999289 ) ) ;
#51046=CARTESIAN_POINT ( 'NONE',  ( 53.37543019189811133, -5.291415217122920289, -3.055000000000001492 ) ) ;
#51054=LINE ( 'NONE', #106836, #46692 ) ;
#51059=CARTESIAN_POINT ( 'NONE',  ( 99.97502705046289861, -5.819803920172573086, 5.819803920172573086 ) ) ;
#51067=( BOUNDED_CURVE ( )  B_SPLINE_CURVE ( 2, ( #33028, #11189, #55470, #99655, #122122, #328, #88818, #133048, #22776, #67056, #69199, #138737, #91649 ),
 .UNSPECIFIED., .F., .T. ) 
 B_SPLINE_CURVE_WITH_KNOTS ( ( 3, 2, 2, 2, 2, 2, 3 ),
 ( 0.9166666666666666297, 0.9194444444444443976, 0.9222222222222222765, 0.9250000000000000444, 0.9277777777777778123, 0.9305555555555555802, 0.9333333333333333481 ),
 .UNSPECIFIED. ) 
 CURVE ( )  GEOMETRIC_REPRESENTATION_ITEM ( )  RATIONAL_B_SPLINE_CURVE ( ( 1.000000000000000000, 0.9659258262890683122, 1.000000000000000000, 0.9659258262890683122, 1.000000000000000000, 0.9659258262890683122, 1.000000000000000000, 0.9659258262890683122, 1.000000000000000000, 0.9659258262890683122, 1.000000000000000000, 0.9659258262890683122, 1.000000000000000000 ) ) 
 REPRESENTATION_ITEM ( '' )  );
#51071=CARTESIAN_POINT ( 'NONE',  ( 89.03752705046288440, -9.735942053221456900E-16, 7.949999999999998401 ) ) ;
#51072=CARTESIAN_POINT ( 'NONE',  ( 76.03709685856478018, -3.054999999999998828, -5.291415217122919401 ) ) ;
#51075=CARTESIAN_POINT ( 'NONE',  ( 73.28752705046288440, 0.000000000000000000, -7.949999999999998401 ) ) ;
#51107=CARTESIAN_POINT ( 'NONE',  ( 84.78709685856478018, 3.054999999999997495, 5.291415217122919401 ) ) ;
#51132=CARTESIAN_POINT ( 'NONE',  ( 43.45876352523143993, 0.000000000000000000, -6.110000000000001208 ) ) ;
#51178=CARTESIAN_POINT ( 'NONE',  ( 72.68293019189810877, -1.637169565754159173, -6.109999999999999432 ) ) ;
#51191=AXIS2_PLACEMENT_3D ( 'NONE', #47880, #92044, #5000 ) ;
#51206=CARTESIAN_POINT ( 'NONE',  ( 97.64169371712954160, -2.130196079827424871, -7.949999999999999289 ) ) ;
#51216=FACE_OUTER_BOUND ( 'NONE', #43809, .T. ) ;
#51224=CARTESIAN_POINT ( 'NONE',  ( 87.50043019189810423, -3.055000000000002380, 5.291415217122920289 ) ) ;
#51245=CARTESIAN_POINT ( 'NONE',  ( 71.60459685856477563, 1.637169565754164946, -6.109999999999999432 ) ) ;
#51259=CARTESIAN_POINT ( 'NONE',  ( 34.35002705046289151, -5.819803920172573086, -5.819803920172573086 ) ) ;
#51285=ORIENTED_EDGE ( 'NONE', *, *, #635, .T. ) ;
#51303=CARTESIAN_POINT ( 'NONE',  ( 73.20876352523143282, -7.482591942790329030E-16, 6.110000000000001208 ) ) ;
#51307=CARTESIAN_POINT ( 'NONE',  ( 108.9379301918980758, -6.110000000000001208, 1.637169565754158951 ) ) ;
#51341=ORIENTED_EDGE ( 'NONE', *, *, #129731, .F. ) ;
#51354=CARTESIAN_POINT ( 'NONE',  ( 41.24999999999999289, -9.735942053221458872E-16, 7.950000000000000178 ) ) ;
#51357=CARTESIAN_POINT ( 'NONE',  ( 74.35416666666667140, -2.130196079827425759, -7.950000000000000178 ) ) ;
#51372=CARTESIAN_POINT ( 'NONE',  ( 120.3916937171295700, 2.130196079827421762, 7.950000000000001066 ) ) ;
#51389=CARTESIAN_POINT ( 'NONE',  ( 79.89583333333331439, -2.130196079827427091, 7.949999999999999289 ) ) ;
#51393=CARTESIAN_POINT ( 'NONE',  ( 91.22502705046289861, 5.819803920172573974, -5.819803920172573086 ) ) ;
#51415=CARTESIAN_POINT ( 'NONE',  ( 97.85459685856477563, -1.637169565754161615, 6.110000000000000320 ) ) ;
#51426=CARTESIAN_POINT ( 'NONE',  ( 94.70376352523145158, 6.109999999999998543, 1.122388791418548911E-15 ) ) ;
#51434=DIRECTION ( 'NONE',  ( 1.000000000000000000, 0.000000000000000000, 1.899332272967292827E-15 ) ) ;
#51474=CARTESIAN_POINT ( 'NONE',  ( 33.01626352523144448, -4.472830434245838482, 4.472830434245838482 ) ) ;
#51482=AXIS2_PLACEMENT_3D ( 'NONE', #67026, #21377, #10473 ) ;
#51514=CARTESIAN_POINT ( 'NONE',  ( 91.05793019189812298, 6.110000000000001208, -1.637169565754156286 ) ) ;
#51547=CARTESIAN_POINT ( 'NONE',  ( 27.00000000000001421, 3.441786896390103934, 7.166352137582786774 ) ) ;
#51553=CARTESIAN_POINT ( 'NONE',  ( 46.93749999999999289, 5.819803920172574863, -5.819803920172573086 ) ) ;
#51565=CARTESIAN_POINT ( 'NONE',  ( 115.3333333333333286, -6.884901960086287964, 3.974999999999998312 ) ) ;
#51566=ORIENTED_EDGE ( 'NONE', *, *, #113714, .T. ) ;
#51579=CARTESIAN_POINT ( 'NONE',  ( 102.3754301918981184, -5.291415217122920289, -3.055000000000001492 ) ) ;
#51585=CARTESIAN_POINT ( 'NONE',  ( 27.78752705046289151, 0.000000000000000000, -7.949999999999998401 ) ) ;
#51590=CARTESIAN_POINT ( 'NONE',  ( 24.62499999999999289, -7.950000000000000178, -4.867971026610729436E-16 ) ) ;
#51603=CARTESIAN_POINT ( 'NONE',  ( 122.9954301918981230, 5.291415217122916737, 3.055000000000001936 ) ) ;
#51614=CARTESIAN_POINT ( 'NONE',  ( 45.20876352523143993, -7.482591942790329030E-16, 6.110000000000001208 ) ) ;
#51622=CARTESIAN_POINT ( 'NONE',  ( 35.49543019189811588, 5.291415217122916737, 3.055000000000001936 ) ) ;
#51631=CARTESIAN_POINT ( 'NONE',  ( 59.87086038379622721, 6.884901960086289741, -3.974999999999993427 ) ) ;
#51649=CARTESIAN_POINT ( 'NONE',  ( 59.41209685856478728, 5.291415217122921177, -3.054999999999994831 ) ) ;
#51684=CARTESIAN_POINT ( 'NONE',  ( 127.5162635252314516, -4.472830434245839371, 4.472830434245839371 ) ) ;
#51724=LINE ( 'NONE', #123417, #120763 ) ;
#51727=CARTESIAN_POINT ( 'NONE',  ( 41.76626352523145158, 4.472830434245839371, -4.472830434245839371 ) ) ;
#51753=CARTESIAN_POINT ( 'NONE',  ( 103.3291937171295700, -3.975000000000001865, 6.884901960086284411 ) ) ;
#51755=CARTESIAN_POINT ( 'NONE',  ( 70.51669371712954160, 7.950000000000001066, -2.130196079827421318 ) ) ;
#51760=CARTESIAN_POINT ( 'NONE',  ( 53.20833333333332860, -3.974999999999999201, -6.884901960086287964 ) ) ;
#51767=CARTESIAN_POINT ( 'NONE',  ( 51.62543019189811133, 5.291415217122919401, 3.055000000000002824 ) ) ;
#51784=CARTESIAN_POINT ( 'NONE',  ( 127.0000000000000000, 1.564650039245123914, 6.154215649023822010 ) ) ;
#51796=CARTESIAN_POINT ( 'NONE',  ( 78.66209685856479439, -5.291415217122919401, 3.054999999999997939 ) ) ;
#51824=CARTESIAN_POINT ( 'NONE',  ( 86.09959685856478018, -6.109999999999997655, -1.637169565754160283 ) ) ;
#51845=CARTESIAN_POINT ( 'NONE',  ( 34.85459685856477563, -1.637169565754161615, 6.110000000000000320 ) ) ;
#51853=( BOUNDED_CURVE ( )  B_SPLINE_CURVE ( 2, ( #54044, #53275, #304, #33008, #76496, #119936, #9776, #109813, #97489, #58157, #54737, #22759, #64178 ),
 .UNSPECIFIED., .F., .T. ) 
 B_SPLINE_CURVE_WITH_KNOTS ( ( 3, 2, 2, 2, 2, 2, 3 ),
 ( 0.2999999999999999889, 0.3027777777777777568, 0.3055555555555555802, 0.3083333333333333481, 0.3111111111111111160, 0.3138888888888888840, 0.3166666666666666519 ),
 .UNSPECIFIED. ) 
 CURVE ( )  GEOMETRIC_REPRESENTATION_ITEM ( )  RATIONAL_B_SPLINE_CURVE ( ( 1.000000000000000000, 0.9659258262890683122, 1.000000000000000000, 0.9659258262890683122, 1.000000000000000000, 0.9659258262890683122, 1.000000000000000000, 0.9659258262890683122, 1.000000000000000000, 0.9659258262890683122, 1.000000000000000000, 0.9659258262890683122, 1.000000000000000000 ) ) 
 REPRESENTATION_ITEM ( '' )  );
#51901=CARTESIAN_POINT ( 'NONE',  ( 72.39126352523145158, -4.472830434245839371, -4.472830434245839371 ) ) ;
#51906=ORIENTED_EDGE ( 'NONE', *, *, #135838, .T. ) ;
#51925=CARTESIAN_POINT ( 'NONE',  ( 97.49586038379624142, -3.974999999999998312, -6.884901960086286188 ) ) ;
#51926=CARTESIAN_POINT ( 'NONE',  ( 0.000000000000000000, 0.000000000000000000, 6.349999999999997868 ) ) ;
#51940=CARTESIAN_POINT ( 'NONE',  ( 81.52126352523141861, -4.472830434245839371, -4.472830434245840259 ) ) ;
#51958=CARTESIAN_POINT ( 'NONE',  ( 76.12543019189810423, 5.291415217122919401, 3.055000000000002824 ) ) ;
#51967=CARTESIAN_POINT ( 'NONE',  ( 36.53752705046288440, -9.735942053221456900E-16, 7.949999999999998401 ) ) ;
#51997=CARTESIAN_POINT ( 'NONE',  ( 27.00000000000001066, -5.997342894908404887, -3.744407088454140276 ) ) ;
#52006=CARTESIAN_POINT ( 'NONE',  ( 67.81293019189809002, -1.637169565754159617, -6.110000000000001208 ) ) ;
#52014=CARTESIAN_POINT ( 'NONE',  ( 97.85459685856477563, -1.637169565754161615, 6.110000000000000320 ) ) ;
#52059=CARTESIAN_POINT ( 'NONE',  ( 25.81293019189810778, -1.637169565754159617, -6.110000000000001208 ) ) ;
#52078=CARTESIAN_POINT ( 'NONE',  ( 119.9541937171295700, 6.884901960086283523, 3.975000000000002753 ) ) ;
#52093=CARTESIAN_POINT ( 'NONE',  ( 29.53752705046289151, -9.735942053221456900E-16, 7.949999999999998401 ) ) ;
#52101=CARTESIAN_POINT ( 'NONE',  ( 40.52083333333332860, 7.949999999999998401, 2.130196079827431532 ) ) ;
#52111=CARTESIAN_POINT ( 'NONE',  ( 104.7087635252314328, -7.482591942790329030E-16, 6.110000000000001208 ) ) ;
#52120=CARTESIAN_POINT ( 'NONE',  ( 99.66209685856478018, -5.291415217122919401, 3.054999999999997939 ) ) ;
#52154=EDGE_CURVE ( 'NONE', #136489, #95449, #50347, .T. ) ;
#52168=CARTESIAN_POINT ( 'NONE',  ( 27.32876352523144803, 0.000000000000000000, -6.109999999999998543 ) ) ;
#52203=CARTESIAN_POINT ( 'NONE',  ( 96.30793019189810877, -6.109999999999999432, 1.637169565754158507 ) ) ;
#52255=CARTESIAN_POINT ( 'NONE',  ( 109.0625000000000000, -5.819803920172572198, -5.819803920172573086 ) ) ;
#52266=CARTESIAN_POINT ( 'NONE',  ( 100.7712635252314328, 4.472830434245839371, 4.472830434245842035 ) ) ;
#52278=CARTESIAN_POINT ( 'NONE',  ( 27.83333333333332149, -6.884901960086287964, 3.974999999999998312 ) ) ;
#52287=CARTESIAN_POINT ( 'NONE',  ( 121.3912635252314374, -4.472830434245839371, -4.472830434245839371 ) ) ;
#52297=CARTESIAN_POINT ( 'NONE',  ( 44.18793019189810423, 6.110000000000002984, -1.637169565754156730 ) ) ;
#52304=( BOUNDED_CURVE ( )  B_SPLINE_CURVE ( 2, ( #46765, #48144, #37261, #114103, #14787, #24934, #34404, #35143, #102536, #67791, #92324, #59060, #114785 ),
 .UNSPECIFIED., .F., .T. ) 
 B_SPLINE_CURVE_WITH_KNOTS ( ( 3, 2, 2, 2, 2, 2, 3 ),
 ( 0.5999999999999999778, 0.6027777777777777457, 0.6055555555555555136, 0.6083333333333332815, 0.6111111111111111605, 0.6138888888888889284, 0.6166666666666666963 ),
 .UNSPECIFIED. ) 
 CURVE ( )  GEOMETRIC_REPRESENTATION_ITEM ( )  RATIONAL_B_SPLINE_CURVE ( ( 1.000000000000000000, 0.9659258262890683122, 1.000000000000000000, 0.9659258262890683122, 1.000000000000000000, 0.9659258262890683122, 1.000000000000000000, 0.9659258262890683122, 1.000000000000000000, 0.9659258262890683122, 1.000000000000000000, 0.9659258262890683122, 1.000000000000000000 ) ) 
 REPRESENTATION_ITEM ( '' )  );
#52308=CARTESIAN_POINT ( 'NONE',  ( 43.80793019189810877, -6.109999999999998543, 1.637169565754158063 ) ) ;
#52317=CARTESIAN_POINT ( 'NONE',  ( 79.70419371712955581, -6.884901960086285300, -3.975000000000000089 ) ) ;
#52319=CARTESIAN_POINT ( 'NONE',  ( 43.82919371712955581, -3.975000000000001865, 6.884901960086284411 ) ) ;
#52338=CARTESIAN_POINT ( 'NONE',  ( 54.74543019189812298, -5.291415217122918513, -3.055000000000000160 ) ) ;
#52371=CARTESIAN_POINT ( 'NONE',  ( 116.2870968585647802, 3.054999999999997939, 5.291415217122920289 ) ) ;
#52381=EDGE_CURVE ( 'NONE', #83142, #32075, #79027, .T. ) ;
#52410=CARTESIAN_POINT ( 'NONE',  ( 34.76626352523145158, 4.472830434245839371, -4.472830434245839371 ) ) ;
#52434=CARTESIAN_POINT ( 'NONE',  ( 59.57919371712955581, 3.975000000000002753, -6.884901960086283523 ) ) ;
#52440=CARTESIAN_POINT ( 'NONE',  ( 58.60416666666665719, 2.130196079827422206, 7.950000000000001954 ) ) ;
#52447=CARTESIAN_POINT ( 'NONE',  ( 45.20876352523143993, -7.482591942790329030E-16, 6.110000000000001208 ) ) ;
#52449=EDGE_CURVE ( 'NONE', #40381, #142459, #56809, .T. ) ;
#52474=CARTESIAN_POINT ( 'NONE',  ( 65.09959685856478018, -6.109999999999997655, -1.637169565754160283 ) ) ;
#52506=ORIENTED_EDGE ( 'NONE', *, *, #120905, .T. ) ;
#52508=CARTESIAN_POINT ( 'NONE',  ( 86.82876352523145158, 0.000000000000000000, -6.109999999999998543 ) ) ;
#52534=CARTESIAN_POINT ( 'NONE',  ( 37.91709685856477563, 3.054999999999998828, 5.291415217122922066 ) ) ;
#52536=CARTESIAN_POINT ( 'NONE',  ( 45.47916666666666430, -7.950000000000000178, 2.130196079827424427 ) ) ;
#52576=DIRECTION ( 'NONE',  ( -1.000000000000000000, -0.000000000000000000, -0.000000000000000000 ) ) ;
#52585=CARTESIAN_POINT ( 'NONE',  ( 68.89126352523142316, -4.472830434245839371, -4.472830434245839371 ) ) ;
#52611=CARTESIAN_POINT ( 'NONE',  ( 87.57919371712957002, 3.975000000000002753, -6.884901960086283523 ) ) ;
#52622=CARTESIAN_POINT ( 'NONE',  ( 76.70876352523144703, -7.482591942790329030E-16, 6.110000000000001208 ) ) ;
#52645=CARTESIAN_POINT ( 'NONE',  ( 77.87543019189810423, -5.291415217122920289, -3.055000000000001492 ) ) ;
#52698=CARTESIAN_POINT ( 'NONE',  ( 67.08376352523143282, -6.110000000000001208, -3.741295971395164515E-16 ) ) ;
#52705=CARTESIAN_POINT ( 'NONE',  ( 101.5004301918981042, -3.055000000000002380, 5.291415217122920289 ) ) ;
#52711=CARTESIAN_POINT ( 'NONE',  ( 90.68750000000001421, -5.819803920172573974, 5.819803920172573086 ) ) ;
#52719=CARTESIAN_POINT ( 'NONE',  ( 125.9120968585647802, 5.291415217122921177, -3.054999999999994831 ) ) ;
#52735=CARTESIAN_POINT ( 'NONE',  ( 10.46945953031644372, -8.432637487761466488, -4.375000000000003553 ) ) ;
#52746=CARTESIAN_POINT ( 'NONE',  ( 32.52126352523142572, -4.472830434245839371, -4.472830434245840259 ) ) ;
#52751=FACE_OUTER_BOUND ( 'NONE', #114051, .T. ) ;
#52754=CARTESIAN_POINT ( 'NONE',  ( 42.27083333333332149, -7.949999999999998401, -2.130196079827426203 ) ) ;
#52765=CARTESIAN_POINT ( 'NONE',  ( 126.5166937171295700, 7.950000000000001066, -2.130196079827421318 ) ) ;
#52784=ORIENTED_EDGE ( 'NONE', *, *, #13700, .F. ) ;
#52790=CARTESIAN_POINT ( 'NONE',  ( 39.79166666666665719, 3.975000000000003642, -6.884901960086285300 ) ) ;
#52791=CARTESIAN_POINT ( 'NONE',  ( 70.56250000000000000, -5.819803920172573086, -5.819803920172573974 ) ) ;
#52799=CARTESIAN_POINT ( 'NONE',  ( 103.8337635252314328, 6.110000000000001208, 1.122388791418549305E-15 ) ) ;
#52804=CARTESIAN_POINT ( 'NONE',  ( 84.51669371712955581, 7.950000000000000178, -2.130196079827421318 ) ) ;
#52809=CARTESIAN_POINT ( 'NONE',  ( 97.32876352523145158, 0.000000000000000000, -6.109999999999998543 ) ) ;
#52816=ORIENTED_EDGE ( 'NONE', *, *, #60056, .F. ) ;
#52818=EDGE_CURVE ( 'NONE', #53423, #26730, #73371, .T. ) ;
#52851=ORIENTED_EDGE ( 'NONE', *, *, #73633, .F. ) ;
#52859=CARTESIAN_POINT ( 'NONE',  ( 32.14126352523144448, 4.472830434245835818, 4.472830434245840259 ) ) ;
#52862=CARTESIAN_POINT ( 'NONE',  ( 124.1045968585647756, 1.637169565754164946, -6.109999999999999432 ) ) ;
#52889=CARTESIAN_POINT ( 'NONE',  ( 90.18293019189809456, -1.637169565754159173, -6.109999999999999432 ) ) ;
#52934=CARTESIAN_POINT ( 'NONE',  ( 0.000000000000000000, 0.000000000000000000, 0.000000000000000000 ) ) ;
#52946=CARTESIAN_POINT ( 'NONE',  ( 112.8541666666666572, -2.130196079827425315, -7.950000000000001066 ) ) ;
#52963=CARTESIAN_POINT ( 'NONE',  ( 101.0629301918980900, 1.637169565754157174, 6.110000000000002984 ) ) ;
#52973=CARTESIAN_POINT ( 'NONE',  ( 31.43336038379622721, 2.130196079827431532, -7.949999999999997513 ) ) ;
#52978=CARTESIAN_POINT ( 'NONE',  ( 26.52083333333332860, 7.949999999999999289, 2.130196079827431532 ) ) ;
#52990=CARTESIAN_POINT ( 'NONE',  ( 120.5162635252314374, -4.472830434245839371, 4.472830434245839371 ) ) ;
#52999=CARTESIAN_POINT ( 'NONE',  ( 42.87543019189810423, -5.291415217122920289, -3.055000000000001492 ) ) ;
#53008=CARTESIAN_POINT ( 'NONE',  ( 36.80793019189810167, -6.109999999999998543, 1.637169565754158063 ) ) ;
#53040=CARTESIAN_POINT ( 'NONE',  ( 59.12043019189810877, 3.055000000000001936, -5.291415217122916737 ) ) ;
#53072=DIRECTION ( 'NONE',  ( -1.000000000000000000, -0.000000000000000000, -0.000000000000000000 ) ) ;
#53074=CARTESIAN_POINT ( 'NONE',  ( 119.2037635252314658, 6.109999999999999432, 1.122388791418549108E-15 ) ) ;
#53106=CARTESIAN_POINT ( 'NONE',  ( 150.3000000000000114, 5.817072295949924468E-16, -4.749999999999997335 ) ) ;
#53113=CARTESIAN_POINT ( 'NONE',  ( 34.03709685856478018, -3.054999999999999272, -5.291415217122919401 ) ) ;
#53137=CARTESIAN_POINT ( 'NONE',  ( 79.45833333333332860, 3.974999999999997424, 6.884901960086288852 ) ) ;
#53143=CARTESIAN_POINT ( 'NONE',  ( 54.76669371712954870, -7.949999999999999289, 2.130196079827424427 ) ) ;
#53148=CARTESIAN_POINT ( 'NONE',  ( 56.85416666666666430, -2.130196079827425315, -7.950000000000001066 ) ) ;
#53158=CARTESIAN_POINT ( 'NONE',  ( 44.77126352523143282, 4.472830434245839371, 4.472830434245842035 ) ) ;
#53167=CARTESIAN_POINT ( 'NONE',  ( 80.43336038379622721, 2.130196079827431532, -7.949999999999996625 ) ) ;
#53178=CARTESIAN_POINT ( 'NONE',  ( 83.12543019189810423, 5.291415217122919401, 3.055000000000002824 ) ) ;
#53187=CARTESIAN_POINT ( 'NONE',  ( 88.45419371712957002, 6.884901960086283523, 3.975000000000002753 ) ) ;
#53188=CARTESIAN_POINT ( 'NONE',  ( 64.07876352523145158, -7.482591942790325086E-16, 6.109999999999998543 ) ) ;
#53195=DIRECTION ( 'NONE',  ( 1.000000000000000000, 0.000000000000000000, 0.000000000000000000 ) ) ;
#53215=CARTESIAN_POINT ( 'NONE',  ( 81.14126352523143737, 4.472830434245835818, 4.472830434245840259 ) ) ;
#53239=CARTESIAN_POINT ( 'NONE',  ( 38.64626352523143993, -4.472830434245840259, 4.472830434245838482 ) ) ;
#53275=CARTESIAN_POINT ( 'NONE',  ( 97.64169371712954160, -2.130196079827424871, -7.949999999999998401 ) ) ;
#53296=CARTESIAN_POINT ( 'NONE',  ( 65.68293019189810877, -1.637169565754159173, -6.109999999999999432 ) ) ;
#53302=CARTESIAN_POINT ( 'NONE',  ( 83.97916666666665719, -7.950000000000000178, 2.130196079827424427 ) ) ;
#53323=CARTESIAN_POINT ( 'NONE',  ( 87.14169371712958423, -2.130196079827424871, -7.949999999999999289 ) ) ;
#53338=CARTESIAN_POINT ( 'NONE',  ( 75.97959685856477563, 6.109999999999999432, 1.637169565754164280 ) ) ;
#53363=CARTESIAN_POINT ( 'NONE',  ( 61.54209685856476852, 5.291415217122923842, -3.054999999999996163 ) ) ;
#53382=VECTOR ( 'NONE', #43874, 1000.000000000000000 ) ;
#53390=CARTESIAN_POINT ( 'NONE',  ( 127.2844355792472584, -1.701477371938903360, 6.349999999999264233 ) ) ;
#53398=CARTESIAN_POINT ( 'NONE',  ( 109.5787635252314516, -7.482591942790325086E-16, 6.109999999999998543 ) ) ;
#53423=VERTEX_POINT ( 'NONE', #74974 ) ;
#53424=CARTESIAN_POINT ( 'NONE',  ( 60.08376352523143993, -6.110000000000001208, -3.741295971395164515E-16 ) ) ;
#53430=CARTESIAN_POINT ( 'NONE',  ( 96.39626352523141861, 4.472830434245840259, -4.472830434245838482 ) ) ;
#53437=CARTESIAN_POINT ( 'NONE',  ( 91.41666666666667140, -6.884901960086287076, -3.975000000000000977 ) ) ;
#53446=CARTESIAN_POINT ( 'NONE',  ( 123.7245968585647660, -1.637169565754160949, 6.109999999999997655 ) ) ;
#53476=CIRCLE ( 'NONE', #37227, 4.749999999999997335 ) ;
#53486=CARTESIAN_POINT ( 'NONE',  ( 30.04209685856476497, 5.291415217122923842, -3.054999999999996163 ) ) ;
#53508=CARTESIAN_POINT ( 'NONE',  ( 111.9333603837962272, 2.130196079827431532, -7.949999999999997513 ) ) ;
#53535=CYLINDRICAL_SURFACE ( 'NONE', #121165, 7.950000000000000178 ) ;
#53548=CARTESIAN_POINT ( 'NONE',  ( 92.45876352523144703, 0.000000000000000000, -6.110000000000001208 ) ) ;
#53560=CARTESIAN_POINT ( 'NONE',  ( 93.39126352523143737, -4.472830434245839371, -4.472830434245839371 ) ) ;
#53649=CARTESIAN_POINT ( 'NONE',  ( 90.76626352523146579, 4.472830434245839371, -4.472830434245839371 ) ) ;
#53651=CARTESIAN_POINT ( 'NONE',  ( 7.437137942570125837, -8.911461087268691017, 3.298467410628505014 ) ) ;
#53682=VERTEX_POINT ( 'NONE', #5735 ) ;
#53709=CARTESIAN_POINT ( 'NONE',  ( 98.85416666666664298, -2.130196079827425315, -7.950000000000001066 ) ) ;
#53731=CARTESIAN_POINT ( 'NONE',  ( 31.72502705046288796, 5.819803920172573086, -5.819803920172572198 ) ) ;
#53736=CARTESIAN_POINT ( 'NONE',  ( 29.72916666666665009, 7.950000000000001954, -2.130196079827421762 ) ) ;
#53747=CARTESIAN_POINT ( 'NONE',  ( 126.9329301918981088, 1.637169565754156508, 6.110000000000000320 ) ) ;
#53757=CARTESIAN_POINT ( 'NONE',  ( 49.29209685856476852, -5.291415217122921177, 3.054999999999999272 ) ) ;
#53765=CARTESIAN_POINT ( 'NONE',  ( 35.05793019189811588, 6.110000000000000320, -1.637169565754156064 ) ) ;
#53775=CARTESIAN_POINT ( 'NONE',  ( 79.12086038379622721, -6.884901960086286188, 3.974999999999997424 ) ) ;
#53797=CARTESIAN_POINT ( 'NONE',  ( 58.68293019189811588, -1.637169565754158951, -6.109999999999998543 ) ) ;
#53832=CARTESIAN_POINT ( 'NONE',  ( 119.9329301918981230, 1.637169565754156730, 6.110000000000001208 ) ) ;
#53849=DIRECTION ( 'NONE',  ( -1.000000000000000000, -0.000000000000000000, -0.000000000000000000 ) ) ;
#53879=CARTESIAN_POINT ( 'NONE',  ( 37.82876352523144448, 0.000000000000000000, -6.109999999999999432 ) ) ;
#53909=CARTESIAN_POINT ( 'NONE',  ( 55.93336038379622011, 2.130196079827431532, -7.949999999999997513 ) ) ;
#53915=CARTESIAN_POINT ( 'NONE',  ( 59.18749999999997868, -5.819803920172573086, 5.819803920172572198 ) ) ;
#53923=CARTESIAN_POINT ( 'NONE',  ( 48.70876352523144703, -7.482591942790329030E-16, 6.110000000000001208 ) ) ;
#53938=CARTESIAN_POINT ( 'NONE',  ( 84.00043019189810423, -3.055000000000002380, 5.291415217122920289 ) ) ;
#53947=CARTESIAN_POINT ( 'NONE',  ( 63.49543019189811588, 5.291415217122916737, 3.055000000000001936 ) ) ;
#53954=DIRECTION ( 'NONE',  ( -1.000000000000000000, -0.000000000000000000, -0.000000000000000000 ) ) ;
#53976=CARTESIAN_POINT ( 'NONE',  ( 85.37043019189812298, -3.055000000000001492, 5.291415217122917625 ) ) ;
#54004=CARTESIAN_POINT ( 'NONE',  ( 33.97959685856477563, 6.109999999999999432, 1.637169565754164280 ) ) ;
#54029=ORIENTED_EDGE ( 'NONE', *, *, #118122, .F. ) ;
#54044=CARTESIAN_POINT ( 'NONE',  ( 97.78752705046289861, 0.000000000000000000, -7.949999999999998401 ) ) ;
#54064=CARTESIAN_POINT ( 'NONE',  ( 69.91209685856478018, 5.291415217122922066, -3.054999999999995275 ) ) ;
#54068=CARTESIAN_POINT ( 'NONE',  ( 84.85416666666667140, -2.130196079827463507, -7.949999999999979750 ) ) ;
#54079=CARTESIAN_POINT ( 'NONE',  ( 107.6041666666666714, 2.130196079827441746, 7.949999999999992184 ) ) ;
#54091=CARTESIAN_POINT ( 'NONE',  ( 84.37086038379624142, 6.884901960086289741, -3.974999999999993427 ) ) ;
#54097=CARTESIAN_POINT ( 'NONE',  ( 87.33333333333332860, -6.884901960086287964, 3.974999999999998312 ) ) ;
#54106=CARTESIAN_POINT ( 'NONE',  ( 71.75043019189811844, 3.055000000000002824, -5.291415217122919401 ) ) ;
#54124=CARTESIAN_POINT ( 'NONE',  ( 60.66709685856477563, -3.055000000000000160, -5.291415217122921177 ) ) ;
#54149=CARTESIAN_POINT ( 'NONE',  ( 61.22916666666666430, 7.950000000000001954, -2.130196079827421762 ) ) ;
#54159=CARTESIAN_POINT ( 'NONE',  ( 111.0370968585647944, -3.054999999999998828, -5.291415217122919401 ) ) ;
#54183=CARTESIAN_POINT ( 'NONE',  ( 63.29209685856476852, -5.291415217122921177, 3.054999999999999272 ) ) ;
#54189=CARTESIAN_POINT ( 'NONE',  ( 103.3962635252314470, 4.472830434245840259, -4.472830434245838482 ) ) ;
#54207=CARTESIAN_POINT ( 'NONE',  ( 124.0162635252314516, -4.472830434245838482, 4.472830434245838482 ) ) ;
#54212=ORIENTED_EDGE ( 'NONE', *, *, #73856, .T. ) ;
#54221=CARTESIAN_POINT ( 'NONE',  ( 11.47472276569333083, -8.505968740979792386, -4.231148911907932408 ) ) ;
#54232=CARTESIAN_POINT ( 'NONE',  ( 29.31293019189811133, -1.637169565754159617, -6.110000000000001208 ) ) ;
#54254=CARTESIAN_POINT ( 'NONE',  ( 116.4541937171295558, 6.884901960086283523, 3.975000000000002753 ) ) ;
#54255=CARTESIAN_POINT ( 'NONE',  ( 48.78752705046289151, 0.000000000000000000, -7.949999999999998401 ) ) ;
#54290=VERTEX_POINT ( 'NONE', #141086 ) ;
#54292=CARTESIAN_POINT ( 'NONE',  ( 93.91709685856477563, 3.054999999999998828, 5.291415217122922066 ) ) ;
#54295=CARTESIAN_POINT ( 'NONE',  ( 84.95419371712955581, 6.884901960086283523, 3.975000000000002753 ) ) ;
#54298=DIRECTION ( 'NONE',  ( -0.000000000000000000, 0.000000000000000000, 1.000000000000000000 ) ) ;
#54300=CARTESIAN_POINT ( 'NONE',  ( 90.18293019189809456, -1.637169565754158951, -6.109999999999998543 ) ) ;
#54337=CARTESIAN_POINT ( 'NONE',  ( 118.9791666666666430, -7.950000000000000178, 2.130196079827424427 ) ) ;
#54368=EDGE_CURVE ( 'NONE', #127835, #139877, #56289, .T. ) ;
#54385=CARTESIAN_POINT ( 'NONE',  ( 90.32876352523145158, 0.000000000000000000, -6.109999999999999432 ) ) ;
#54391=CARTESIAN_POINT ( 'NONE',  ( 0.000000000000000000, 0.000000000000000000, 0.000000000000000000 ) ) ;
#54403=ORIENTED_EDGE ( 'NONE', *, *, #135838, .F. ) ;
#54433=CARTESIAN_POINT ( 'NONE',  ( 97.39583333333334281, -2.130196079827427091, 7.949999999999999289 ) ) ;
#54453=CARTESIAN_POINT ( 'NONE',  ( 27.35002705046288085, -5.819803920172572198, -5.819803920172572198 ) ) ;
#54459=CARTESIAN_POINT ( 'NONE',  ( 116.6670968585647756, -3.055000000000000160, -5.291415217122921177 ) ) ;
#54468=CARTESIAN_POINT ( 'NONE',  ( 122.7037635252314516, 6.109999999999998543, 1.122388791418548911E-15 ) ) ;
#54469=ORIENTED_EDGE ( 'NONE', *, *, #42566, .F. ) ;
#54474=CARTESIAN_POINT ( 'NONE',  ( 36.45876352523143282, 0.000000000000000000, -6.110000000000001208 ) ) ;
#54481=CARTESIAN_POINT ( 'NONE',  ( 42.49543019189810877, 5.291415217122916737, 3.055000000000001936 ) ) ;
#54511=CARTESIAN_POINT ( 'NONE',  ( 45.12043019189810877, 3.055000000000001936, -5.291415217122916737 ) ) ;
#54546=CARTESIAN_POINT ( 'NONE',  ( 117.7454301918981230, -5.291415217122919401, -3.055000000000000604 ) ) ;
#54549=EDGE_CURVE ( 'NONE', #7898, #4663, #131496, .T. ) ;
#54556=CARTESIAN_POINT ( 'NONE',  ( 76.20419371712955581, -6.884901960086285300, -3.975000000000000089 ) ) ;
#54582=CARTESIAN_POINT ( 'NONE',  ( 42.20376352523144448, 6.109999999999999432, 1.122388791418549108E-15 ) ) ;
#54598=CARTESIAN_POINT ( 'NONE',  ( 123.8129301918981184, -1.637169565754159617, -6.110000000000001208 ) ) ;
#54607=CARTESIAN_POINT ( 'NONE',  ( 60.89169371712955581, 2.130196079827421762, 7.950000000000001066 ) ) ;
#54613=CARTESIAN_POINT ( 'NONE',  ( 44.02083333333333570, 7.949999999999999289, 2.130196079827431532 ) ) ;
#54621=CARTESIAN_POINT ( 'NONE',  ( 49.58376352523144703, -6.110000000000001208, -3.741295971395164515E-16 ) ) ;
#54634=CARTESIAN_POINT ( 'NONE',  ( 78.60459685856477563, 1.637169565754164946, -6.109999999999999432 ) ) ;
#54645=CARTESIAN_POINT ( 'NONE',  ( 65.97459685856479439, 1.637169565754164058, -6.109999999999996767 ) ) ;
#54667=EDGE_CURVE ( 'NONE', #20647, #121702, #132952, .T. ) ;
#54669=CARTESIAN_POINT ( 'NONE',  ( 41.20419371712954870, -6.884901960086285300, -3.975000000000000089 ) ) ;
#54678=CARTESIAN_POINT ( 'NONE',  ( 77.78709685856478018, 3.054999999999997495, 5.291415217122919401 ) ) ;
#54702=CARTESIAN_POINT ( 'NONE',  ( 38.50043019189809712, -3.055000000000002380, 5.291415217122920289 ) ) ;
#54737=CARTESIAN_POINT ( 'NONE',  ( 96.32919371712955581, -3.975000000000001865, 6.884901960086284411 ) ) ;
#54754=CARTESIAN_POINT ( 'NONE',  ( 52.91666666666666430, -6.884901960086287076, -3.975000000000000977 ) ) ;
#54756=CARTESIAN_POINT ( 'NONE',  ( 69.76626352523143737, 4.472830434245839371, -4.472830434245839371 ) ) ;
#54781=CARTESIAN_POINT ( 'NONE',  ( 82.91252705046289861, -7.949999999999998401, -4.867971026610728450E-16 ) ) ;
#54786=CARTESIAN_POINT ( 'NONE',  ( 81.49999999999998579, 0.000000000000000000, -7.950000000000000178 ) ) ;
#54797=CARTESIAN_POINT ( 'NONE',  ( 76.85459685856477563, -1.637169565754161615, 6.110000000000000320 ) ) ;
#54800=DIRECTION ( 'NONE',  ( -1.000000000000000000, 0.000000000000000000, -0.000000000000000000 ) ) ;
#54814=CARTESIAN_POINT ( 'NONE',  ( 66.35459685856476142, -1.637169565754161615, 6.110000000000000320 ) ) ;
#54821=CARTESIAN_POINT ( 'NONE',  ( 125.3500270504628844, -5.819803920172573086, -5.819803920172573086 ) ) ;
#54848=EDGE_CURVE ( 'NONE', #7244, #135518, #68036, .T. ) ;
#54850=CARTESIAN_POINT ( 'NONE',  ( 116.7245968585647802, -1.637169565754160949, 6.109999999999997655 ) ) ;
#54860=CARTESIAN_POINT ( 'NONE',  ( 68.76669371712957002, -7.949999999999998401, 2.130196079827423983 ) ) ;
#54862=CARTESIAN_POINT ( 'NONE',  ( 37.74999999999999289, -9.735942053221458872E-16, 7.950000000000000178 ) ) ;
#54874=CARTESIAN_POINT ( 'NONE',  ( 67.22959685856476142, -6.110000000000000320, -1.637169565754161393 ) ) ;
#54875=AXIS2_PLACEMENT_3D ( 'NONE', #49895, #69506, #47768 ) ;
#54878=( BOUNDED_CURVE ( )  B_SPLINE_CURVE ( 2, ( #81872, #51357, #38332, #126065, #28884, #73121, #6352, #26731, #49936, #82548, #126735, #84008, #104998 ),
 .UNSPECIFIED., .F., .T. ) 
 B_SPLINE_CURVE_WITH_KNOTS ( ( 3, 2, 2, 2, 2, 2, 3 ),
 ( 0.5000000000000000000, 0.5027777777777777679, 0.5055555555555555358, 0.5083333333333333037, 0.5111111111111110716, 0.5138888888888888395, 0.5166666666666667185 ),
 .UNSPECIFIED. ) 
 CURVE ( )  GEOMETRIC_REPRESENTATION_ITEM ( )  RATIONAL_B_SPLINE_CURVE ( ( 1.000000000000000000, 0.9659258262890683122, 1.000000000000000000, 0.9659258262890683122, 1.000000000000000000, 0.9659258262890683122, 1.000000000000000000, 0.9659258262890683122, 1.000000000000000000, 0.9659258262890683122, 1.000000000000000000, 0.9659258262890683122, 1.000000000000000000 ) ) 
 REPRESENTATION_ITEM ( '' )  );
#54883=CARTESIAN_POINT ( 'NONE',  ( 100.6254301918981042, 5.291415217122919401, 3.055000000000002824 ) ) ;
#54890=CARTESIAN_POINT ( 'NONE',  ( 92.00000000000000000, 0.000000000000000000, -7.950000000000000178 ) ) ;
#54896=ORIENTED_EDGE ( 'NONE', *, *, #56539, .F. ) ;
#54897=CARTESIAN_POINT ( 'NONE',  ( 126.0579301918981230, 6.110000000000000320, -1.637169565754156064 ) ) ;
#54922=CARTESIAN_POINT ( 'NONE',  ( 30.33376352523143993, 6.110000000000001208, 1.122388791418549305E-15 ) ) ;
#54928=CARTESIAN_POINT ( 'NONE',  ( 128.8886022459138019, 0.000000000000000000, -6.349999999999997868 ) ) ;
#54948=CARTESIAN_POINT ( 'NONE',  ( 114.8500270504628844, -5.819803920172572198, -5.819803920172572198 ) ) ;
#54980=CARTESIAN_POINT ( 'NONE',  ( 70.70833333333332860, -3.974999999999999201, -6.884901960086287964 ) ) ;
#54987=CARTESIAN_POINT ( 'NONE',  ( 94.93793019189810423, -6.110000000000001208, 1.637169565754158951 ) ) ;
#54990=EDGE_CURVE ( 'NONE', #34604, #120211, #7830, .T. ) ;
#54996=PLANE ( 'NONE',  #28097 ) ;
#54999=CARTESIAN_POINT ( 'NONE',  ( 82.45376352523145158, -6.109999999999998543, -3.741295971395162543E-16 ) ) ;
#55038=CARTESIAN_POINT ( 'NONE',  ( 116.0166937171295700, 7.950000000000000178, -2.130196079827421318 ) ) ;
#55078=CARTESIAN_POINT ( 'NONE',  ( 81.87043019189812298, -3.055000000000001936, 5.291415217122918513 ) ) ;
#55081=ORIENTED_EDGE ( 'NONE', *, *, #127793, .F. ) ;
#55111=EDGE_CURVE ( 'NONE', #125681, #135809, #100822, .T. ) ;
#55126=CARTESIAN_POINT ( 'NONE',  ( 104.2500000000000000, -9.735942053221458872E-16, 7.950000000000000178 ) ) ;
#55154=CARTESIAN_POINT ( 'NONE',  ( 123.6670968585647756, -3.055000000000000160, -5.291415217122921177 ) ) ;
#55163=CARTESIAN_POINT ( 'NONE',  ( 111.9120968585647944, 5.291415217122921177, -3.054999999999994831 ) ) ;
#55171=ADVANCED_FACE ( 'NONE', ( #28268 ), #28977, .T. ) ;
#55174=CARTESIAN_POINT ( 'NONE',  ( 39.66709685856477563, -3.055000000000000160, -5.291415217122921177 ) ) ;
#55181=CARTESIAN_POINT ( 'NONE',  ( 29.80793019189811588, -6.109999999999998543, 1.637169565754158063 ) ) ;
#55208=CARTESIAN_POINT ( 'NONE',  ( 43.66209685856478728, -5.291415217122919401, 3.054999999999997939 ) ) ;
#55246=CARTESIAN_POINT ( 'NONE',  ( 111.3287635252314516, 0.000000000000000000, -6.109999999999999432 ) ) ;
#55294=CARTESIAN_POINT ( 'NONE',  ( 27.47459685856478018, 1.637169565754164280, -6.109999999999997655 ) ) ;
#55311=CARTESIAN_POINT ( 'NONE',  ( 125.5629301918981042, 1.637169565754157174, 6.110000000000002984 ) ) ;
#55320=CARTESIAN_POINT ( 'NONE',  ( 59.72502705046289861, 5.819803920172573086, -5.819803920172572198 ) ) ;
#55325=CARTESIAN_POINT ( 'NONE',  ( 45.18749999999998579, -5.819803920172573086, 5.819803920172572198 ) ) ;
#55332=CARTESIAN_POINT ( 'NONE',  ( 36.16709685856476852, -3.055000000000000160, -5.291415217122921177 ) ) ;
#55343=DIRECTION ( 'NONE',  ( -1.000000000000000000, -0.000000000000000000, -0.000000000000000000 ) ) ;
#55350=CARTESIAN_POINT ( 'NONE',  ( 86.04209685856477563, 5.291415217122923842, -3.054999999999996163 ) ) ;
#55354=DIRECTION ( 'NONE',  ( -1.000000000000000000, -0.000000000000000000, -0.000000000000000000 ) ) ;
#55359=CARTESIAN_POINT ( 'NONE',  ( 65.68293019189810877, -1.637169565754158951, -6.109999999999998543 ) ) ;
#55390=CARTESIAN_POINT ( 'NONE',  ( 76.32876352523145158, 0.000000000000000000, -6.109999999999998543 ) ) ;
#55412=CARTESIAN_POINT ( 'NONE',  ( 27.85459685856476852, -1.637169565754161615, 6.110000000000000320 ) ) ;
#55466=CARTESIAN_POINT ( 'NONE',  ( 67.43293019189812298, 1.637169565754156730, 6.110000000000001208 ) ) ;
#55469=CARTESIAN_POINT ( 'NONE',  ( 118.2500000000000000, -9.735942053221458872E-16, 7.950000000000000178 ) ) ;
#55470=CARTESIAN_POINT ( 'NONE',  ( 32.74586038379622011, 3.974999999999996980, 6.884901960086287964 ) ) ;
#55490=CARTESIAN_POINT ( 'NONE',  ( 26.65943557924714113, -6.350000000000002309, -1.701477371937631045 ) ) ;
#55495=CARTESIAN_POINT ( 'NONE',  ( 81.60002705046289861, 5.819803920172570422, 5.819803920172574863 ) ) ;
#55499=CARTESIAN_POINT ( 'NONE',  ( 75.22916666666665719, 7.950000000000001954, -2.130196079827421762 ) ) ;
#55509=CARTESIAN_POINT ( 'NONE',  ( 70.14626352523143282, -4.472830434245840259, 4.472830434245839371 ) ) ;
#55516=DIRECTION ( 'NONE',  ( 0.000000000000000000, 0.000000000000000000, 1.000000000000000000 ) ) ;
#55526=CARTESIAN_POINT ( 'NONE',  ( 59.93793019189809712, -6.110000000000001208, 1.637169565754158951 ) ) ;
#55540=CARTESIAN_POINT ( 'NONE',  ( 111.9333603837962272, 2.130196079827431532, -7.949999999999996625 ) ) ;
#55545=( BOUNDED_CURVE ( )  B_SPLINE_CURVE ( 2, ( #20306, #129082, #32651, #75438, #97133, #18894, #141392, #10848, #139996, #31223, #131967, #107332, #76889 ),
 .UNSPECIFIED., .F., .T. ) 
 B_SPLINE_CURVE_WITH_KNOTS ( ( 3, 2, 2, 2, 2, 2, 3 ),
 ( 0.9000000000000001332, 0.9027777777777779011, 0.9055555555555556690, 0.9083333333333334370, 0.9111111111111110938, 0.9138888888888888618, 0.9166666666666666297 ),
 .UNSPECIFIED. ) 
 CURVE ( )  GEOMETRIC_REPRESENTATION_ITEM ( )  RATIONAL_B_SPLINE_CURVE ( ( 0.9999999999999986677, 0.9659258262890696445, 1.000000000000000000, 0.9659258262890683122, 1.000000000000000000, 0.9659258262890683122, 1.000000000000000000, 0.9659258262890683122, 1.000000000000000000, 0.9659258262890683122, 1.000000000000000000, 0.9659258262890683122, 1.000000000000000000 ) ) 
 REPRESENTATION_ITEM ( '' )  );
#55548=EDGE_CURVE ( 'NONE', #96695, #19121, #7169, .T. ) ;
#55551=CARTESIAN_POINT ( 'NONE',  ( 127.7219355792471305, -5.499261314031185677, 3.174999999999998046 ) ) ;
#55552=CARTESIAN_POINT ( 'NONE',  ( 61.37500000000000000, 7.950000000000000178, 1.460391307983218535E-15 ) ) ;
#55557=VERTEX_POINT ( 'NONE', #117051 ) ;
#55560=CARTESIAN_POINT ( 'NONE',  ( 100.5370968585647802, -3.054999999999998828, -5.291415217122919401 ) ) ;
#55580=CARTESIAN_POINT ( 'NONE',  ( 86.89583333333335702, -2.130196079827389344, 7.950000000000021494 ) ) ;
#55589=CARTESIAN_POINT ( 'NONE',  ( 58.33376352523143993, 6.110000000000001208, 1.122388791418549305E-15 ) ) ;
#55595=CARTESIAN_POINT ( 'NONE',  ( 91.72959685856477563, -6.110000000000000320, -1.637169565754161393 ) ) ;
#55609=CARTESIAN_POINT ( 'NONE',  ( 124.3079301918981230, -6.109999999999998543, 1.637169565754158507 ) ) ;
#55645=CARTESIAN_POINT ( 'NONE',  ( 42.41666666666665719, -6.884901960086287076, -3.975000000000000977 ) ) ;
#55658=CARTESIAN_POINT ( 'NONE',  ( 112.3708603837962272, 6.884901960086289741, -3.974999999999993427 ) ) ;
#55676=CARTESIAN_POINT ( 'NONE',  ( 105.1462635252314612, -4.472830434245840259, 4.472830434245839371 ) ) ;
#55703=CARTESIAN_POINT ( 'NONE',  ( 90.27126352523143282, 4.472830434245839371, 4.472830434245842035 ) ) ;
#55712=CARTESIAN_POINT ( 'NONE',  ( 49.85416666666665719, -2.130196079827501698, -7.949999999999956657 ) ) ;
#55713=CARTESIAN_POINT ( 'NONE',  ( 84.49543019189812298, 5.291415217122916737, 3.055000000000001936 ) ) ;
#55740=CARTESIAN_POINT ( 'NONE',  ( 57.24586038379622721, 3.974999999999996980, 6.884901960086287964 ) ) ;
#55802=CARTESIAN_POINT ( 'NONE',  ( 79.68293019189812298, -1.637169565754159173, -6.109999999999999432 ) ) ;
#55843=DIRECTION ( 'NONE',  ( -1.000000000000000000, -0.000000000000000000, -0.000000000000000000 ) ) ;
#55854=CARTESIAN_POINT ( 'NONE',  ( 102.3541666666666714, -2.130196079827425315, -7.950000000000001066 ) ) ;
#55878=CARTESIAN_POINT ( 'NONE',  ( 85.97502705046289861, -5.819803920172573086, 5.819803920172573086 ) ) ;
#55884=CARTESIAN_POINT ( 'NONE',  ( 120.6045968585647614, 1.637169565754164946, -6.109999999999999432 ) ) ;
#55893=CARTESIAN_POINT ( 'NONE',  ( 110.1620968585647944, -5.291415217122919401, 3.054999999999997939 ) ) ;
#55896=ORIENTED_EDGE ( 'NONE', *, *, #39376, .F. ) ;
#55901=CARTESIAN_POINT ( 'NONE',  ( 36.75043019189811133, 3.055000000000002824, -5.291415217122919401 ) ) ;
#55907=CARTESIAN_POINT ( 'NONE',  ( 33.89126352523143737, -4.472830434245839371, -4.472830434245839371 ) ) ;
#55939=CARTESIAN_POINT ( 'NONE',  ( 50.22459685856478018, -1.637169565754160949, 6.109999999999997655 ) ) ;
#55967=CARTESIAN_POINT ( 'NONE',  ( 36.53752705046288440, -9.735942053221456900E-16, 7.949999999999998401 ) ) ;
#55968=VERTEX_POINT ( 'NONE', #93718 ) ;
#55982=CARTESIAN_POINT ( 'NONE',  ( 115.2662635252314374, 4.472830434245839371, -4.472830434245839371 ) ) ;
#56026=CARTESIAN_POINT ( 'NONE',  ( 126.9294095003570817, -4.539267423379012456, -4.720787893125737433 ) ) ;
#56027=CARTESIAN_POINT ( 'NONE',  ( 127.5375270504628986, -9.735942053221456900E-16, 7.949999999999998401 ) ) ;
#56032=CARTESIAN_POINT ( 'NONE',  ( 126.5624999999999858, -5.819803920172572198, -5.819803920172573086 ) ) ;
#56045=CARTESIAN_POINT ( 'NONE',  ( 124.2504301918981184, 3.055000000000002824, -5.291415217122919401 ) ) ;
#56047=ADVANCED_FACE ( 'NONE', ( #71268 ), #118299, .T. ) ;
#56056=CARTESIAN_POINT ( 'NONE',  ( 46.01669371712956291, 7.950000000000001066, -2.130196079827421318 ) ) ;
#56061=CARTESIAN_POINT ( 'NONE',  ( 47.37500000000000000, 7.950000000000000178, 1.460391307983218535E-15 ) ) ;
#56073=CARTESIAN_POINT ( 'NONE',  ( 42.29209685856477563, -5.291415217122921177, 3.054999999999999272 ) ) ;
#56082=DIRECTION ( 'NONE',  ( 0.000000000000000000, 0.000000000000000000, 1.000000000000000000 ) ) ;
#56096=CARTESIAN_POINT ( 'NONE',  ( 56.64126352523144448, 4.472830434245836706, 4.472830434245840259 ) ) ;
#56127=CARTESIAN_POINT ( 'NONE',  ( 76.62043019189812298, 3.055000000000001936, -5.291415217122916737 ) ) ;
#56128=ORIENTED_EDGE ( 'NONE', *, *, #85740, .F. ) ;
#56139=DIRECTION ( 'NONE',  ( -1.000000000000000000, -0.000000000000000000, -0.000000000000000000 ) ) ;
#56156=CARTESIAN_POINT ( 'NONE',  ( 25.66709685856477563, -3.055000000000000160, -5.291415217122921177 ) ) ;
#56213=CARTESIAN_POINT ( 'NONE',  ( 55.03709685856478018, -3.054999999999999272, -5.291415217122919401 ) ) ;
#56217=CARTESIAN_POINT ( 'NONE',  ( 84.27083333333332860, -7.949999999999998401, -2.130196079827426203 ) ) ;
#56240=CARTESIAN_POINT ( 'NONE',  ( 75.32919371712957002, -3.975000000000001865, 6.884901960086284411 ) ) ;
#56245=CARTESIAN_POINT ( 'NONE',  ( 75.95833333333332860, 3.974999999999997424, 6.884901960086288852 ) ) ;
#56251=ORIENTED_EDGE ( 'NONE', *, *, #1920, .F. ) ;
#56257=CARTESIAN_POINT ( 'NONE',  ( 67.37543019189810423, -5.291415217122920289, -3.055000000000001492 ) ) ;
#56275=CARTESIAN_POINT ( 'NONE',  ( 66.93793019189809002, -6.110000000000001208, 1.637169565754158951 ) ) ;
#56289=LINE ( 'NONE', #100470, #46813 ) ;
#56306=CARTESIAN_POINT ( 'NONE',  ( 101.4120968585647802, 5.291415217122921177, -3.054999999999994831 ) ) ;
#56332=ORIENTED_EDGE ( 'NONE', *, *, #44687, .T. ) ;
#56335=CARTESIAN_POINT ( 'NONE',  ( 51.62543019189811133, 5.291415217122919401, 3.055000000000002824 ) ) ;
#56342=CARTESIAN_POINT ( 'NONE',  ( 94.79209685856476142, -5.291415217122921177, 3.054999999999999272 ) ) ;
#56407=CARTESIAN_POINT ( 'NONE',  ( 111.4958603837962272, -3.974999999999998312, -6.884901960086286188 ) ) ;
#56426=CARTESIAN_POINT ( 'NONE',  ( 93.77126352523141861, 4.472830434245839371, 4.472830434245842035 ) ) ;
#56434=( BOUNDED_CURVE ( )  B_SPLINE_CURVE ( 2, ( #51071, #84430, #62662, #106852, #53187, #97387, #42349, #143062, #65548, #101693, #88706, #22670, #134346 ),
 .UNSPECIFIED., .F., .T. ) 
 B_SPLINE_CURVE_WITH_KNOTS ( ( 3, 2, 2, 2, 2, 2, 3 ),
 ( 0.3833333333333333592, 0.3861111111111111271, 0.3888888888888888951, 0.3916666666666666630, 0.3944444444444444309, 0.3972222222222221988, 0.4000000000000000222 ),
 .UNSPECIFIED. ) 
 CURVE ( )  GEOMETRIC_REPRESENTATION_ITEM ( )  RATIONAL_B_SPLINE_CURVE ( ( 1.000000000000000000, 0.9659258262890683122, 1.000000000000000000, 0.9659258262890683122, 1.000000000000000000, 0.9659258262890683122, 1.000000000000000000, 0.9659258262890683122, 1.000000000000000000, 0.9659258262890683122, 1.000000000000000000, 0.9659258262890683122, 1.000000000000000000 ) ) 
 REPRESENTATION_ITEM ( '' )  );
#56445=DIRECTION ( 'NONE',  ( -1.000000000000000000, -0.000000000000000000, -0.000000000000000000 ) ) ;
#56448=VECTOR ( 'NONE', #119888, 1000.000000000000000 ) ;
#56452=CARTESIAN_POINT ( 'NONE',  ( 88.08376352523144703, -6.110000000000001208, -3.741295971395164515E-16 ) ) ;
#56464=CARTESIAN_POINT ( 'NONE',  ( 99.00000000000000000, 0.000000000000000000, -7.950000000000000178 ) ) ;
#56465=CARTESIAN_POINT ( 'NONE',  ( 85.51626352523145158, -4.472830434245839371, 4.472830434245839371 ) ) ;
#56515=CARTESIAN_POINT ( 'NONE',  ( 116.2295968585647756, -6.110000000000000320, -1.637169565754161393 ) ) ;
#56539=EDGE_CURVE ( 'NONE', #69571, #29421, #65945, .T. ) ;
#56549=CARTESIAN_POINT ( 'NONE',  ( 82.89126352523142316, -4.472830434245839371, -4.472830434245839371 ) ) ;
#56598=CARTESIAN_POINT ( 'NONE',  ( 101.3333333333333286, -6.884901960086287964, 3.974999999999998312 ) ) ;
#56620=CARTESIAN_POINT ( 'NONE',  ( 86.12086038379622721, -6.884901960086286188, 3.974999999999997424 ) ) ;
#56625=CARTESIAN_POINT ( 'NONE',  ( 122.0629301918981042, 1.637169565754157174, 6.110000000000002984 ) ) ;
#56634=CARTESIAN_POINT ( 'NONE',  ( 111.1829301918981230, -1.637169565754158951, -6.109999999999998543 ) ) ;
#56637=ORIENTED_EDGE ( 'NONE', *, *, #139767, .T. ) ;
#56642=CARTESIAN_POINT ( 'NONE',  ( 37.33376352523143282, 6.110000000000001208, 1.122388791418549305E-15 ) ) ;
#56649=CARTESIAN_POINT ( 'NONE',  ( 26.74543019189810877, -5.291415217122918513, -3.055000000000000160 ) ) ;
#56671=CARTESIAN_POINT ( 'NONE',  ( 0.000000000000000000, 0.000000000000000000, 7.950000000000000178 ) ) ;
#56679=CARTESIAN_POINT ( 'NONE',  ( 42.78709685856478728, 3.054999999999997495, 5.291415217122919401 ) ) ;
#56687=CARTESIAN_POINT ( 'NONE',  ( 160.0000000000000000, 7.776507174585690191E-16, -6.349999999999997868 ) ) ;
#56698=CARTESIAN_POINT ( 'NONE',  ( 35.95419371712956291, 6.884901960086283523, 3.975000000000002753 ) ) ;
#56713=CARTESIAN_POINT ( 'NONE',  ( 108.8495968585647660, 6.109999999999997655, 1.637169565754163836 ) ) ;
#56726=CARTESIAN_POINT ( 'NONE',  ( 121.3124999999999858, 5.819803920172571310, 5.819803920172576639 ) ) ;
#56749=AXIS2_PLACEMENT_3D ( 'NONE', #54391, #87696, #142792 ) ;
#56755=CARTESIAN_POINT ( 'NONE',  ( 128.5583603837962130, -7.949999999999997513, -2.130196079827425759 ) ) ;
#56772=CARTESIAN_POINT ( 'NONE',  ( 118.8545968585647898, -1.637169565754161615, 6.110000000000000320 ) ) ;
#56777=CARTESIAN_POINT ( 'NONE',  ( 78.43750000000000000, 5.819803920172574863, -5.819803920172573086 ) ) ;
#56783=CARTESIAN_POINT ( 'NONE',  ( 51.85002705046287730, -5.819803920172572198, -5.819803920172572198 ) ) ;
#56789=CARTESIAN_POINT ( 'NONE',  ( 47.66666666666666430, 6.884901960086285300, 3.975000000000003642 ) ) ;
#56796=CARTESIAN_POINT ( 'NONE',  ( 35.43793019189810423, -6.110000000000001208, 1.637169565754158951 ) ) ;
#56809=LINE ( 'NONE', #67681, #62412 ) ;
#56817=CARTESIAN_POINT ( 'NONE',  ( 56.93293019189810877, 1.637169565754156508, 6.110000000000000320 ) ) ;
#56849=CARTESIAN_POINT ( 'NONE',  ( 78.37043019189812298, -3.055000000000001492, 5.291415217122917625 ) ) ;
#56858=CARTESIAN_POINT ( 'NONE',  ( 122.9166666666666714, -6.884901960086287076, -3.975000000000000977 ) ) ;
#56870=ORIENTED_EDGE ( 'NONE', *, *, #125828, .F. ) ;
#56872=CARTESIAN_POINT ( 'NONE',  ( 26.83376352523143993, 6.110000000000001208, 1.122388791418549305E-15 ) ) ;
#56876=CARTESIAN_POINT ( 'NONE',  ( 89.91252705046289861, -7.949999999999998401, -4.867971026610728450E-16 ) ) ;
#56909=CARTESIAN_POINT ( 'NONE',  ( 111.8333333333333428, -6.884901960086287964, 3.974999999999998312 ) ) ;
#56912=CARTESIAN_POINT ( 'NONE',  ( 54.45376352523144448, -6.109999999999999432, -3.741295971395163529E-16 ) ) ;
#56936=CARTESIAN_POINT ( 'NONE',  ( 77.37086038379622721, 6.884901960086289741, -3.974999999999993427 ) ) ;
#56942=CARTESIAN_POINT ( 'NONE',  ( 70.56250000000001421, -5.819803920172572198, -5.819803920172573086 ) ) ;
#56953=CARTESIAN_POINT ( 'NONE',  ( 61.68793019189811844, 6.110000000000002984, -1.637169565754156730 ) ) ;
#56971=CARTESIAN_POINT ( 'NONE',  ( 58.91709685856477563, 3.054999999999998828, 5.291415217122922066 ) ) ;
#56976=ADVANCED_FACE ( 'NONE', ( #128006 ), #31353, .T. ) ;
#56986=ADVANCED_FACE ( 'NONE', ( #138152 ), #117082, .T. ) ;
#56995=CARTESIAN_POINT ( 'NONE',  ( 37.26669371712955581, -7.949999999999998401, 2.130196079827423983 ) ) ;
#57003=CARTESIAN_POINT ( 'NONE',  ( 107.6829301918981088, -1.637169565754158951, -6.109999999999998543 ) ) ;
#57019=CARTESIAN_POINT ( 'NONE',  ( 69.10416666666665719, 2.130196079827422206, 7.950000000000001954 ) ) ;
#57024=CARTESIAN_POINT ( 'NONE',  ( 87.04166666666665719, -3.975000000000002753, 6.884901960086286188 ) ) ;
#57031=CARTESIAN_POINT ( 'NONE',  ( 50.75043019189810423, 3.055000000000002824, -5.291415217122919401 ) ) ;
#57037=CARTESIAN_POINT ( 'NONE',  ( 88.81293019189809002, -1.637169565754159617, -6.110000000000001208 ) ) ;
#57073=CARTESIAN_POINT ( 'NONE',  ( 57.87499999999999289, 7.950000000000000178, 1.460391307983218535E-15 ) ) ;
#57077=CARTESIAN_POINT ( 'NONE',  ( 9.743626569336168330, 8.447988834747505393, 4.345749975250972064 ) ) ;
#57101=CARTESIAN_POINT ( 'NONE',  ( 98.95419371712955581, 6.884901960086283523, 3.975000000000002753 ) ) ;
#57123=CARTESIAN_POINT ( 'NONE',  ( 92.45876352523144703, 0.000000000000000000, -6.110000000000001208 ) ) ;
#57151=CARTESIAN_POINT ( 'NONE',  ( 84.00043019189810423, -3.055000000000002380, 5.291415217122920289 ) ) ;
#57163=CARTESIAN_POINT ( 'NONE',  ( 90.03709685856478018, -3.054999999999998828, -5.291415217122919401 ) ) ;
#57188=DIRECTION ( 'NONE',  ( 0.000000000000000000, 0.000000000000000000, 1.000000000000000000 ) ) ;
#57191=DIRECTION ( 'NONE',  ( -1.000000000000000000, -0.000000000000000000, -0.000000000000000000 ) ) ;
#57210=CARTESIAN_POINT ( 'NONE',  ( 113.7504301918981042, 3.055000000000002824, -5.291415217122919401 ) ) ;
#57240=CARTESIAN_POINT ( 'NONE',  ( 80.26626352523145158, 4.472830434245839371, -4.472830434245839371 ) ) ;
#57291=CARTESIAN_POINT ( 'NONE',  ( 91.41666666666667140, -6.884901960086287076, -3.975000000000000977 ) ) ;
#57297=CARTESIAN_POINT ( 'NONE',  ( 88.64583333333334281, 2.130196079827394229, -7.950000000000021494 ) ) ;
#57298=CARTESIAN_POINT ( 'NONE',  ( 10.90756199573120000, 8.448038036319919897, -4.345660073319586481 ) ) ;
#57306=CARTESIAN_POINT ( 'NONE',  ( 128.3912635252314374, -4.472830434245838482, -4.472830434245838482 ) ) ;
#57317=CARTESIAN_POINT ( 'NONE',  ( 121.9170968585647756, 3.054999999999998828, 5.291415217122922066 ) ) ;
#57324=CARTESIAN_POINT ( 'NONE',  ( 111.7662635252314516, 4.472830434245839371, -4.472830434245838482 ) ) ;
#57369=CARTESIAN_POINT ( 'NONE',  ( 45.99543019189810877, 5.291415217122916737, 3.055000000000001936 ) ) ;
#57378=EDGE_CURVE ( 'NONE', #942, #90062, #52304, .T. ) ;
#57398=CARTESIAN_POINT ( 'NONE',  ( 114.6829301918980946, -1.637169565754159173, -6.109999999999999432 ) ) ;
#57412=FACE_OUTER_BOUND ( 'NONE', #106712, .T. ) ;
#57437=ORIENTED_EDGE ( 'NONE', *, *, #74104, .F. ) ;
#57448=ORIENTED_EDGE ( 'NONE', *, *, #13248, .F. ) ;
#57456=ORIENTED_EDGE ( 'NONE', *, *, #18148, .T. ) ;
#57463=CARTESIAN_POINT ( 'NONE',  ( 123.3754301918981184, -5.291415217122920289, -3.055000000000001492 ) ) ;
#57467=CARTESIAN_POINT ( 'NONE',  ( 105.0791937171295700, 3.975000000000002753, -6.884901960086283523 ) ) ;
#57474=CARTESIAN_POINT ( 'NONE',  ( 43.97502705046288440, -5.819803920172572198, 5.819803920172572198 ) ) ;
#57479=CARTESIAN_POINT ( 'NONE',  ( 48.39583333333332860, -2.130196079827427091, 7.949999999999999289 ) ) ;
#57489=CARTESIAN_POINT ( 'NONE',  ( 37.04209685856476852, 5.291415217122923842, -3.054999999999996163 ) ) ;
#57510=CARTESIAN_POINT ( 'NONE',  ( 56.34959685856478018, 6.109999999999996767, 1.637169565754163836 ) ) ;
#57541=CARTESIAN_POINT ( 'NONE',  ( 79.68293019189812298, -1.637169565754158951, -6.109999999999998543 ) ) ;
#57567=CARTESIAN_POINT ( 'NONE',  ( 30.18793019189809357, 6.110000000000002984, -1.637169565754156730 ) ) ;
#57569=CARTESIAN_POINT ( 'NONE',  ( 45.04166666666665719, -3.975000000000002753, 6.884901960086286188 ) ) ;
#57577=CARTESIAN_POINT ( 'NONE',  ( 120.1000270504628986, 5.819803920172570422, 5.819803920172575751 ) ) ;
#57579=AXIS2_PLACEMENT_3D ( 'NONE', #127848, #82910, #106037 ) ;
#57616=CARTESIAN_POINT ( 'NONE',  ( 59.26626352523145869, 4.472830434245839371, -4.472830434245839371 ) ) ;
#57635=CYLINDRICAL_SURFACE ( 'NONE', #129791, 7.950000000000000178 ) ;
#57640=CARTESIAN_POINT ( 'NONE',  ( 0.000000000000000000, 0.000000000000000000, 0.000000000000000000 ) ) ;
#57646=CARTESIAN_POINT ( 'NONE',  ( 70.80836038379624142, 7.949999999999997513, 2.130196079827431088 ) ) ;
#57650=CARTESIAN_POINT ( 'NONE',  ( 74.20833333333331439, -3.974999999999999201, -6.884901960086287964 ) ) ;
#57663=CARTESIAN_POINT ( 'NONE',  ( 69.27126352523144703, 4.472830434245839371, 4.472830434245842035 ) ) ;
#57685=CARTESIAN_POINT ( 'NONE',  ( 59.06293019189809712, 1.637169565754157174, 6.110000000000002984 ) ) ;
#57686=EDGE_CURVE ( 'NONE', #25494, #135001, #132136, .T. ) ;
#57699=CARTESIAN_POINT ( 'NONE',  ( 113.3916937171295700, 2.130196079827421762, 7.950000000000000178 ) ) ;
#57711=CARTESIAN_POINT ( 'NONE',  ( 99.95376352523145158, -6.109999999999998543, -3.741295971395162543E-16 ) ) ;
#57722=CARTESIAN_POINT ( 'NONE',  ( 67.64583333333331439, 2.130196079827431976, -7.949999999999998401 ) ) ;
#57723=CARTESIAN_POINT ( 'NONE',  ( 27.10359120979227399, -7.619655331802865028, -2.702369829154340319 ) ) ;
#57737=CARTESIAN_POINT ( 'NONE',  ( 52.64626352523143282, -4.472830434245840259, 4.472830434245838482 ) ) ;
#57743=CARTESIAN_POINT ( 'NONE',  ( 89.10459685856478984, 1.637169565754164946, -6.109999999999999432 ) ) ;
#57787=UNCERTAINTY_MEASURE_WITH_UNIT (LENGTH_MEASURE( 1.000000000000000082E-05 ), #133637, 'distance_accuracy_value', 'NONE');
#57790=CARTESIAN_POINT ( 'NONE',  ( 6.178324517025699514, 9.396498330079532835, -1.424408727490640070 ) ) ;
#57806=DIRECTION ( 'NONE',  ( -1.000000000000000000, -0.000000000000000000, -0.000000000000000000 ) ) ;
#57815=CARTESIAN_POINT ( 'NONE',  ( 103.7666937171295416, -7.949999999999999289, 2.130196079827424427 ) ) ;
#57829=CARTESIAN_POINT ( 'NONE',  ( 94.64626352523143282, -4.472830434245840259, 4.472830434245839371 ) ) ;
#57858=CARTESIAN_POINT ( 'NONE',  ( 79.18793019189810423, 6.110000000000002984, -1.637169565754156730 ) ) ;
#57867=CARTESIAN_POINT ( 'NONE',  ( 103.3750000000000000, 7.950000000000000178, 1.460391307983218535E-15 ) ) ;
#57871=CARTESIAN_POINT ( 'NONE',  ( 76.18293019189810877, -1.637169565754158951, -6.109999999999998543 ) ) ;
#57899=CARTESIAN_POINT ( 'NONE',  ( 56.51669371712956291, 7.950000000000000178, -2.130196079827421318 ) ) ;
#57927=CARTESIAN_POINT ( 'NONE',  ( 120.7504301918981184, 3.055000000000002824, -5.291415217122919401 ) ) ;
#57980=CIRCLE ( 'NONE', #127370, 7.950000000000000178 ) ;
#57985=ORIENTED_EDGE ( 'NONE', *, *, #114098, .T. ) ;
#58010=CARTESIAN_POINT ( 'NONE',  ( 96.52083333333332860, 7.949999999999999289, 2.130196079827431532 ) ) ;
#58017=CARTESIAN_POINT ( 'NONE',  ( 14.25109569580971147, 9.301276702823301434, -1.951341953592312883 ) ) ;
#58025=CARTESIAN_POINT ( 'NONE',  ( 127.3704301918981088, -3.055000000000001492, 5.291415217122917625 ) ) ;
#58037=CARTESIAN_POINT ( 'NONE',  ( 107.7712635252314186, 4.472830434245839371, 4.472830434245842035 ) ) ;
#58048=CARTESIAN_POINT ( 'NONE',  ( 100.8287635252314516, 0.000000000000000000, -6.109999999999998543 ) ) ;
#58057=CARTESIAN_POINT ( 'NONE',  ( 99.00000000000000000, 0.000000000000000000, -7.950000000000000178 ) ) ;
#58066=CARTESIAN_POINT ( 'NONE',  ( 34.47459685856478018, 1.637169565754164058, -6.109999999999996767 ) ) ;
#58086=CARTESIAN_POINT ( 'NONE',  ( 63.66252705046289151, 7.949999999999998401, 1.460391307983218338E-15 ) ) ;
#58089=LINE ( 'NONE', #56671, #111703 ) ;
#58096=CARTESIAN_POINT ( 'NONE',  ( 39.57876352523144448, -7.482591942790325086E-16, 6.109999999999998543 ) ) ;
#58136=CARTESIAN_POINT ( 'NONE',  ( 108.9954301918981088, 5.291415217122917625, 3.055000000000002380 ) ) ;
#58157=CARTESIAN_POINT ( 'NONE',  ( 96.47502705046288440, -5.819803920172573086, 5.819803920172573086 ) ) ;
#58186=VECTOR ( 'NONE', #40755, 1000.000000000000000 ) ;
#58189=CARTESIAN_POINT ( 'NONE',  ( 119.7083333333333286, -3.974999999999999201, -6.884901960086287964 ) ) ;
#58204=CARTESIAN_POINT ( 'NONE',  ( 109.9587635252314470, 0.000000000000000000, -6.110000000000001208 ) ) ;
#58209=CARTESIAN_POINT ( 'NONE',  ( 105.8083603837962414, 7.949999999999996625, 2.130196079827431088 ) ) ;
#58215=CARTESIAN_POINT ( 'NONE',  ( 43.39169371712955581, 2.130196079827421762, 7.950000000000001066 ) ) ;
#58221=CARTESIAN_POINT ( 'NONE',  ( 31.77083333333333215, -7.949999999999999289, -2.130196079827426203 ) ) ;
#58231=CARTESIAN_POINT ( 'NONE',  ( 41.41709685856477563, 3.054999999999998828, 5.291415217122922066 ) ) ;
#58233=ORIENTED_EDGE ( 'NONE', *, *, #60905, .T. ) ;
#58253=CARTESIAN_POINT ( 'NONE',  ( 59.26626352523145869, 4.472830434245839371, -4.472830434245838482 ) ) ;
#58285=CARTESIAN_POINT ( 'NONE',  ( 65.09959685856478018, -6.109999999999997655, -1.637169565754160283 ) ) ;
#58334=LINE ( 'NONE', #25635, #124301 ) ;
#58365=CARTESIAN_POINT ( 'NONE',  ( 60.87043019189810877, -3.055000000000001936, 5.291415217122918513 ) ) ;
#58388=CARTESIAN_POINT ( 'NONE',  ( 78.53752705046289861, -9.735942053221456900E-16, 7.949999999999998401 ) ) ;
#58392=CARTESIAN_POINT ( 'NONE',  ( 73.33333333333332860, -6.884901960086287964, 3.974999999999998312 ) ) ;
#58401=CARTESIAN_POINT ( 'NONE',  ( 65.04209685856477563, 5.291415217122923842, -3.054999999999996163 ) ) ;
#58408=CARTESIAN_POINT ( 'NONE',  ( 43.87500000000000000, 7.950000000000000178, 1.460391307983218535E-15 ) ) ;
#58411=CARTESIAN_POINT ( 'NONE',  ( 86.75000000000000000, -9.735942053221458872E-16, 7.950000000000000178 ) ) ;
#58421=CARTESIAN_POINT ( 'NONE',  ( 57.60459685856477563, 1.637169565754164946, -6.109999999999999432 ) ) ;
#58428=LINE ( 'NONE', #102607, #36214 ) ;
#58429=CARTESIAN_POINT ( 'NONE',  ( 54.08333333333332860, 6.884901960086290629, -3.974999999999994316 ) ) ;
#58455=CARTESIAN_POINT ( 'NONE',  ( 104.0370968585647802, -3.054999999999998828, -5.291415217122919401 ) ) ;
#58488=CARTESIAN_POINT ( 'NONE',  ( 55.27126352523142572, 4.472830434245838482, 4.472830434245842035 ) ) ;
#58534=CARTESIAN_POINT ( 'NONE',  ( 5.978975958053759143, 9.486554164729072980, 0.5799792595215604862 ) ) ;
#58536=( BOUNDED_CURVE ( )  B_SPLINE_CURVE ( 2, ( #65162, #88332, #122346, #78171, #54295, #23023, #107891, #52804, #99904, #87603, #110049, #131115, #33271 ),
 .UNSPECIFIED., .F., .F. ) 
 B_SPLINE_CURVE_WITH_KNOTS ( ( 3, 2, 2, 2, 2, 2, 3 ),
 ( 0.4166666666666666852, 0.4194444444444444531, 0.4222222222222222210, 0.4249999999999999889, 0.4277777777777777568, 0.4305555555555555802, 0.4333333333333333481 ),
 .UNSPECIFIED. ) 
 CURVE ( )  GEOMETRIC_REPRESENTATION_ITEM ( )  RATIONAL_B_SPLINE_CURVE ( ( 1.000000000000000000, 0.9659258262890683122, 1.000000000000000000, 0.9659258262890683122, 1.000000000000000000, 0.9659258262890683122, 1.000000000000000000, 0.9659258262890683122, 1.000000000000000000, 0.9659258262890683122, 1.000000000000000000, 0.9659258262890683122, 1.000000000000000000 ) ) 
 REPRESENTATION_ITEM ( '' )  );
#58546=( BOUNDED_CURVE ( )  B_SPLINE_CURVE ( 2, ( #58411, #125772, #35207, #80142, #79449, #68545, #26445, #35922, #13394, #2514, #114844, #102594, #101856 ),
 .UNSPECIFIED., .F., .T. ) 
 B_SPLINE_CURVE_WITH_KNOTS ( ( 3, 2, 2, 2, 2, 2, 3 ),
 ( 0.3833333333333334147, 0.3861111111111111827, 0.3888888888888889506, 0.3916666666666667185, 0.3944444444444444864, 0.3972222222222222543, 0.4000000000000000777 ),
 .UNSPECIFIED. ) 
 CURVE ( )  GEOMETRIC_REPRESENTATION_ITEM ( )  RATIONAL_B_SPLINE_CURVE ( ( 0.9999999999999993339, 0.9659258262890689783, 1.000000000000000000, 0.9659258262890683122, 1.000000000000000000, 0.9659258262890683122, 1.000000000000000000, 0.9659258262890683122, 1.000000000000000000, 0.9659258262890683122, 1.000000000000000000, 0.9659258262890676461, 1.000000000000000666 ) ) 
 REPRESENTATION_ITEM ( '' )  );
#58559=CARTESIAN_POINT ( 'NONE',  ( 99.24586038379624142, 3.974999999999996980, 6.884901960086287964 ) ) ;
#58577=CARTESIAN_POINT ( 'NONE',  ( 94.20876352523144703, -7.482591942790329030E-16, 6.110000000000001208 ) ) ;
#58599=CARTESIAN_POINT ( 'NONE',  ( 85.60459685856478984, 1.637169565754164946, -6.109999999999999432 ) ) ;
#58613=CARTESIAN_POINT ( 'NONE',  ( 77.64126352523146579, 4.472830434245836706, 4.472830434245840259 ) ) ;
#58624=CARTESIAN_POINT ( 'NONE',  ( 65.31250000000000000, 5.819803920172571310, 5.819803920172576639 ) ) ;
#58644=CARTESIAN_POINT ( 'NONE',  ( 56.95419371712956291, 6.884901960086283523, 3.975000000000002753 ) ) ;
#58665=CARTESIAN_POINT ( 'NONE',  ( 116.5212635252314612, -4.472830434245838482, -4.472830434245840259 ) ) ;
#58688=ADVANCED_FACE ( 'NONE', ( #103927 ), #35168, .T. ) ;
#58703=FACE_OUTER_BOUND ( 'NONE', #123008, .T. ) ;
#58744=CARTESIAN_POINT ( 'NONE',  ( 94.91666666666665719, -6.884901960086287076, -3.975000000000000977 ) ) ;
#58751=CYLINDRICAL_SURFACE ( 'NONE', #138038, 7.950000000000000178 ) ;
#58756=CARTESIAN_POINT ( 'NONE',  ( 125.8772101740147917, 2.453750636162616239, -7.181886997138566819 ) ) ;
#58771=CARTESIAN_POINT ( 'NONE',  ( 113.0212635252314186, -4.472830434245839371, -4.472830434245840259 ) ) ;
#58776=CARTESIAN_POINT ( 'NONE',  ( 99.58333333333332860, 6.884901960086290629, -3.974999999999994316 ) ) ;
#58784=CARTESIAN_POINT ( 'NONE',  ( 108.5579301918980946, 6.110000000000000320, -1.637169565754156064 ) ) ;
#58789=CARTESIAN_POINT ( 'NONE',  ( 98.70833333333332860, -3.974999999999999201, -6.884901960086287964 ) ) ;
#58796=VECTOR ( 'NONE', #40423, 1000.000000000000000 ) ;
#58813=B_SPLINE_CURVE_WITH_KNOTS ( 'NONE', 3,
 ( #35568, #111663, #25348, #91359, #135566, #36249, #66731, #23945, #13032, #89200 ),
 .UNSPECIFIED., .F., .F.,
 ( 4, 2, 2, 2, 4 ),
 ( 0.0007022386915571705726, 0.002041165551483828822, 0.003380092411410488048, 0.004719019271337147707, 0.006057946131263806933 ),
 .UNSPECIFIED. ) ;
#58824=ORIENTED_EDGE ( 'NONE', *, *, #54667, .T. ) ;
#58829=CARTESIAN_POINT ( 'NONE',  ( 38.70376352523144448, 6.109999999999998543, 1.122388791418548911E-15 ) ) ;
#58839=VECTOR ( 'NONE', #57806, 1000.000000000000000 ) ;
#58865=CARTESIAN_POINT ( 'NONE',  ( 100.0995968585647944, -6.109999999999998543, -1.637169565754160727 ) ) ;
#58912=CARTESIAN_POINT ( 'NONE',  ( 122.6250000000000000, -7.950000000000000178, -4.867971026610729436E-16 ) ) ;
#58926=CARTESIAN_POINT ( 'NONE',  ( 109.3754301918981042, -5.291415217122920289, -3.055000000000001492 ) ) ;
#58937=CARTESIAN_POINT ( 'NONE',  ( 48.64169371712955581, -2.130196079827424871, -7.949999999999999289 ) ) ;
#58940=AXIS2_PLACEMENT_3D ( 'NONE', #83973, #21363, #132298 ) ;
#58944=CARTESIAN_POINT ( 'NONE',  ( 39.06249999999999289, -5.819803920172572198, -5.819803920172573086 ) ) ;
#58953=DIRECTION ( 'NONE',  ( 0.000000000000000000, 0.000000000000000000, 1.000000000000000000 ) ) ;
#58954=SHAPE_REPRESENTATION ( '1.2 Vise Screw', ( #127880 ), #12041 ) ;
#58956=CYLINDRICAL_SURFACE ( 'NONE', #69899, 7.950000000000000178 ) ;
#58957=CARTESIAN_POINT ( 'NONE',  ( 27.41709685856476142, 3.054999999999998828, 5.291415217122922066 ) ) ;
#58966=CARTESIAN_POINT ( 'NONE',  ( 63.70833333333332860, -3.974999999999999201, -6.884901960086287964 ) ) ;
#58974=CARTESIAN_POINT ( 'NONE',  ( 53.57876352523144448, -7.482591942790325086E-16, 6.109999999999998543 ) ) ;
#59000=CARTESIAN_POINT ( 'NONE',  ( 62.76626352523144448, 4.472830434245838482, -4.472830434245837594 ) ) ;
#59034=CARTESIAN_POINT ( 'NONE',  ( 119.5166937171295558, 7.950000000000000178, -2.130196079827421318 ) ) ;
#59054=ORIENTED_EDGE ( 'NONE', *, *, #105216, .T. ) ;
#59060=CARTESIAN_POINT ( 'NONE',  ( 64.68336038379622721, -2.130196079827426203, 7.949999999999996625 ) ) ;
#59068=CARTESIAN_POINT ( 'NONE',  ( 51.53709685856478018, -3.054999999999999272, -5.291415217122919401 ) ) ;
#59088=CARTESIAN_POINT ( 'NONE',  ( 74.60002705046289861, 5.819803920172570422, 5.819803920172574863 ) ) ;
#59094=CARTESIAN_POINT ( 'NONE',  ( 62.83333333333332149, -6.884901960086287964, 3.974999999999998312 ) ) ;
#59106=CARTESIAN_POINT ( 'NONE',  ( 53.52126352523144703, -4.472830434245839371, -4.472830434245840259 ) ) ;
#59157=CARTESIAN_POINT ( 'NONE',  ( 94.12043019189810877, 3.055000000000001936, -5.291415217122916737 ) ) ;
#59161=DIRECTION ( 'NONE',  ( -1.000000000000000000, -0.000000000000000000, -0.000000000000000000 ) ) ;
#59179=CARTESIAN_POINT ( 'NONE',  ( 43.02126352523142572, -4.472830434245838482, -4.472830434245840259 ) ) ;
#59195=CARTESIAN_POINT ( 'NONE',  ( 27.78752705046289151, 0.000000000000000000, -7.949999999999998401 ) ) ;
#59233=CARTESIAN_POINT ( 'NONE',  ( 80.47916666666664298, -7.950000000000000178, 2.130196079827424427 ) ) ;
#59252=CARTESIAN_POINT ( 'NONE',  ( 101.4333603837962414, 2.130196079827431532, -7.949999999999997513 ) ) ;
#59253=CARTESIAN_POINT ( 'NONE',  ( 10.32500000000000107, 8.432637487761466488, 4.375000000000001776 ) ) ;
#59263=ORIENTED_EDGE ( 'NONE', *, *, #44687, .F. ) ;
#59268=CARTESIAN_POINT ( 'NONE',  ( 98.43793019189811844, -6.110000000000001208, 1.637169565754158951 ) ) ;
#59291=CARTESIAN_POINT ( 'NONE',  ( 86.77126352523141861, 4.472830434245839371, 4.472830434245842035 ) ) ;
#59302=CARTESIAN_POINT ( 'NONE',  ( 73.55793019189812298, 6.110000000000000320, -1.637169565754156064 ) ) ;
#59314=FACE_OUTER_BOUND ( 'NONE', #6338, .T. ) ;
#59331=CARTESIAN_POINT ( 'NONE',  ( 69.78752705046289861, 0.000000000000000000, -7.949999999999998401 ) ) ;
#59345=CARTESIAN_POINT ( 'NONE',  ( 71.75043019189811844, 3.055000000000002824, -5.291415217122919401 ) ) ;
#59349=CARTESIAN_POINT ( 'NONE',  ( 118.5629301918981042, 1.637169565754157174, 6.110000000000002984 ) ) ;
#59365=( BOUNDED_CURVE ( )  B_SPLINE_CURVE ( 2, ( #107334, #74008, #41357, #73305, #108020, #83461, #128396, #117475, #85571, #51553, #129802, #84875, #42111 ),
 .UNSPECIFIED., .F., .T. ) 
 B_SPLINE_CURVE_WITH_KNOTS ( ( 3, 2, 2, 2, 2, 2, 3 ),
 ( 0.7500000000000000000, 0.7527777777777777679, 0.7555555555555555358, 0.7583333333333333037, 0.7611111111111109606, 0.7638888888888887285, 0.7666666666666666075 ),
 .UNSPECIFIED. ) 
 CURVE ( )  GEOMETRIC_REPRESENTATION_ITEM ( )  RATIONAL_B_SPLINE_CURVE ( ( 1.000000000000000000, 0.9659258262890683122, 1.000000000000000000, 0.9659258262890683122, 1.000000000000000000, 0.9659258262890683122, 1.000000000000000000, 0.9659258262890683122, 1.000000000000000000, 0.9659258262890683122, 1.000000000000000000, 0.9659258262890696445, 0.9999999999999986677 ) ) 
 REPRESENTATION_ITEM ( '' )  );
#59418=CARTESIAN_POINT ( 'NONE',  ( 128.9958603837962414, -3.974999999999998312, -6.884901960086286188 ) ) ;
#59435=CARTESIAN_POINT ( 'NONE',  ( 94.62500000000000000, -7.950000000000000178, -4.867971026610729436E-16 ) ) ;
#59456=CARTESIAN_POINT ( 'NONE',  ( 107.4795968585647614, 6.109999999999999432, 1.637169565754164280 ) ) ;
#59466=CARTESIAN_POINT ( 'NONE',  ( 101.2662635252314374, 4.472830434245839371, -4.472830434245838482 ) ) ;
#59508=CARTESIAN_POINT ( 'NONE',  ( 35.64126352523145158, 4.472830434245835818, 4.472830434245840259 ) ) ;
#59533=EDGE_CURVE ( 'NONE', #75066, #13817, #57980, .T. ) ;
#59540=( BOUNDED_CURVE ( )  B_SPLINE_CURVE ( 2, ( #34527, #66458, #69310, #77357, #110624, #46894, #122966, #79512, #132457, #12750, #57024, #55580, #89610 ),
 .UNSPECIFIED., .F., .T. ) 
 B_SPLINE_CURVE_WITH_KNOTS ( ( 3, 2, 2, 2, 2, 2, 3 ),
 ( 0.3666666666666666963, 0.3694444444444445197, 0.3722222222222222876, 0.3750000000000000555, 0.3777777777777778234, 0.3805555555555555913, 0.3833333333333334147 ),
 .UNSPECIFIED. ) 
 CURVE ( )  GEOMETRIC_REPRESENTATION_ITEM ( )  RATIONAL_B_SPLINE_CURVE ( ( 0.9999999999999993339, 0.9659258262890689783, 1.000000000000000000, 0.9659258262890683122, 1.000000000000000000, 0.9659258262890683122, 1.000000000000000000, 0.9659258262890683122, 1.000000000000000000, 0.9659258262890683122, 1.000000000000000000, 0.9659258262890676461, 1.000000000000000666 ) ) 
 REPRESENTATION_ITEM ( '' )  );
#59545=CARTESIAN_POINT ( 'NONE',  ( 103.7454301918981230, -5.291415217122919401, -3.055000000000000604 ) ) ;
#59587=CARTESIAN_POINT ( 'NONE',  ( 28.37086038379622721, 6.884901960086289741, -3.974999999999993427 ) ) ;
#59593=CARTESIAN_POINT ( 'NONE',  ( 116.2083333333333286, -3.974999999999999201, -6.884901960086287964 ) ) ;
#59607=CARTESIAN_POINT ( 'NONE',  ( 112.4379301918981184, -6.110000000000001208, 1.637169565754158951 ) ) ;
#59619=CARTESIAN_POINT ( 'NONE',  ( 34.64169371712954160, -2.130196079827424871, -7.949999999999999289 ) ) ;
#59625=CARTESIAN_POINT ( 'NONE',  ( 34.39583333333333570, -2.130196079827427091, 7.949999999999999289 ) ) ;
#59627=ORIENTED_EDGE ( 'NONE', *, *, #39758, .F. ) ;
#59635=CARTESIAN_POINT ( 'NONE',  ( 0.000000000000000000, 0.000000000000000000, 0.000000000000000000 ) ) ;
#59636=CARTESIAN_POINT ( 'NONE',  ( 26.68793019189810067, 6.110000000000002984, -1.637169565754156730 ) ) ;
#59643=ORIENTED_EDGE ( 'NONE', *, *, #48408, .T. ) ;
#59652=CARTESIAN_POINT ( 'NONE',  ( 48.76626352523144448, 4.472830434245839371, -4.472830434245838482 ) ) ;
#59664=CARTESIAN_POINT ( 'NONE',  ( 59.57919371712955581, 3.975000000000002753, -6.884901960086283523 ) ) ;
#59678=CARTESIAN_POINT ( 'NONE',  ( 67.72459685856476597, -1.637169565754160949, 6.109999999999997655 ) ) ;
#59688=CARTESIAN_POINT ( 'NONE',  ( 100.8958333333333570, -2.130196079827465283, 7.949999999999977973 ) ) ;
#59717=CARTESIAN_POINT ( 'NONE',  ( 118.7875270504628986, 0.000000000000000000, -7.949999999999998401 ) ) ;
#59726=CARTESIAN_POINT ( 'NONE',  ( 108.1874999999999716, -5.819803920172573974, 5.819803920172573086 ) ) ;
#59755=CARTESIAN_POINT ( 'NONE',  ( 45.55793019189811588, 6.110000000000001208, -1.637169565754156286 ) ) ;
#59771=CARTESIAN_POINT ( 'NONE',  ( 20.65000000000000213, 0.000000000000000000, 0.000000000000000000 ) ) ;
#59774=EDGE_CURVE ( 'NONE', #7223, #120796, #2311, .T. ) ;
#59776=CARTESIAN_POINT ( 'NONE',  ( 68.18336038379622721, -2.130196079827426203, 7.949999999999997513 ) ) ;
#59777=CARTESIAN_POINT ( 'NONE',  ( 0.000000000000000000, 0.000000000000000000, 0.000000000000000000 ) ) ;
#59781=CARTESIAN_POINT ( 'NONE',  ( 67.06249999999997158, -5.819803920172572198, -5.819803920172573086 ) ) ;
#59783=EDGE_CURVE ( 'NONE', #24699, #135809, #6954, .T. ) ;
#59790=CARTESIAN_POINT ( 'NONE',  ( 56.00043019189809712, -3.055000000000002380, 5.291415217122920289 ) ) ;
#59840=CARTESIAN_POINT ( 'NONE',  ( 95.87043019189810877, -3.055000000000001492, 5.291415217122917625 ) ) ;
#59851=CARTESIAN_POINT ( 'NONE',  ( 68.08333333333332860, 6.884901960086290629, -3.974999999999994316 ) ) ;
#59861=CARTESIAN_POINT ( 'NONE',  ( 48.27126352523143993, 4.472830434245838482, 4.472830434245842035 ) ) ;
#59901=DIRECTION ( 'NONE',  ( 0.000000000000000000, 0.000000000000000000, 1.000000000000000000 ) ) ;
#59919=CARTESIAN_POINT ( 'NONE',  ( 77.93293019189812298, 1.637169565754156730, 6.110000000000001208 ) ) ;
#59947=CARTESIAN_POINT ( 'NONE',  ( 103.4750270504628702, -5.819803920172572198, 5.819803920172572198 ) ) ;
#59960=CARTESIAN_POINT ( 'NONE',  ( 80.50043019189810423, -3.055000000000002380, 5.291415217122920289 ) ) ;
#59966=CARTESIAN_POINT ( 'NONE',  ( 1.500000000000000000, 0.000000000000000000, 0.000000000000000000 ) ) ;
#59978=CARTESIAN_POINT ( 'NONE',  ( 80.35459685856474721, -1.637169565754161615, 6.110000000000000320 ) ) ;
#59988=CARTESIAN_POINT ( 'NONE',  ( 79.24543019189810877, -5.291415217122918513, -3.055000000000000160 ) ) ;
#60002=CARTESIAN_POINT ( 'NONE',  ( 65.60416666666665719, 2.130196079827422206, 7.950000000000001954 ) ) ;
#60040=CARTESIAN_POINT ( 'NONE',  ( 73.79209685856477563, -5.291415217122921177, 3.054999999999999272 ) ) ;
#60043=AXIS2_PLACEMENT_3D ( 'NONE', #71466, #83797, #28689 ) ;
#60047=CARTESIAN_POINT ( 'NONE',  ( 109.5212635252314470, -4.472830434245838482, -4.472830434245840259 ) ) ;
#60056=EDGE_CURVE ( 'NONE', #32830, #33782, #78639, .T. ) ;
#60066=CARTESIAN_POINT ( 'NONE',  ( 113.8750000000000000, 7.950000000000000178, 1.460391307983218535E-15 ) ) ;
#60067=ADVANCED_FACE ( 'NONE', ( #111993 ), #88089, .T. ) ;
#60079=CARTESIAN_POINT ( 'NONE',  ( 12.99696575335027049, -8.842958852558309601, -3.475790897895063125 ) ) ;
#60117=CARTESIAN_POINT ( 'NONE',  ( 127.3916937171295558, 2.130196079827421762, 7.950000000000001066 ) ) ;
#60133=CARTESIAN_POINT ( 'NONE',  ( 93.02083333333331439, 7.949999999999999289, 2.130196079827431532 ) ) ;
#60147=CARTESIAN_POINT ( 'NONE',  ( 125.7294590726101546, -0.005845708547400866630, -7.736937294360648920 ) ) ;
#60159=CARTESIAN_POINT ( 'NONE',  ( 111.2712635252314612, 4.472830434245839371, 4.472830434245842035 ) ) ;
#60166=CARTESIAN_POINT ( 'NONE',  ( 109.2870968585647944, 3.054999999999997495, 5.291415217122919401 ) ) ;
#60215=CARTESIAN_POINT ( 'NONE',  ( 40.74543019189810877, -5.291415217122918513, -3.055000000000000160 ) ) ;
#60256=CARTESIAN_POINT ( 'NONE',  ( 104.7662635252314516, 4.472830434245839371, -4.472830434245839371 ) ) ;
#60280=ORIENTED_EDGE ( 'NONE', *, *, #99965, .F. ) ;
#60283=ORIENTED_EDGE ( 'NONE', *, *, #76128, .F. ) ;
#60307=CARTESIAN_POINT ( 'NONE',  ( 122.1875000000000000, -5.819803920172573086, 5.819803920172572198 ) ) ;
#60322=CARTESIAN_POINT ( 'NONE',  ( 116.6670968585647756, -3.055000000000000160, -5.291415217122921177 ) ) ;
#60330=CARTESIAN_POINT ( 'NONE',  ( 35.66252705046288440, 7.949999999999998401, 1.460391307983218338E-15 ) ) ;
#60335=CARTESIAN_POINT ( 'NONE',  ( 34.10416666666665719, 2.130196079827422206, 7.950000000000001954 ) ) ;
#60346=CARTESIAN_POINT ( 'NONE',  ( 29.45876352523143993, 0.000000000000000000, -6.110000000000001208 ) ) ;
#60362=DIRECTION ( 'NONE',  ( -1.000000000000000000, -0.000000000000000000, -0.000000000000000000 ) ) ;
#60369=CARTESIAN_POINT ( 'NONE',  ( 50.95376352523145158, -6.109999999999998543, -3.741295971395162543E-16 ) ) ;
#60371=CARTESIAN_POINT ( 'NONE',  ( 124.8125000000000142, 5.819803920172571310, 5.819803920172576639 ) ) ;
#60398=CARTESIAN_POINT ( 'NONE',  ( 66.84959685856478018, 6.109999999999996767, 1.637169565754163836 ) ) ;
#60415=VECTOR ( 'NONE', #53849, 1000.000000000000000 ) ;
#60448=CARTESIAN_POINT ( 'NONE',  ( 108.3333333333333428, -6.884901960086287964, 3.974999999999998312 ) ) ;
#60453=CARTESIAN_POINT ( 'NONE',  ( 120.5375270504628844, -9.735942053221456900E-16, 7.949999999999998401 ) ) ;
#60480=CARTESIAN_POINT ( 'NONE',  ( 44.82876352523145158, 0.000000000000000000, -6.109999999999999432 ) ) ;
#60503=CARTESIAN_POINT ( 'NONE',  ( 62.78752705046289151, 0.000000000000000000, -7.949999999999998401 ) ) ;
#60507=CARTESIAN_POINT ( 'NONE',  ( 61.81249999999998579, 5.819803920172571310, 5.819803920172575751 ) ) ;
#60512=CARTESIAN_POINT ( 'NONE',  ( 33.95833333333332860, 3.974999999999997424, 6.884901960086288852 ) ) ;
#60516=CARTESIAN_POINT ( 'NONE',  ( 57.60459685856477563, 1.637169565754164946, -6.109999999999999432 ) ) ;
#60518=DIRECTION ( 'NONE',  ( -1.000000000000000000, -0.000000000000000000, -0.000000000000000000 ) ) ;
#60545=AXIS2_PLACEMENT_3D ( 'NONE', #126157, #17374, #26124 ) ;
#60548=EDGE_CURVE ( 'NONE', #38530, #107625, #66294, .T. ) ;
#60579=CARTESIAN_POINT ( 'NONE',  ( 91.64126352523143737, 4.472830434245835818, 4.472830434245840259 ) ) ;
#60607=CARTESIAN_POINT ( 'NONE',  ( 46.37543019189810423, -5.291415217122920289, -3.055000000000001492 ) ) ;
#60616=DIRECTION ( 'NONE',  ( 0.000000000000000000, 0.000000000000000000, 1.000000000000000000 ) ) ;
#60663=CARTESIAN_POINT ( 'NONE',  ( 71.66209685856478018, -5.291415217122919401, 3.054999999999998384 ) ) ;
#60666=CARTESIAN_POINT ( 'NONE',  ( 74.89169371712955581, 2.130196079827421762, 7.950000000000000178 ) ) ;
#60690=CARTESIAN_POINT ( 'NONE',  ( 92.97502705046289861, -5.819803920172572198, 5.819803920172572198 ) ) ;
#60691=CARTESIAN_POINT ( 'NONE',  ( 72.02083333333334281, 7.949999999999998401, 2.130196079827431532 ) ) ;
#60700=AXIS2_PLACEMENT_3D ( 'NONE', #30323, #85397, #31060 ) ;
#60704=CARTESIAN_POINT ( 'NONE',  ( 81.66709685856477563, -3.055000000000000160, -5.291415217122921177 ) ) ;
#60722=CARTESIAN_POINT ( 'NONE',  ( 70.43793019189810423, -6.110000000000001208, 1.637169565754158951 ) ) ;
#60746=COLOUR_RGB ( '', 0.72549020, 0.75294118, 0.79215686) ;
#60750=CARTESIAN_POINT ( 'NONE',  ( 65.16666666666667140, 6.884901960086285300, 3.975000000000003642 ) ) ;
#60755=CARTESIAN_POINT ( 'NONE',  ( 54.03752705046288440, -9.735942053221456900E-16, 7.949999999999998401 ) ) ;
#60785=CARTESIAN_POINT ( 'NONE',  ( 74.95876352523143282, 0.000000000000000000, -6.110000000000001208 ) ) ;
#60789=CARTESIAN_POINT ( 'NONE',  ( 109.0837635252314470, -6.110000000000001208, -3.741295971395164515E-16 ) ) ;
#60804=CARTESIAN_POINT ( 'NONE',  ( 113.8291937171295558, -3.975000000000001865, 6.884901960086284411 ) ) ;
#60840=CARTESIAN_POINT ( 'NONE',  ( 25.08376352523143638, -6.110000000000001208, -3.741295971395164515E-16 ) ) ;
#60857=CARTESIAN_POINT ( 'NONE',  ( 122.5791937171295700, 3.975000000000002753, -6.884901960086283523 ) ) ;
#60873=CARTESIAN_POINT ( 'NONE',  ( 78.72916666666667140, 7.950000000000001954, -2.130196079827421762 ) ) ;
#60887=CARTESIAN_POINT ( 'NONE',  ( 126.1031985511058622, 5.455129984951537558, -4.927627306428293608 ) ) ;
#60898=CARTESIAN_POINT ( 'NONE',  ( 112.0004301918981042, -3.055000000000002380, 5.291415217122920289 ) ) ;
#60905=EDGE_CURVE ( 'NONE', #93164, #125049, #42175, .T. ) ;
#60907=CARTESIAN_POINT ( 'NONE',  ( 75.95833333333332860, 3.974999999999997424, 6.884901960086288852 ) ) ;
#60909=CARTESIAN_POINT ( 'NONE',  ( 105.7870968585647802, 3.054999999999997495, 5.291415217122919401 ) ) ;
#60936=AXIS2_PLACEMENT_3D ( 'NONE', #41512, #8832, #107488 ) ;
#60938=CARTESIAN_POINT ( 'NONE',  ( 110.7454301918981088, -5.291415217122918513, -3.055000000000000160 ) ) ;
#60964=CARTESIAN_POINT ( 'NONE',  ( 33.45376352523145158, -6.109999999999998543, -3.741295971395162543E-16 ) ) ;
#60990=DIRECTION ( 'NONE',  ( -1.000000000000000000, -0.000000000000000000, -0.000000000000000000 ) ) ;
#60998=CARTESIAN_POINT ( 'NONE',  ( 102.7245968585647802, -1.637169565754161171, 6.109999999999998543 ) ) ;
#61051=CARTESIAN_POINT ( 'NONE',  ( 111.6875000000000000, -5.819803920172573086, 5.819803920172572198 ) ) ;
#61065=CARTESIAN_POINT ( 'NONE',  ( 110.1045968585647756, 1.637169565754164946, -6.109999999999999432 ) ) ;
#61073=CARTESIAN_POINT ( 'NONE',  ( 33.32919371712955581, -3.975000000000001865, 6.884901960086284411 ) ) ;
#61079=CARTESIAN_POINT ( 'NONE',  ( 32.20833333333332149, -3.974999999999999201, -6.884901960086287964 ) ) ;
#61091=CARTESIAN_POINT ( 'NONE',  ( 31.20876352523144348, -7.482591942790329030E-16, 6.110000000000001208 ) ) ;
#61096=ORIENTED_EDGE ( 'NONE', *, *, #35226, .F. ) ;
#61104=CARTESIAN_POINT ( 'NONE',  ( 51.91709685856476852, 3.054999999999998828, 5.291415217122922066 ) ) ;
#61116=CARTESIAN_POINT ( 'NONE',  ( 45.99543019189810877, 5.291415217122916737, 3.055000000000001936 ) ) ;
#61117=ORIENTED_EDGE ( 'NONE', *, *, #30334, .T. ) ;
#61122=VECTOR ( 'NONE', #126613, 1000.000000000000000 ) ;
#61144=CARTESIAN_POINT ( 'NONE',  ( 66.99543019189812298, 5.291415217122916737, 3.055000000000001936 ) ) ;
#61164=ORIENTED_EDGE ( 'NONE', *, *, #108429, .F. ) ;
#61185=CARTESIAN_POINT ( 'NONE',  ( 109.2083333333333428, -3.974999999999999201, -6.884901960086287964 ) ) ;
#61202=CARTESIAN_POINT ( 'NONE',  ( 58.75000000000000000, -9.735942053221458872E-16, 7.950000000000000178 ) ) ;
#61219=CARTESIAN_POINT ( 'NONE',  ( 48.32876352523145158, 0.000000000000000000, -6.109999999999999432 ) ) ;
#61238=EDGE_CURVE ( 'NONE', #128126, #71447, #121604, .T. ) ;
#61242=CARTESIAN_POINT ( 'NONE',  ( 62.35002705046287730, -5.819803920172572198, -5.819803920172572198 ) ) ;
#61246=CARTESIAN_POINT ( 'NONE',  ( 64.87499999999998579, 7.950000000000000178, 1.460391307983218535E-15 ) ) ;
#61255=DIRECTION ( 'NONE',  ( -1.000000000000000000, -0.000000000000000000, -0.000000000000000000 ) ) ;
#61256=CARTESIAN_POINT ( 'NONE',  ( 52.50043019189811133, -3.055000000000002380, 5.291415217122920289 ) ) ;
#61268=CARTESIAN_POINT ( 'NONE',  ( 99.53752705046289861, -9.735942053221456900E-16, 7.949999999999998401 ) ) ;
#61288=ADVANCED_FACE ( 'NONE', ( #89704 ), #31764, .T. ) ;
#61309=CARTESIAN_POINT ( 'NONE',  ( 93.24543019189812298, -5.291415217122918513, -3.055000000000000160 ) ) ;
#61331=CARTESIAN_POINT ( 'NONE',  ( 41.27126352523144703, 4.472830434245838482, 4.472830434245842035 ) ) ;
#61339=CARTESIAN_POINT ( 'NONE',  ( 0.000000000000000000, 0.000000000000000000, 0.000000000000000000 ) ) ;
#61360=ORIENTED_EDGE ( 'NONE', *, *, #64493, .F. ) ;
#61361=CARTESIAN_POINT ( 'NONE',  ( 66.47916666666665719, -7.950000000000000178, 2.130196079827424427 ) ) ;
#61382=CARTESIAN_POINT ( 'NONE',  ( 78.22459685856479439, -1.637169565754161171, 6.109999999999998543 ) ) ;
#61404=CARTESIAN_POINT ( 'NONE',  ( 95.60002705046287019, 5.819803920172570422, 5.819803920172574863 ) ) ;
#61411=DIRECTION ( 'NONE',  ( -1.000000000000000000, -0.000000000000000000, -0.000000000000000000 ) ) ;
#61418=CARTESIAN_POINT ( 'NONE',  ( 46.60002705046288440, 5.819803920172570422, 5.819803920172575751 ) ) ;
#61421=CARTESIAN_POINT ( 'NONE',  ( 86.62543019189811844, 5.291415217122919401, 3.055000000000002824 ) ) ;
#61440=CARTESIAN_POINT ( 'NONE',  ( 74.52126352523141861, -4.472830434245839371, -4.472830434245840259 ) ) ;
#61449=EDGE_LOOP ( 'NONE', ( #76658, #51285, #75530, #98444 ) ) ;
#61469=ADVANCED_FACE ( 'NONE', ( #51216 ), #6931, .T. ) ;
#61479=CARTESIAN_POINT ( 'NONE',  ( 27.00000000000000711, -4.501766353396367215, -4.693270563879029744 ) ) ;
#61490=CARTESIAN_POINT ( 'NONE',  ( 69.41709685856477563, 3.054999999999998828, 5.291415217122922066 ) ) ;
#61496=CARTESIAN_POINT ( 'NONE',  ( 107.4795968585647614, 6.109999999999999432, 1.637169565754164280 ) ) ;
#61504=CARTESIAN_POINT ( 'NONE',  ( 35.66252705046288440, 7.949999999999998401, 1.460391307983218338E-15 ) ) ;
#61521=EDGE_CURVE ( 'NONE', #64622, #36177, #85242, .T. ) ;
#61527=CARTESIAN_POINT ( 'NONE',  ( 12.52996815765592942, -8.713228220513846267, 3.789303709965370359 ) ) ;
#61558=CARTESIAN_POINT ( 'NONE',  ( 121.9958603837962272, -3.974999999999998312, -6.884901960086286188 ) ) ;
#61572=CARTESIAN_POINT ( 'NONE',  ( 82.81250000000000000, 5.819803920172571310, 5.819803920172575751 ) ) ;
#61595=CARTESIAN_POINT ( 'NONE',  ( 98.58376352523144703, -6.110000000000001208, -3.741295971395164515E-16 ) ) ;
#61606=CARTESIAN_POINT ( 'NONE',  ( 91.49543019189812298, 5.291415217122916737, 3.055000000000001936 ) ) ;
#61630=CARTESIAN_POINT ( 'NONE',  ( 115.7037635252314516, 6.109999999999998543, 1.122388791418548911E-15 ) ) ;
#61651=CARTESIAN_POINT ( 'NONE',  ( 28.34959685856477662, 6.109999999999996767, 1.637169565754163836 ) ) ;
#61685=CARTESIAN_POINT ( 'NONE',  ( 100.9745968585647660, 1.637169565754164280, -6.109999999999997655 ) ) ;
#61733=CARTESIAN_POINT ( 'NONE',  ( 109.2083333333333428, -3.974999999999999201, -6.884901960086287964 ) ) ;
#61741=ORIENTED_EDGE ( 'NONE', *, *, #12988, .T. ) ;
#61746=CARTESIAN_POINT ( 'NONE',  ( 107.4795968585647614, 6.109999999999999432, 1.637169565754164280 ) ) ;
#61754=CARTESIAN_POINT ( 'NONE',  ( 36.82919371712956291, -3.975000000000001865, 6.884901960086284411 ) ) ;
#61761=CARTESIAN_POINT ( 'NONE',  ( 126.5837635252314612, -6.110000000000001208, -3.741295971395164515E-16 ) ) ;
#61769=CARTESIAN_POINT ( 'NONE',  ( 27.56293019189811133, 1.637169565754157174, 6.110000000000002984 ) ) ;
#61779=ORIENTED_EDGE ( 'NONE', *, *, #68538, .T. ) ;
#61780=CARTESIAN_POINT ( 'NONE',  ( 59.79209685856477563, -5.291415217122921177, 3.054999999999999272 ) ) ;
#61791=CARTESIAN_POINT ( 'NONE',  ( 51.24543019189811588, -5.291415217122918513, -3.055000000000000160 ) ) ;
#61801=CARTESIAN_POINT ( 'NONE',  ( 60.89169371712955581, 2.130196079827421762, 7.950000000000000178 ) ) ;
#61805=CARTESIAN_POINT ( 'NONE',  ( 45.14169371712955581, -2.130196079827424871, -7.949999999999998401 ) ) ;
#61819=FACE_OUTER_BOUND ( 'NONE', #76321, .T. ) ;
#61821=CARTESIAN_POINT ( 'NONE',  ( 52.99543019189811588, 5.291415217122916737, 3.055000000000001936 ) ) ;
#61826=VERTEX_POINT ( 'NONE', #72663 ) ;
#61828=AXIS2_PLACEMENT_3D ( 'NONE', #96469, #87776, #1 ) ;
#61844=CARTESIAN_POINT ( 'NONE',  ( 54.91252705046288440, -7.949999999999998401, -4.867971026610728450E-16 ) ) ;
#61900=CARTESIAN_POINT ( 'NONE',  ( 50.80793019189810167, -6.109999999999999432, 1.637169565754158507 ) ) ;
#61908=( BOUNDED_CURVE ( )  B_SPLINE_CURVE ( 2, ( #69886, #126356, #116204, #114746, #105316, #116909, #138689, #103865, #48821, #16894, #103178, #36503, #27045 ),
 .UNSPECIFIED., .F., .T. ) 
 B_SPLINE_CURVE_WITH_KNOTS ( ( 3, 2, 2, 2, 2, 2, 3 ),
 ( 0.9166666666666666297, 0.9194444444444443976, 0.9222222222222222765, 0.9250000000000000444, 0.9277777777777778123, 0.9305555555555555802, 0.9333333333333333481 ),
 .UNSPECIFIED. ) 
 CURVE ( )  GEOMETRIC_REPRESENTATION_ITEM ( )  RATIONAL_B_SPLINE_CURVE ( ( 1.000000000000000000, 0.9659258262890683122, 1.000000000000000000, 0.9659258262890683122, 1.000000000000000000, 0.9659258262890683122, 1.000000000000000000, 0.9659258262890683122, 1.000000000000000000, 0.9659258262890683122, 1.000000000000000000, 0.9659258262890683122, 1.000000000000000000 ) ) 
 REPRESENTATION_ITEM ( '' )  );
#61924=CARTESIAN_POINT ( 'NONE',  ( 62.05836038379622011, -7.949999999999997513, -2.130196079827425759 ) ) ;
#61930=CARTESIAN_POINT ( 'NONE',  ( 59.77083333333332860, -7.949999999999999289, -2.130196079827426203 ) ) ;
#61939=CARTESIAN_POINT ( 'NONE',  ( 55.27126352523143282, 4.472830434245839371, 4.472830434245842035 ) ) ;
#61951=CARTESIAN_POINT ( 'NONE',  ( 99.82919371712955581, -3.975000000000001865, 6.884901960086284411 ) ) ;
#61965=CARTESIAN_POINT ( 'NONE',  ( 71.82919371712957002, -3.975000000000001865, 6.884901960086284411 ) ) ;
#61974=CARTESIAN_POINT ( 'NONE',  ( 62.78752705046289151, 0.000000000000000000, -7.949999999999998401 ) ) ;
#61994=CARTESIAN_POINT ( 'NONE',  ( 92.95376352523145158, -6.109999999999998543, -3.741295971395162543E-16 ) ) ;
#62016=CARTESIAN_POINT ( 'NONE',  ( 43.75043019189810423, 3.055000000000002824, -5.291415217122919401 ) ) ;
#62069=CARTESIAN_POINT ( 'NONE',  ( 76.03709685856478018, -3.054999999999999272, -5.291415217122919401 ) ) ;
#62093=CARTESIAN_POINT ( 'NONE',  ( 96.03752705046289861, -9.735942053221456900E-16, 7.949999999999998401 ) ) ;
#62104=CARTESIAN_POINT ( 'NONE',  ( 89.39626352523144703, 4.472830434245840259, -4.472830434245839371 ) ) ;
#62121=CARTESIAN_POINT ( 'NONE',  ( 73.50043019189811844, -3.055000000000002380, 5.291415217122920289 ) ) ;
#62178=CARTESIAN_POINT ( 'NONE',  ( 75.39626352523141861, 4.472830434245840259, -4.472830434245838482 ) ) ;
#62184=CARTESIAN_POINT ( 'NONE',  ( 104.4170968585647756, 3.054999999999998828, 5.291415217122922066 ) ) ;
#62203=CARTESIAN_POINT ( 'NONE',  ( 113.9750270504628844, -5.819803920172573086, 5.819803920172573086 ) ) ;
#62251=CARTESIAN_POINT ( 'NONE',  ( 120.6833603837962414, -2.130196079827426203, 7.949999999999997513 ) ) ;
#62265=CARTESIAN_POINT ( 'NONE',  ( 82.22916666666665719, 7.950000000000001954, -2.130196079827421762 ) ) ;
#62293=CARTESIAN_POINT ( 'NONE',  ( 106.4587635252314328, 0.000000000000000000, -6.110000000000001208 ) ) ;
#62301=( BOUNDED_CURVE ( )  B_SPLINE_CURVE ( 2, ( #106294, #114358, #6973, #51259, #138258, #38943, #95453, #104906, #125964, #5574, #49845, #107745, #62859 ),
 .UNSPECIFIED., .F., .F. ) 
 B_SPLINE_CURVE_WITH_KNOTS ( ( 3, 2, 2, 2, 2, 2, 3 ),
 ( 0.9000000000000000222, 0.9027777777777777901, 0.9055555555555555580, 0.9083333333333333259, 0.9111111111111110938, 0.9138888888888888618, 0.9166666666666666297 ),
 .UNSPECIFIED. ) 
 CURVE ( )  GEOMETRIC_REPRESENTATION_ITEM ( )  RATIONAL_B_SPLINE_CURVE ( ( 1.000000000000000000, 0.9659258262890683122, 1.000000000000000000, 0.9659258262890683122, 1.000000000000000000, 0.9659258262890683122, 1.000000000000000000, 0.9659258262890683122, 1.000000000000000000, 0.9659258262890683122, 1.000000000000000000, 0.9659258262890683122, 1.000000000000000000 ) ) 
 REPRESENTATION_ITEM ( '' )  );
#62303=CARTESIAN_POINT ( 'NONE',  ( 94.84959685856476597, 6.109999999999996767, 1.637169565754163836 ) ) ;
#62310=( BOUNDED_CURVE ( )  B_SPLINE_CURVE ( 2, ( #58057, #33446, #58789, #122539, #91380, #132756, #69636, #750, #77647, #13760, #121816, #134895, #2903 ),
 .UNSPECIFIED., .F., .F. ) 
 B_SPLINE_CURVE_WITH_KNOTS ( ( 3, 2, 2, 2, 2, 2, 3 ),
 ( 0.2666666666666666075, 0.2694444444444443754, 0.2722222222222221433, 0.2750000000000000222, 0.2777777777777777901, 0.2805555555555555580, 0.2833333333333333259 ),
 .UNSPECIFIED. ) 
 CURVE ( )  GEOMETRIC_REPRESENTATION_ITEM ( )  RATIONAL_B_SPLINE_CURVE ( ( 1.000000000000000666, 0.9659258262890676461, 1.000000000000000000, 0.9659258262890683122, 1.000000000000000000, 0.9659258262890683122, 1.000000000000000000, 0.9659258262890683122, 1.000000000000000000, 0.9659258262890683122, 1.000000000000000000, 0.9659258262890683122, 1.000000000000000000 ) ) 
 REPRESENTATION_ITEM ( '' )  );
#62311=CARTESIAN_POINT ( 'NONE',  ( 128.1437635252314351, 0.000000000000000000, -6.109999999999999432 ) ) ;
#62316=B_SPLINE_CURVE_WITH_KNOTS ( 'NONE', 3,
 ( #130724, #56026, #85751, #119097, #19781, #31389, #108190, #141584, #75612, #136396, #124104, #24780, #23342, #3024, #69028, #133564, #25483, #89332, #70489, #81339, #134274, #114636, #123422, #36386, #3704, #24082, #67616, #12471 ),
 .UNSPECIFIED., .F., .F.,
 ( 4, 2, 2, 2, 2, 2, 2, 2, 2, 2, 2, 2, 2, 4 ),
 ( 0.000000000000000000, 0.001834580916944877167, 0.002751871375417315642, 0.003669161833889754334, 0.004586452292362193026, 0.005503742750834631284, 0.006421033209307069542, 0.007338323667779508667, 0.008255614126251946058, 0.009172904584724386051, 0.01100748550166926257, 0.01192477596014169909, 0.01284206641861413561, 0.01467664733555900693 ),
 .UNSPECIFIED. ) ;
#62358=CARTESIAN_POINT ( 'NONE',  ( 30.39126352523144448, -4.472830434245838482, -4.472830434245838482 ) ) ;
#62392=CARTESIAN_POINT ( 'NONE',  ( 92.07876352523145158, -7.482591942790327058E-16, 6.109999999999999432 ) ) ;
#62412=VECTOR ( 'NONE', #121995, 1000.000000000000000 ) ;
#62441=CARTESIAN_POINT ( 'NONE',  ( 109.7916666666666572, 3.975000000000003642, -6.884901960086285300 ) ) ;
#62442=ADVANCED_FACE ( 'NONE', ( #81018 ), #3410, .T. ) ;
#62453=CARTESIAN_POINT ( 'NONE',  ( 106.4587635252314328, 0.000000000000000000, -6.110000000000001208 ) ) ;
#62459=CARTESIAN_POINT ( 'NONE',  ( 41.35002705046288440, -5.819803920172572198, -5.819803920172572198 ) ) ;
#62464=CARTESIAN_POINT ( 'NONE',  ( 25.79166666666665719, 3.975000000000003642, -6.884901960086285300 ) ) ;
#62472=CARTESIAN_POINT ( 'NONE',  ( 124.8912635252314516, -4.472830434245839371, -4.472830434245839371 ) ) ;
#62480=SURFACE_STYLE_FILL_AREA ( #40041 ) ;
#62484=CARTESIAN_POINT ( 'NONE',  ( 49.00043019189810423, -3.055000000000002380, 5.291415217122920289 ) ) ;
#62494=CARTESIAN_POINT ( 'NONE',  ( 43.37043019189810877, -3.055000000000001492, 5.291415217122917625 ) ) ;
#62530=CARTESIAN_POINT ( 'NONE',  ( 55.91209685856478018, 5.291415217122921177, -3.054999999999994831 ) ) ;
#62571=EDGE_CURVE ( 'NONE', #67893, #10128, #87466, .T. ) ;
#62599=CARTESIAN_POINT ( 'NONE',  ( 40.74543019189810877, -5.291415217122919401, -3.055000000000000604 ) ) ;
#62625=CYLINDRICAL_SURFACE ( 'NONE', #40444, 7.950000000000000178 ) ;
#62626=CARTESIAN_POINT ( 'NONE',  ( 104.6416937171295416, -2.130196079827424871, -7.949999999999998401 ) ) ;
#62627=CARTESIAN_POINT ( 'NONE',  ( 65.70419371712955581, -6.884901960086285300, -3.975000000000000089 ) ) ;
#62632=CARTESIAN_POINT ( 'NONE',  ( 52.62499999999999289, -7.950000000000000178, -4.867971026610729436E-16 ) ) ;
#62639=CARTESIAN_POINT ( 'NONE',  ( 34.10416666666665719, 2.130196079827498146, 7.949999999999958433 ) ) ;
#62640=CARTESIAN_POINT ( 'NONE',  ( 42.87543019189810423, -5.291415217122920289, -3.055000000000001492 ) ) ;
#62642=ORIENTED_EDGE ( 'NONE', *, *, #135821, .F. ) ;
#62644=AXIS2_PLACEMENT_3D ( 'NONE', #50076, #60990, #14575 ) ;
#62662=CARTESIAN_POINT ( 'NONE',  ( 88.74586038379622721, 3.974999999999996980, 6.884901960086287964 ) ) ;
#62663=CARTESIAN_POINT ( 'NONE',  ( 79.53709685856478018, -3.054999999999998828, -5.291415217122919401 ) ) ;
#62667=CARTESIAN_POINT ( 'NONE',  ( 72.99586038379622721, -3.974999999999998312, -6.884901960086286188 ) ) ;
#62701=CARTESIAN_POINT ( 'NONE',  ( 82.74543019189812298, -5.291415217122918513, -3.055000000000000160 ) ) ;
#62729=CARTESIAN_POINT ( 'NONE',  ( 32.08376352523143993, -6.110000000000001208, -3.741295971395164515E-16 ) ) ;
#62777=VECTOR ( 'NONE', #34209, 1000.000000000000000 ) ;
#62779=CARTESIAN_POINT ( 'NONE',  ( 79.39126352523146579, -4.472830434245839371, -4.472830434245839371 ) ) ;
#62809=CARTESIAN_POINT ( 'NONE',  ( 93.85002705046289861, -5.819803920172572198, -5.819803920172572198 ) ) ;
#62822=CARTESIAN_POINT ( 'NONE',  ( 45.87086038379622721, 6.884901960086289741, -3.974999999999993427 ) ) ;
#62825=CARTESIAN_POINT ( 'NONE',  ( 86.04209685856477563, 5.291415217122923842, -3.054999999999996163 ) ) ;
#62843=CARTESIAN_POINT ( 'NONE',  ( 78.16709685856476142, -3.055000000000000160, -5.291415217122921177 ) ) ;
#62859=CARTESIAN_POINT ( 'NONE',  ( 33.03752705046289151, -9.735942053221456900E-16, 7.949999999999998401 ) ) ;
#62879=ORIENTED_EDGE ( 'NONE', *, *, #32571, .T. ) ;
#62905=CARTESIAN_POINT ( 'NONE',  ( 65.04209685856477563, 5.291415217122923842, -3.054999999999996163 ) ) ;
#62913=CARTESIAN_POINT ( 'NONE',  ( 113.4587635252314470, 0.000000000000000000, -6.110000000000001208 ) ) ;
#62942=CARTESIAN_POINT ( 'NONE',  ( 10.90341945100486143, -8.451216681753212612, -4.339032109071985666 ) ) ;
#62957=CARTESIAN_POINT ( 'NONE',  ( 26.97959685856476497, 6.109999999999999432, 1.637169565754164280 ) ) ;
#62974=CARTESIAN_POINT ( 'NONE',  ( 0.000000000000000000, 9.735942053221458872E-16, -7.950000000000000178 ) ) ;
#62978=CARTESIAN_POINT ( 'NONE',  ( 93.85002705046288440, -5.819803920172573086, -5.819803920172573086 ) ) ;
#62979=CARTESIAN_POINT ( 'NONE',  ( 121.8500270504628702, -5.819803920172572198, -5.819803920172572198 ) ) ;
#63010=DIRECTION ( 'NONE',  ( 0.000000000000000000, 0.000000000000000000, 1.000000000000000000 ) ) ;
#63019=ORIENTED_EDGE ( 'NONE', *, *, #125135, .T. ) ;
#63021=CARTESIAN_POINT ( 'NONE',  ( 97.56293019189810423, 1.637169565754157174, 6.110000000000002984 ) ) ;
#63032=CARTESIAN_POINT ( 'NONE',  ( 96.45376352523145158, -6.109999999999998543, -3.741295971395162543E-16 ) ) ;
#63062=EDGE_LOOP ( 'NONE', ( #88054, #87344, #51566, #138421 ) ) ;
#63066=AXIS2_PLACEMENT_3D ( 'NONE', #100732, #133374, #109460 ) ;
#63118=CARTESIAN_POINT ( 'NONE',  ( 91.49543019189812298, 5.291415217122917625, 3.055000000000002380 ) ) ;
#63144=EDGE_LOOP ( 'NONE', ( #25261, #43092, #54029, #84819 ) ) ;
#63165=VECTOR ( 'NONE', #30148, 1000.000000000000000 ) ;
#63171=( BOUNDED_CURVE ( )  B_SPLINE_CURVE ( 2, ( #134526, #46841, #78001, #67867, #46097, #113447, #14137, #133799, #58429, #35938, #135249, #35223, #102608 ),
 .UNSPECIFIED., .F., .F. ) 
 B_SPLINE_CURVE_WITH_KNOTS ( ( 3, 2, 2, 2, 2, 2, 3 ),
 ( 0.6833333333333334592, 0.6861111111111112271, 0.6888888888888889950, 0.6916666666666667629, 0.6944444444444445308, 0.6972222222222222987, 0.7000000000000000666 ),
 .UNSPECIFIED. ) 
 CURVE ( )  GEOMETRIC_REPRESENTATION_ITEM ( )  RATIONAL_B_SPLINE_CURVE ( ( 0.9999999999999986677, 0.9659258262890696445, 1.000000000000000000, 0.9659258262890683122, 1.000000000000000000, 0.9659258262890683122, 1.000000000000000000, 0.9659258262890683122, 1.000000000000000000, 0.9659258262890683122, 1.000000000000000000, 0.9659258262890669799, 1.000000000000001332 ) ) 
 REPRESENTATION_ITEM ( '' )  );
#63174=CARTESIAN_POINT ( 'NONE',  ( 111.9791666666666714, -7.950000000000001066, 2.130196079827424427 ) ) ;
#63183=( BOUNDED_CURVE ( )  B_SPLINE_CURVE ( 2, ( #8870, #108936, #53137, #31414, #9625, #21240, #33580, #100936, #45179, #56777, #123450, #98782, #124125 ),
 .UNSPECIFIED., .F., .T. ) 
 B_SPLINE_CURVE_WITH_KNOTS ( ( 3, 2, 2, 2, 2, 2, 3 ),
 ( 0.4500000000000001221, 0.4527777777777778900, 0.4555555555555556024, 0.4583333333333333703, 0.4611111111111111938, 0.4638888888888889062, 0.4666666666666666741 ),
 .UNSPECIFIED. ) 
 CURVE ( )  GEOMETRIC_REPRESENTATION_ITEM ( )  RATIONAL_B_SPLINE_CURVE ( ( 0.9999999999999986677, 0.9659258262890696445, 1.000000000000000000, 0.9659258262890683122, 1.000000000000000000, 0.9659258262890683122, 1.000000000000000000, 0.9659258262890683122, 1.000000000000000000, 0.9659258262890683122, 1.000000000000000000, 0.9659258262890683122, 1.000000000000000000 ) ) 
 REPRESENTATION_ITEM ( '' )  );
#63189=CARTESIAN_POINT ( 'NONE',  ( 101.3545968585647614, -1.637169565754161615, 6.110000000000000320 ) ) ;
#63199=CARTESIAN_POINT ( 'NONE',  ( 29.82919371712955581, -3.975000000000001865, 6.884901960086284411 ) ) ;
#63203=CARTESIAN_POINT ( 'NONE',  ( 28.70833333333332149, -3.974999999999999201, -6.884901960086287964 ) ) ;
#63215=CARTESIAN_POINT ( 'NONE',  ( 126.3495968585647944, 6.109999999999996767, 1.637169565754163836 ) ) ;
#63229=CARTESIAN_POINT ( 'NONE',  ( 48.85459685856476142, -1.637169565754161615, 6.110000000000000320 ) ) ;
#63236=CARTESIAN_POINT ( 'NONE',  ( 37.82876352523144448, 0.000000000000000000, -6.109999999999998543 ) ) ;
#63246=CARTESIAN_POINT ( 'NONE',  ( 79.99586038379621300, -3.974999999999998312, -6.884901960086286188 ) ) ;
#63266=CARTESIAN_POINT ( 'NONE',  ( 55.32876352523144448, 0.000000000000000000, -6.109999999999998543 ) ) ;
#63290=CARTESIAN_POINT ( 'NONE',  ( 55.78752705046288440, 0.000000000000000000, -7.949999999999998401 ) ) ;
#63300=CARTESIAN_POINT ( 'NONE',  ( 117.1620968585647802, -5.291415217122919401, 3.054999999999998384 ) ) ;
#63339=CARTESIAN_POINT ( 'NONE',  ( 34.91209685856478018, 5.291415217122922066, -3.054999999999995275 ) ) ;
#63357=CARTESIAN_POINT ( 'NONE',  ( 82.37500000000000000, 7.950000000000000178, 1.460391307983218535E-15 ) ) ;
#63359=ORIENTED_EDGE ( 'NONE', *, *, #69348, .F. ) ;
#63365=CARTESIAN_POINT ( 'NONE',  ( 104.2041937171295700, -6.884901960086285300, -3.975000000000000089 ) ) ;
#63367=CARTESIAN_POINT ( 'NONE',  ( 58.70419371712954870, -6.884901960086285300, -3.975000000000000089 ) ) ;
#63372=CARTESIAN_POINT ( 'NONE',  ( 51.45833333333332860, 3.974999999999997424, 6.884901960086288852 ) ) ;
#63379=CARTESIAN_POINT ( 'NONE',  ( 50.45876352523143282, 0.000000000000000000, -6.110000000000001208 ) ) ;
#63404=CARTESIAN_POINT ( 'NONE',  ( 65.53709685856478018, -3.054999999999998828, -5.291415217122919401 ) ) ;
#63406=EDGE_CURVE ( 'NONE', #49442, #129167, #18030, .T. ) ;
#63435=CARTESIAN_POINT ( 'NONE',  ( 87.55793019189812298, 6.110000000000000320, -1.637169565754156064 ) ) ;
#63442=EDGE_CURVE ( 'NONE', #33782, #942, #77331, .T. ) ;
#63459=CARTESIAN_POINT ( 'NONE',  ( 38.35459685856476852, -1.637169565754161615, 6.110000000000000320 ) ) ;
#63480=CARTESIAN_POINT ( 'NONE',  ( 108.8708603837962272, 6.884901960086289741, -3.974999999999993427 ) ) ;
#63510=CARTESIAN_POINT ( 'NONE',  ( 61.74543019189811588, -5.291415217122919401, -3.055000000000000604 ) ) ;
#63512=CARTESIAN_POINT ( 'NONE',  ( 73.43336038379621300, 2.130196079827431532, -7.949999999999996625 ) ) ;
#63537=CARTESIAN_POINT ( 'NONE',  ( 84.22502705046287019, 5.819803920172573086, -5.819803920172572198 ) ) ;
#63551=CARTESIAN_POINT ( 'NONE',  ( 76.27126352523144703, 4.472830434245839371, 4.472830434245842035 ) ) ;
#63559=FACE_OUTER_BOUND ( 'NONE', #22572, .T. ) ;
#63571=CARTESIAN_POINT ( 'NONE',  ( 75.10459685856474721, 1.637169565754164946, -6.109999999999999432 ) ) ;
#63594=CARTESIAN_POINT ( 'NONE',  ( 127.1386022459138019, -7.776507174585692163E-16, 6.349999999999999645 ) ) ;
#63616=CARTESIAN_POINT ( 'NONE',  ( 51.60416666666665009, 2.130196079827498146, 7.949999999999958433 ) ) ;
#63623=CARTESIAN_POINT ( 'NONE',  ( 66.93793019189810423, -6.110000000000001208, 1.637169565754158951 ) ) ;
#63630=CARTESIAN_POINT ( 'NONE',  ( 99.45876352523144703, 0.000000000000000000, -6.110000000000001208 ) ) ;
#63634=CARTESIAN_POINT ( 'NONE',  ( 56.99999999999999289, 0.000000000000000000, -7.950000000000000178 ) ) ;
#63652=AXIS2_PLACEMENT_3D ( 'NONE', #38830, #26523, #139602 ) ;
#63670=CARTESIAN_POINT ( 'NONE',  ( 0.000000000000000000, 0.000000000000000000, 0.000000000000000000 ) ) ;
#63671=CARTESIAN_POINT ( 'NONE',  ( 25.37543019189810067, -5.291415217122920289, -3.055000000000001492 ) ) ;
#63690=CARTESIAN_POINT ( 'NONE',  ( 118.0583603837962130, -7.949999999999997513, -2.130196079827425759 ) ) ;
#63718=CARTESIAN_POINT ( 'NONE',  ( 69.68750000000000000, -5.819803920172573974, 5.819803920172573086 ) ) ;
#63727=CARTESIAN_POINT ( 'NONE',  ( 103.9795968585647756, 6.109999999999999432, 1.637169565754164280 ) ) ;
#63736=CARTESIAN_POINT ( 'NONE',  ( 49.12500000000000000, -7.950000000000000178, -4.867971026610729436E-16 ) ) ;
#63737=CARTESIAN_POINT ( 'NONE',  ( 91.78709685856478018, 3.054999999999997495, 5.291415217122919401 ) ) ;
#63739=ORIENTED_EDGE ( 'NONE', *, *, #3223, .T. ) ;
#63771=CARTESIAN_POINT ( 'NONE',  ( 37.31250000000000000, 5.819803920172571310, 5.819803920172576639 ) ) ;
#63785=CARTESIAN_POINT ( 'NONE',  ( 31.70376352523145158, 6.109999999999998543, 1.122388791418548911E-15 ) ) ;
#63817=CARTESIAN_POINT ( 'NONE',  ( 90.03709685856478018, -3.054999999999999272, -5.291415217122919401 ) ) ;
#63841=ORIENTED_EDGE ( 'NONE', *, *, #93484, .T. ) ;
#63871=CARTESIAN_POINT ( 'NONE',  ( 107.6041666666666572, 2.130196079827422206, 7.950000000000001954 ) ) ;
#63882=CARTESIAN_POINT ( 'NONE',  ( 102.9587635252314470, 0.000000000000000000, -6.110000000000001208 ) ) ;
#63890=CARTESIAN_POINT ( 'NONE',  ( 32.45419371712955581, 6.884901960086283523, 3.975000000000002753 ) ) ;
#63894=CARTESIAN_POINT ( 'NONE',  ( 30.89583333333332860, -2.130196079827427091, 7.949999999999999289 ) ) ;
#63902=CARTESIAN_POINT ( 'NONE',  ( 126.2037635252314658, 6.109999999999998543, 1.122388791418548911E-15 ) ) ;
#63911=CARTESIAN_POINT ( 'NONE',  ( 48.12543019189810423, 5.291415217122919401, 3.055000000000002824 ) ) ;
#63917=CARTESIAN_POINT ( 'NONE',  ( 40.89126352523144448, -4.472830434245839371, -4.472830434245839371 ) ) ;
#63944=VERTEX_POINT ( 'NONE', #121734 ) ;
#63948=CARTESIAN_POINT ( 'NONE',  ( 56.64126352523144448, 4.472830434245835818, 4.472830434245840259 ) ) ;
#63965=ORIENTED_EDGE ( 'NONE', *, *, #71408, .F. ) ;
#63979=CARTESIAN_POINT ( 'NONE',  ( 122.4120968585647802, 5.291415217122922066, -3.054999999999995275 ) ) ;
#63986=CARTESIAN_POINT ( 'NONE',  ( 67.30836038379622721, 7.949999999999996625, 2.130196079827431088 ) ) ;
#63990=CARTESIAN_POINT ( 'NONE',  ( 43.00000000000000000, 0.000000000000000000, -7.950000000000000178 ) ) ;
#64000=FACE_OUTER_BOUND ( 'NONE', #125416, .T. ) ;
#64022=CARTESIAN_POINT ( 'NONE',  ( 41.91209685856478728, 5.291415217122922066, -3.054999999999995275 ) ) ;
#64046=CIRCLE ( 'NONE', #8414, 4.749999999999997335 ) ;
#64047=CARTESIAN_POINT ( 'NONE',  ( 52.87086038379622011, 6.884901960086289741, -3.974999999999993427 ) ) ;
#64052=CARTESIAN_POINT ( 'NONE',  ( 50.29166666666666430, 3.975000000000003642, -6.884901960086285300 ) ) ;
#64060=CARTESIAN_POINT ( 'NONE',  ( 51.47959685856477563, 6.109999999999999432, 1.637169565754164280 ) ) ;
#64066=CARTESIAN_POINT ( 'NONE',  ( 81.30836038379622721, 7.949999999999996625, 2.130196079827431088 ) ) ;
#64074=CARTESIAN_POINT ( 'NONE',  ( 87.06293019189809002, 1.637169565754157174, 6.110000000000002984 ) ) ;
#64081=CARTESIAN_POINT ( 'NONE',  ( 64.51626352523143737, -4.472830434245839371, 4.472830434245839371 ) ) ;
#64092=DIRECTION ( 'NONE',  ( -1.000000000000000000, -0.000000000000000000, -0.000000000000000000 ) ) ;
#64113=CARTESIAN_POINT ( 'NONE',  ( 88.14126352523143737, 4.472830434245835818, 4.472830434245840259 ) ) ;
#64122=ADVANCED_FACE ( 'NONE', ( #58703 ), #39026, .T. ) ;
#64142=CARTESIAN_POINT ( 'NONE',  ( 33.10459685856476852, 1.637169565754164946, -6.109999999999999432 ) ) ;
#64165=CARTESIAN_POINT ( 'NONE',  ( 110.0375270504628986, -9.735942053221456900E-16, 7.949999999999998401 ) ) ;
#64178=CARTESIAN_POINT ( 'NONE',  ( 96.03752705046289861, -9.735942053221456900E-16, 7.949999999999998401 ) ) ;
#64196=CARTESIAN_POINT ( 'NONE',  ( 64.95376352523145158, -6.109999999999999432, -3.741295971395163529E-16 ) ) ;
#64221=CARTESIAN_POINT ( 'NONE',  ( 80.28752705046289861, 0.000000000000000000, -7.949999999999998401 ) ) ;
#64233=CARTESIAN_POINT ( 'NONE',  ( 73.79209685856477563, -5.291415217122921177, 3.054999999999999272 ) ) ;
#64254=CARTESIAN_POINT ( 'NONE',  ( 68.68793019189809002, 6.110000000000002984, -1.637169565754156730 ) ) ;
#64273=CARTESIAN_POINT ( 'NONE',  ( 128.7427689125804591, -1.701477371937628824, -6.349999999999999645 ) ) ;
#64282=CARTESIAN_POINT ( 'NONE',  ( 116.4329301918981088, 1.637169565754156508, 6.110000000000000320 ) ) ;
#64308=EDGE_CURVE ( 'NONE', #10128, #2613, #92089, .T. ) ;
#64310=CARTESIAN_POINT ( 'NONE',  ( 67.95876352523144703, 0.000000000000000000, -6.110000000000001208 ) ) ;
#64316=CARTESIAN_POINT ( 'NONE',  ( 99.02126352523143282, -4.472830434245838482, -4.472830434245840259 ) ) ;
#64323=CARTESIAN_POINT ( 'NONE',  ( 91.56249999999998579, -5.819803920172573086, -5.819803920172573974 ) ) ;
#64325=ORIENTED_EDGE ( 'NONE', *, *, #135623, .T. ) ;
#64327=CARTESIAN_POINT ( 'NONE',  ( 109.5000000000000000, 0.000000000000000000, -7.950000000000000178 ) ) ;
#64332=CARTESIAN_POINT ( 'NONE',  ( 119.6412635252314516, 4.472830434245835818, 4.472830434245840259 ) ) ;
#64346=CARTESIAN_POINT ( 'NONE',  ( 37.89583333333332149, -2.130196079827351596, 7.950000000000043698 ) ) ;
#64357=CARTESIAN_POINT ( 'NONE',  ( 33.97959685856477563, 6.109999999999999432, 1.637169565754164280 ) ) ;
#64376=ORIENTED_EDGE ( 'NONE', *, *, #74463, .F. ) ;
#64378=CARTESIAN_POINT ( 'NONE',  ( 112.6625270504628986, 7.949999999999998401, 1.460391307983218338E-15 ) ) ;
#64394=CARTESIAN_POINT ( 'NONE',  ( 92.53752705046289861, -9.735942053221456900E-16, 7.949999999999998401 ) ) ;
#64400=CARTESIAN_POINT ( 'NONE',  ( 93.60416666666665719, 2.130196079827422206, 7.950000000000001954 ) ) ;
#64406=CARTESIAN_POINT ( 'NONE',  ( 69.25000000000000000, -9.735942053221458872E-16, 7.950000000000000178 ) ) ;
#64413=CARTESIAN_POINT ( 'NONE',  ( 99.75043019189810423, 3.055000000000002824, -5.291415217122919401 ) ) ;
#64422=CARTESIAN_POINT ( 'NONE',  ( 94.12043019189810877, 3.055000000000001936, -5.291415217122916737 ) ) ;
#64455=CARTESIAN_POINT ( 'NONE',  ( 56.56250000000000000, -5.819803920172573086, -5.819803920172573974 ) ) ;
#64478=CARTESIAN_POINT ( 'NONE',  ( 29.22459685856478373, -1.637169565754160949, 6.109999999999997655 ) ) ;
#64493=EDGE_CURVE ( 'NONE', #129366, #37814, #121721, .T. ) ;
#64512=CARTESIAN_POINT ( 'NONE',  ( 93.97459685856478018, 1.637169565754164280, -6.109999999999997655 ) ) ;
#64530=AXIS2_PLACEMENT_3D ( 'NONE', #10064, #124550, #89085 ) ;
#64562=CARTESIAN_POINT ( 'NONE',  ( 99.14583333333331439, 2.130196079827431976, -7.949999999999999289 ) ) ;
#64565=EDGE_LOOP ( 'NONE', ( #56870, #83095, #95121, #129348 ) ) ;
#64577=CARTESIAN_POINT ( 'NONE',  ( 108.0629301918980900, 1.637169565754157174, 6.110000000000002984 ) ) ;
#64588=CARTESIAN_POINT ( 'NONE',  ( 32.89169371712954870, 2.130196079827421762, 7.950000000000001066 ) ) ;
#64592=CARTESIAN_POINT ( 'NONE',  ( 31.33333333333332504, -6.884901960086287964, 3.974999999999998312 ) ) ;
#64603=CARTESIAN_POINT ( 'NONE',  ( 119.0579301918981230, 6.110000000000000320, -1.637169565754156064 ) ) ;
#64611=CARTESIAN_POINT ( 'NONE',  ( 44.62543019189810423, 5.291415217122919401, 3.055000000000002824 ) ) ;
#64616=CARTESIAN_POINT ( 'NONE',  ( 35.34959685856478728, 6.109999999999996767, 1.637169565754163836 ) ) ;
#64622=VERTEX_POINT ( 'NONE', #19946 ) ;
#64627=CARTESIAN_POINT ( 'NONE',  ( 79.26669371712955581, -7.949999999999998401, 2.130196079827423983 ) ) ;
#64652=CARTESIAN_POINT ( 'NONE',  ( 53.28709685856478018, 3.054999999999997495, 5.291415217122919401 ) ) ;
#64663=EDGE_CURVE ( 'NONE', #82847, #93164, #86624, .T. ) ;
#64672=ORIENTED_EDGE ( 'NONE', *, *, #87360, .T. ) ;
#64695=CARTESIAN_POINT ( 'NONE',  ( 118.6204301918981230, 3.055000000000002380, -5.291415217122917625 ) ) ;
#64704=DIRECTION ( 'NONE',  ( 1.000000000000000000, 0.000000000000000000, 0.000000000000000000 ) ) ;
#64727=CARTESIAN_POINT ( 'NONE',  ( 38.70376352523144448, 6.109999999999999432, 1.122388791418549108E-15 ) ) ;
#64759=CARTESIAN_POINT ( 'NONE',  ( 60.30836038379622011, 7.949999999999997513, 2.130196079827431088 ) ) ;
#64765=CARTESIAN_POINT ( 'NONE',  ( 51.31249999999998579, 5.819803920172571310, 5.819803920172575751 ) ) ;
#64777=CARTESIAN_POINT ( 'NONE',  ( 50.16709685856476852, -3.055000000000000160, -5.291415217122921177 ) ) ;
#64794=CARTESIAN_POINT ( 'NONE',  ( 81.66709685856477563, -3.055000000000000160, -5.291415217122921177 ) ) ;
#64804=CARTESIAN_POINT ( 'NONE',  ( 66.41209685856478018, 5.291415217122921177, -3.054999999999994831 ) ) ;
#64829=CARTESIAN_POINT ( 'NONE',  ( 1.500000000000000000, 0.000000000000000000, 0.000000000000000000 ) ) ;
#64834=CARTESIAN_POINT ( 'NONE',  ( 80.70376352523145158, 6.109999999999998543, 1.122388791418548911E-15 ) ) ;
#64863=CARTESIAN_POINT ( 'NONE',  ( 39.66709685856477563, -3.055000000000000160, -5.291415217122921177 ) ) ;
#64911=CARTESIAN_POINT ( 'NONE',  ( 111.9791666666666714, -7.950000000000000178, 2.130196079827424427 ) ) ;
#64915=CARTESIAN_POINT ( 'NONE',  ( 69.03709685856478018, -3.054999999999999272, -5.291415217122919401 ) ) ;
#64918=CARTESIAN_POINT ( 'NONE',  ( 84.41666666666667140, -6.884901960086287076, -3.975000000000000977 ) ) ;
#64928=ORIENTED_EDGE ( 'NONE', *, *, #136460, .T. ) ;
#64942=CARTESIAN_POINT ( 'NONE',  ( 85.68336038379624142, -2.130196079827426203, 7.949999999999997513 ) ) ;
#64948=CARTESIAN_POINT ( 'NONE',  ( 83.24999999999998579, -9.735942053221458872E-16, 7.950000000000000178 ) ) ;
#64961=CARTESIAN_POINT ( 'NONE',  ( 76.56293019189810423, 1.637169565754157174, 6.110000000000002984 ) ) ;
#64984=CARTESIAN_POINT ( 'NONE',  ( 61.39626352523143993, 4.472830434245840259, -4.472830434245839371 ) ) ;
#65016=CARTESIAN_POINT ( 'NONE',  ( 110.1620968585647944, -5.291415217122919401, 3.054999999999997939 ) ) ;
#65021=CARTESIAN_POINT ( 'NONE',  ( 25.08376352523143638, -6.110000000000001208, -3.741295971395164515E-16 ) ) ;
#65027=CARTESIAN_POINT ( 'NONE',  ( 58.85002705046289151, -5.819803920172573086, -5.819803920172573086 ) ) ;
#65033=CARTESIAN_POINT ( 'NONE',  ( 50.43749999999999289, 5.819803920172574863, -5.819803920172573086 ) ) ;
#65038=CARTESIAN_POINT ( 'NONE',  ( 66.50043019189810423, -3.055000000000002380, 5.291415217122920289 ) ) ;
#65045=CARTESIAN_POINT ( 'NONE',  ( 96.54209685856477563, 5.291415217122923842, -3.054999999999996163 ) ) ;
#65061=ORIENTED_EDGE ( 'NONE', *, *, #130157, .F. ) ;
#65064=CARTESIAN_POINT ( 'NONE',  ( 118.7662635252314516, 4.472830434245838482, -4.472830434245837594 ) ) ;
#65093=CARTESIAN_POINT ( 'NONE',  ( 26.25043019189810067, 3.055000000000002824, -5.291415217122919401 ) ) ;
#65115=CARTESIAN_POINT ( 'NONE',  ( 114.2666937171295700, -7.949999999999999289, 2.130196079827424427 ) ) ;
#65117=CARTESIAN_POINT ( 'NONE',  ( 49.07919371712955581, 3.975000000000002753, -6.884901960086283523 ) ) ;
#65128=DIRECTION ( 'NONE',  ( -1.000000000000000000, -0.000000000000000000, -0.000000000000000000 ) ) ;
#65149=CARTESIAN_POINT ( 'NONE',  ( 95.50000000000000000, 0.000000000000000000, -7.950000000000000178 ) ) ;
#65159=CARTESIAN_POINT ( 'NONE',  ( 93.18793019189809002, 6.110000000000002984, -1.637169565754156730 ) ) ;
#65162=CARTESIAN_POINT ( 'NONE',  ( 85.53752705046288440, -9.735942053221456900E-16, 7.949999999999998401 ) ) ;
#65169=CARTESIAN_POINT ( 'NONE',  ( 89.89126352523143737, -4.472830434245839371, -4.472830434245839371 ) ) ;
#65184=CYLINDRICAL_SURFACE ( 'NONE', #22493, 7.950000000000000178 ) ;
#65199=PLANE ( 'NONE',  #64530 ) ;
#65206=CARTESIAN_POINT ( 'NONE',  ( 119.1250000000000142, -7.950000000000000178, -4.867971026610729436E-16 ) ) ;
#65224=CARTESIAN_POINT ( 'NONE',  ( 125.5629301918981042, 1.637169565754157174, 6.110000000000002984 ) ) ;
#65256=CARTESIAN_POINT ( 'NONE',  ( 91.64126352523143737, 4.472830434245837594, 4.472830434245841147 ) ) ;
#65288=ORIENTED_EDGE ( 'NONE', *, *, #55111, .F. ) ;
#65310=CARTESIAN_POINT ( 'NONE',  ( 105.2708333333333286, -7.949999999999999289, -2.130196079827426203 ) ) ;
#65313=ORIENTED_EDGE ( 'NONE', *, *, #69348, .T. ) ;
#65317=CARTESIAN_POINT ( 'NONE',  ( 89.52083333333332860, 7.949999999999998401, 2.130196079827431532 ) ) ;
#65334=CARTESIAN_POINT ( 'NONE',  ( 29.68336038379622366, -2.130196079827426203, 7.949999999999997513 ) ) ;
#65339=CARTESIAN_POINT ( 'NONE',  ( 121.3337635252314328, 6.110000000000001208, 1.122388791418549305E-15 ) ) ;
#65350=CARTESIAN_POINT ( 'NONE',  ( 124.0162635252314658, -4.472830434245839371, 4.472830434245839371 ) ) ;
#65358=CARTESIAN_POINT ( 'NONE',  ( 42.43793019189809712, -6.110000000000001208, 1.637169565754158951 ) ) ;
#65366=CARTESIAN_POINT ( 'NONE',  ( 37.39126352523143737, -4.472830434245839371, -4.472830434245839371 ) ) ;
#65397=CARTESIAN_POINT ( 'NONE',  ( 44.82876352523145158, 0.000000000000000000, -6.109999999999998543 ) ) ;
#65404=CIRCLE ( 'NONE', #137210, 6.349999999999997868 ) ;
#65420=CARTESIAN_POINT ( 'NONE',  ( 0.000000000000000000, 0.000000000000000000, 0.000000000000000000 ) ) ;
#65431=CARTESIAN_POINT ( 'NONE',  ( 118.3287635252314658, 0.000000000000000000, -6.109999999999999432 ) ) ;
#65441=EDGE_LOOP ( 'NONE', ( #85850, #65061, #107955 ) ) ;
#65445=EDGE_CURVE ( 'NONE', #55968, #91497, #140490, .T. ) ;
#65473=CARTESIAN_POINT ( 'NONE',  ( 38.26626352523144448, 4.472830434245839371, -4.472830434245839371 ) ) ;
#65493=CARTESIAN_POINT ( 'NONE',  ( 83.24999999999998579, -9.735942053221458872E-16, 7.950000000000000178 ) ) ;
#65502=CARTESIAN_POINT ( 'NONE',  ( 20.65000000000000213, 7.776507174585702024E-16, -6.350000000000008527 ) ) ;
#65504=CARTESIAN_POINT ( 'NONE',  ( 55.35002705046288440, -5.819803920172572198, -5.819803920172572198 ) ) ;
#65512=CARTESIAN_POINT ( 'NONE',  ( 49.27083333333333570, -7.949999999999999289, -2.130196079827426203 ) ) ;
#65521=CARTESIAN_POINT ( 'NONE',  ( 47.97959685856477563, 6.109999999999999432, 1.637169565754164280 ) ) ;
#65538=CARTESIAN_POINT ( 'NONE',  ( 78.75043019189810423, 3.055000000000002824, -5.291415217122919401 ) ) ;
#65543=CARTESIAN_POINT ( 'NONE',  ( 0.000000000000000000, 0.000000000000000000, 7.950000000000000178 ) ) ;
#65548=CARTESIAN_POINT ( 'NONE',  ( 87.87086038379622721, 6.884901960086289741, -3.974999999999993427 ) ) ;
#65549=CARTESIAN_POINT ( 'NONE',  ( 67.72459685856478018, -1.637169565754160949, 6.109999999999997655 ) ) ;
#65570=CARTESIAN_POINT ( 'NONE',  ( 41.64169371712954870, -2.130196079827424871, -7.949999999999998401 ) ) ;
#65573=CARTESIAN_POINT ( 'NONE',  ( 51.26669371712954870, -7.949999999999998401, 2.130196079827423983 ) ) ;
#65579=CARTESIAN_POINT ( 'NONE',  ( 89.01626352523143737, -4.472830434245838482, 4.472830434245838482 ) ) ;
#65588=LINE ( 'NONE', #98180, #56448 ) ;
#65606=CARTESIAN_POINT ( 'NONE',  ( 32.95876352523143282, 0.000000000000000000, -6.110000000000001208 ) ) ;
#65610=EDGE_CURVE ( 'NONE', #53682, #71447, #12498, .T. ) ;
#65615=ORIENTED_EDGE ( 'NONE', *, *, #99361, .T. ) ;
#65624=CARTESIAN_POINT ( 'NONE',  ( 113.5375270504628986, -9.735942053221456900E-16, 7.949999999999998401 ) ) ;
#65666=CARTESIAN_POINT ( 'NONE',  ( 63.49543019189811588, 5.291415217122917625, 3.055000000000002380 ) ) ;
#65691=CARTESIAN_POINT ( 'NONE',  ( 83.78752705046288440, 0.000000000000000000, -7.949999999999998401 ) ) ;
#65696=CARTESIAN_POINT ( 'NONE',  ( 86.89583333333332860, -2.130196079827427091, 7.949999999999999289 ) ) ;
#65698=DIRECTION ( 'NONE',  ( -1.000000000000000000, -0.000000000000000000, -0.000000000000000000 ) ) ;
#65706=CARTESIAN_POINT ( 'NONE',  ( 75.68793019189811844, 6.110000000000002984, -1.637169565754156730 ) ) ;
#65725=CARTESIAN_POINT ( 'NONE',  ( 65.33376352523143282, 6.110000000000001208, 1.122388791418549305E-15 ) ) ;
#65755=CARTESIAN_POINT ( 'NONE',  ( 117.3079301918980946, -6.109999999999998543, 1.637169565754158507 ) ) ;
#65782=CARTESIAN_POINT ( 'NONE',  ( 61.83376352523143993, 6.110000000000001208, 1.122388791418549305E-15 ) ) ;
#65789=CARTESIAN_POINT ( 'NONE',  ( 99.60459685856476142, 1.637169565754164946, -6.109999999999999432 ) ) ;
#65804=CARTESIAN_POINT ( 'NONE',  ( 118.6204301918981230, 3.055000000000001936, -5.291415217122916737 ) ) ;
#65829=CARTESIAN_POINT ( 'NONE',  ( 33.39626352523143993, 4.472830434245840259, -4.472830434245839371 ) ) ;
#65832=EDGE_CURVE ( 'NONE', #139700, #49576, #27311, .T. ) ;
#65836=CARTESIAN_POINT ( 'NONE',  ( 0.000000000000000000, 0.000000000000000000, 0.000000000000000000 ) ) ;
#65850=ADVANCED_FACE ( 'NONE', ( #122136 ), #68519, .T. ) ;
#65853=CARTESIAN_POINT ( 'NONE',  ( 107.9958603837962272, -3.974999999999998312, -6.884901960086286188 ) ) ;
#65880=CARTESIAN_POINT ( 'NONE',  ( 69.97916666666665719, -7.950000000000000178, 2.130196079827424427 ) ) ;
#65887=CARTESIAN_POINT ( 'NONE',  ( 89.10459685856477563, 1.637169565754164946, -6.109999999999999432 ) ) ;
#65896=CARTESIAN_POINT ( 'NONE',  ( 85.80793019189810877, -6.109999999999998543, 1.637169565754158063 ) ) ;
#65921=CARTESIAN_POINT ( 'NONE',  ( 56.70833333333333570, -3.974999999999999201, -6.884901960086287964 ) ) ;
#65931=CARTESIAN_POINT ( 'NONE',  ( 116.8916937171295558, 2.130196079827421762, 7.950000000000000178 ) ) ;
#65935=ORIENTED_EDGE ( 'NONE', *, *, #26965, .T. ) ;
#65945=LINE ( 'NONE', #143454, #124805 ) ;
#65948=CARTESIAN_POINT ( 'NONE',  ( 126.4379301918981184, -6.110000000000001208, 1.637169565754158951 ) ) ;
#65978=CARTESIAN_POINT ( 'NONE',  ( 83.32876352523143737, 0.000000000000000000, -6.109999999999999432 ) ) ;
#65979=CARTESIAN_POINT ( 'NONE',  ( 6.092757112198636804, -9.434971466833395937, -1.145375144610985441 ) ) ;
#66022=CARTESIAN_POINT ( 'NONE',  ( 103.5208333333333428, 7.949999999999999289, 2.130196079827431532 ) ) ;
#66029=CARTESIAN_POINT ( 'NONE',  ( 90.25000000000000000, -9.735942053221458872E-16, 7.950000000000000178 ) ) ;
#66048=CARTESIAN_POINT ( 'NONE',  ( 116.0837635252314470, -6.110000000000001208, -3.741295971395164515E-16 ) ) ;
#66057=CARTESIAN_POINT ( 'NONE',  ( 118.0370968585647802, -3.054999999999998828, -5.291415217122919401 ) ) ;
#66064=ORIENTED_EDGE ( 'NONE', *, *, #59783, .F. ) ;
#66065=CARTESIAN_POINT ( 'NONE',  ( 37.91709685856477563, 3.054999999999998828, 5.291415217122922066 ) ) ;
#66071=CARTESIAN_POINT ( 'NONE',  ( 33.01626352523145158, -4.472830434245839371, 4.472830434245839371 ) ) ;
#66097=CARTESIAN_POINT ( 'NONE',  ( 46.43293019189811588, 1.637169565754156508, 6.110000000000000320 ) ) ;
#66108=( BOUNDED_CURVE ( )  B_SPLINE_CURVE ( 2, ( #127903, #62639, #60512, #18363, #72842, #16983, #82957, #48909, #103954, #74220, #93113, #71370, #105399 ),
 .UNSPECIFIED., .F., .F. ) 
 B_SPLINE_CURVE_WITH_KNOTS ( ( 3, 2, 2, 2, 2, 2, 3 ),
 ( 0.8833333333333334147, 0.8861111111111111827, 0.8888888888888889506, 0.8916666666666668295, 0.8944444444444445974, 0.8972222222222223653, 0.9000000000000001332 ),
 .UNSPECIFIED. ) 
 CURVE ( )  GEOMETRIC_REPRESENTATION_ITEM ( )  RATIONAL_B_SPLINE_CURVE ( ( 0.9999999999999986677, 0.9659258262890696445, 1.000000000000000000, 0.9659258262890683122, 1.000000000000000000, 0.9659258262890683122, 1.000000000000000000, 0.9659258262890683122, 1.000000000000000000, 0.9659258262890683122, 1.000000000000000000, 0.9659258262890669799, 1.000000000000001332 ) ) 
 REPRESENTATION_ITEM ( '' )  );
#66136=CARTESIAN_POINT ( 'NONE',  ( 124.3079301918981230, -6.109999999999999432, 1.637169565754158507 ) ) ;
#66173=CARTESIAN_POINT ( 'NONE',  ( 29.07876352523144803, -7.482591942790327058E-16, 6.109999999999999432 ) ) ;
#66188=CARTESIAN_POINT ( 'NONE',  ( 126.7295968585647614, -6.110000000000000320, -1.637169565754161393 ) ) ;
#66198=CARTESIAN_POINT ( 'NONE',  ( 51.99586038379622011, -3.974999999999998312, -6.884901960086286188 ) ) ;
#66204=CARTESIAN_POINT ( 'NONE',  ( 43.43749999999998579, 5.819803920172573974, -5.819803920172572198 ) ) ;
#66211=CARTESIAN_POINT ( 'NONE',  ( 33.54209685856476852, 5.291415217122923842, -3.054999999999996163 ) ) ;
#66227=CARTESIAN_POINT ( 'NONE',  ( 84.29209685856477563, -5.291415217122921177, 3.054999999999999272 ) ) ;
#66237=CARTESIAN_POINT ( 'NONE',  ( 71.07876352523146579, -7.482591942790325086E-16, 6.109999999999998543 ) ) ;
#66245=( NAMED_UNIT ( * ) PLANE_ANGLE_UNIT ( ) SI_UNIT ( $, .RADIAN. ) );
#66265=CARTESIAN_POINT ( 'NONE',  ( 72.82876352523145158, 0.000000000000000000, -6.109999999999998543 ) ) ;
#66284=VERTEX_POINT ( 'NONE', #111074 ) ;
#66294=( BOUNDED_CURVE ( )  B_SPLINE_CURVE ( 2, ( #38527, #27631, #93625, #114637, #104479, #3705, #69029, #50126, #59587, #103748, #49436, #103072, #82752 ),
 .UNSPECIFIED., .F., .T. ) 
 B_SPLINE_CURVE_WITH_KNOTS ( ( 3, 2, 2, 2, 2, 2, 3 ),
 ( 0.9499999999999999556, 0.9527777777777777235, 0.9555555555555556024, 0.9583333333333333703, 0.9611111111111111382, 0.9638888888888889062, 0.9666666666666666741 ),
 .UNSPECIFIED. ) 
 CURVE ( )  GEOMETRIC_REPRESENTATION_ITEM ( )  RATIONAL_B_SPLINE_CURVE ( ( 1.000000000000000000, 0.9659258262890683122, 1.000000000000000000, 0.9659258262890683122, 1.000000000000000000, 0.9659258262890683122, 1.000000000000000000, 0.9659258262890683122, 1.000000000000000000, 0.9659258262890683122, 1.000000000000000000, 0.9659258262890683122, 1.000000000000000000 ) ) 
 REPRESENTATION_ITEM ( '' )  );
#66323=CARTESIAN_POINT ( 'NONE',  ( 129.0581452878471680, 0.000000000000000000, -7.029999999999999361 ) ) ;
#66339=EDGE_LOOP ( 'NONE', ( #113399, #65615, #28028, #132517 ) ) ;
#66348=CARTESIAN_POINT ( 'NONE',  ( 61.89126352523144448, -4.472830434245839371, -4.472830434245839371 ) ) ;
#66352=CARTESIAN_POINT ( 'NONE',  ( 83.24999999999998579, -9.735942053221458872E-16, 7.950000000000000178 ) ) ;
#66360=FACE_OUTER_BOUND ( 'NONE', #95721, .T. ) ;
#66365=CARTESIAN_POINT ( 'NONE',  ( 26.80526891258047328, -5.499261314031188341, -3.175000000000002487 ) ) ;
#66369=CARTESIAN_POINT ( 'NONE',  ( 82.03752705046288440, -9.735942053221456900E-16, 7.949999999999998401 ) ) ;
#66374=CARTESIAN_POINT ( 'NONE',  ( 69.97916666666665719, -7.950000000000001066, 2.130196079827424427 ) ) ;
#66383=CARTESIAN_POINT ( 'NONE',  ( 78.31293019189810423, -1.637169565754159617, -6.110000000000001208 ) ) ;
#66399=CARTESIAN_POINT ( 'NONE',  ( 77.12500000000000000, -7.950000000000000178, -4.867971026610729436E-16 ) ) ;
#66403=ORIENTED_EDGE ( 'NONE', *, *, #110521, .T. ) ;
#66404=CARTESIAN_POINT ( 'NONE',  ( 63.87543019189810423, -5.291415217122920289, -3.055000000000001492 ) ) ;
#66411=CARTESIAN_POINT ( 'NONE',  ( 125.4979281168462961, -3.948843003177505473, -6.900003709242945149 ) ) ;
#66417=EDGE_CURVE ( 'NONE', #75931, #128706, #50609, .T. ) ;
#66437=CARTESIAN_POINT ( 'NONE',  ( 100.2454301918981230, -5.291415217122918513, -3.055000000000000160 ) ) ;
#66450=DIRECTION ( 'NONE',  ( -1.000000000000000000, -0.000000000000000000, -0.000000000000000000 ) ) ;
#66458=CARTESIAN_POINT ( 'NONE',  ( 88.35416666666665719, -2.130196079827463507, -7.949999999999979750 ) ) ;
#66465=CARTESIAN_POINT ( 'NONE',  ( 54.25043019189811133, 3.055000000000002824, -5.291415217122919401 ) ) ;
#66471=CARTESIAN_POINT ( 'NONE',  ( 98.72959685856477563, -6.110000000000000320, -1.637169565754161393 ) ) ;
#66486=CARTESIAN_POINT ( 'NONE',  ( 120.5162635252314374, -4.472830434245838482, 4.472830434245838482 ) ) ;
#66488=DIRECTION ( 'NONE',  ( 0.000000000000000000, 0.000000000000000000, 1.000000000000000000 ) ) ;
#66532=CARTESIAN_POINT ( 'NONE',  ( 115.7250270504628702, 5.819803920172573086, -5.819803920172572198 ) ) ;
#66552=( BOUNDED_CURVE ( )  B_SPLINE_CURVE ( 2, ( #118611, #120750, #141071, #141823, #85993, #22141, #66399, #130951, #110569, #87434, #21457, #86723, #119314 ),
 .UNSPECIFIED., .F., .T. ) 
 B_SPLINE_CURVE_WITH_KNOTS ( ( 3, 2, 2, 2, 2, 2, 3 ),
 ( 0.4666666666666666741, 0.4694444444444444420, 0.4722222222222222099, 0.4749999999999999778, 0.4777777777777778012, 0.4805555555555555691, 0.4833333333333333370 ),
 .UNSPECIFIED. ) 
 CURVE ( )  GEOMETRIC_REPRESENTATION_ITEM ( )  RATIONAL_B_SPLINE_CURVE ( ( 1.000000000000000000, 0.9659258262890683122, 1.000000000000000000, 0.9659258262890683122, 1.000000000000000000, 0.9659258262890683122, 1.000000000000000000, 0.9659258262890683122, 1.000000000000000000, 0.9659258262890683122, 1.000000000000000000, 0.9659258262890683122, 1.000000000000000000 ) ) 
 REPRESENTATION_ITEM ( '' )  );
#66568=VERTEX_POINT ( 'NONE', #22281 ) ;
#66571=CARTESIAN_POINT ( 'NONE',  ( 88.52126352523143282, -4.472830434245839371, -4.472830434245840259 ) ) ;
#66584=CARTESIAN_POINT ( 'NONE',  ( 88.43293019189809456, 1.637169565754156508, 6.110000000000000320 ) ) ;
#66635=CARTESIAN_POINT ( 'NONE',  ( 125.4170968585647756, 3.054999999999998828, 5.291415217122922066 ) ) ;
#66667=CARTESIAN_POINT ( 'NONE',  ( 82.30793019189809456, -6.109999999999999432, 1.637169565754158507 ) ) ;
#66711=CARTESIAN_POINT ( 'NONE',  ( 100.8958333333333144, -2.130196079827427091, 7.949999999999999289 ) ) ;
#66717=EDGE_LOOP ( 'NONE', ( #109012, #125487, #58824, #44944 ) ) ;
#66721=AXIS2_PLACEMENT_3D ( 'NONE', #4659, #38784, #72167 ) ;
#66731=CARTESIAN_POINT ( 'NONE',  ( 26.99999999999999645, 4.648385311654464225, 5.846484084903029732 ) ) ;
#66735=CARTESIAN_POINT ( 'NONE',  ( 86.99586038379622721, -3.974999999999998312, -6.884901960086286188 ) ) ;
#66741=CARTESIAN_POINT ( 'NONE',  ( 119.2920968585647756, -5.291415217122921177, 3.054999999999999272 ) ) ;
#66751=CARTESIAN_POINT ( 'NONE',  ( 118.1829301918981372, -1.637169565754158951, -6.109999999999998543 ) ) ;
#66761=CARTESIAN_POINT ( 'NONE',  ( 35.72959685856475431, -6.110000000000000320, -1.637169565754161393 ) ) ;
#66767=CARTESIAN_POINT ( 'NONE',  ( 27.32876352523144803, 0.000000000000000000, -6.109999999999998543 ) ) ;
#66795=CARTESIAN_POINT ( 'NONE',  ( 48.47459685856478018, 1.637169565754164280, -6.109999999999996767 ) ) ;
#66803=CARTESIAN_POINT ( 'NONE',  ( 71.53752705046289861, -9.735942053221456900E-16, 7.949999999999998401 ) ) ;
#66835=CARTESIAN_POINT ( 'NONE',  ( 111.7662635252314516, 4.472830434245839371, -4.472830434245839371 ) ) ;
#66858=ORIENTED_EDGE ( 'NONE', *, *, #15031, .T. ) ;
#66865=CARTESIAN_POINT ( 'NONE',  ( 0.000000000000000000, 0.000000000000000000, 7.950000000000000178 ) ) ;
#66877=CARTESIAN_POINT ( 'NONE',  ( 127.9750270504628702, -5.819803920172572198, 5.819803920172572198 ) ) ;
#66891=CARTESIAN_POINT ( 'NONE',  ( 119.7295968585647614, -6.110000000000000320, -1.637169565754161393 ) ) ;
#66900=CARTESIAN_POINT ( 'NONE',  ( 49.22502705046289151, 5.819803920172573086, -5.819803920172572198 ) ) ;
#66906=CARTESIAN_POINT ( 'NONE',  ( 46.79166666666666430, 3.975000000000003642, -6.884901960086285300 ) ) ;
#66915=CARTESIAN_POINT ( 'NONE',  ( 33.97959685856477563, 6.109999999999999432, 1.637169565754164280 ) ) ;
#66924=CARTESIAN_POINT ( 'NONE',  ( 81.16252705046289861, 7.949999999999998401, 1.460391307983218338E-15 ) ) ;
#66932=CARTESIAN_POINT ( 'NONE',  ( 80.06293019189807580, 1.637169565754157174, 6.110000000000002984 ) ) ;
#66940=CARTESIAN_POINT ( 'NONE',  ( 54.01626352523143737, -4.472830434245839371, 4.472830434245839371 ) ) ;
#66947=SURFACE_STYLE_USAGE ( .BOTH. , #77827 ) ;
#66974=CARTESIAN_POINT ( 'NONE',  ( 71.66209685856478018, -5.291415217122919401, 3.054999999999997939 ) ) ;
#66998=CARTESIAN_POINT ( 'NONE',  ( 27.70876352523143993, -7.482591942790329030E-16, 6.110000000000001208 ) ) ;
#67026=CARTESIAN_POINT ( 'NONE',  ( 0.000000000000000000, 0.000000000000000000, 0.000000000000000000 ) ) ;
#67046=CARTESIAN_POINT ( 'NONE',  ( 112.5624999999999858, -5.819803920172573086, -5.819803920172573974 ) ) ;
#67051=CARTESIAN_POINT ( 'NONE',  ( 58.53709685856478728, -3.054999999999999272, -5.291415217122919401 ) ) ;
#67056=CARTESIAN_POINT ( 'NONE',  ( 31.72502705046288796, 5.819803920172573974, -5.819803920172573086 ) ) ;
#67067=FACE_OUTER_BOUND ( 'NONE', #9457, .T. ) ;
#67077=CARTESIAN_POINT ( 'NONE',  ( 72.99586038379622721, -3.974999999999998312, -6.884901960086286188 ) ) ;
#67082=CARTESIAN_POINT ( 'NONE',  ( 73.77083333333331439, -7.949999999999999289, -2.130196079827426203 ) ) ;
#67094=CARTESIAN_POINT ( 'NONE',  ( 64.02126352523144703, -4.472830434245839371, -4.472830434245840259 ) ) ;
#67111=CARTESIAN_POINT ( 'NONE',  ( 64.31293019189810423, -1.637169565754159617, -6.110000000000001208 ) ) ;
#67129=ORIENTED_EDGE ( 'NONE', *, *, #129355, .F. ) ;
#67142=CARTESIAN_POINT ( 'NONE',  ( 103.1620968585647802, -5.291415217122919401, 3.054999999999997939 ) ) ;
#67166=CARTESIAN_POINT ( 'NONE',  ( 51.47959685856477563, 6.109999999999999432, 1.637169565754164280 ) ) ;
#67172=CARTESIAN_POINT ( 'NONE',  ( 90.27126352523143282, 4.472830434245838482, 4.472830434245842035 ) ) ;
#67174=EDGE_CURVE ( 'NONE', #13015, #121255, #120011, .T. ) ;
#67189=CARTESIAN_POINT ( 'NONE',  ( 118.9120968585647802, 5.291415217122921177, -3.054999999999994831 ) ) ;
#67211=CARTESIAN_POINT ( 'NONE',  ( 6.093288859525676671, 9.434732237030869939, -1.147367193843239930 ) ) ;
#67240=CARTESIAN_POINT ( 'NONE',  ( 112.0791937171295558, 3.975000000000002753, -6.884901960086283523 ) ) ;
#67260=CARTESIAN_POINT ( 'NONE',  ( 89.97959685856477563, 6.109999999999999432, 1.637169565754164280 ) ) ;
#67274=ADVANCED_FACE ( 'NONE', ( #71231 ), #6607, .T. ) ;
#67277=ORIENTED_EDGE ( 'NONE', *, *, #74104, .T. ) ;
#67279=CARTESIAN_POINT ( 'NONE',  ( 101.7250270504628986, 5.819803920172573974, -5.819803920172573086 ) ) ;
#67286=CARTESIAN_POINT ( 'NONE',  ( 92.02126352523143282, -4.472830434245839371, -4.472830434245840259 ) ) ;
#67301=CARTESIAN_POINT ( 'NONE',  ( 89.30793019189809456, -6.109999999999998543, 1.637169565754158063 ) ) ;
#67335=CARTESIAN_POINT ( 'NONE',  ( 0.000000000000000000, 0.000000000000000000, 0.000000000000000000 ) ) ;
#67356=CARTESIAN_POINT ( 'NONE',  ( 118.7087635252314328, -7.482591942790329030E-16, 6.110000000000001208 ) ) ;
#67394=CARTESIAN_POINT ( 'NONE',  ( 83.03709685856478018, -3.054999999999999272, -5.291415217122919401 ) ) ;
#67447=CARTESIAN_POINT ( 'NONE',  ( 100.0208333333333286, 7.949999999999999289, 2.130196079827431532 ) ) ;
#67450=ORIENTED_EDGE ( 'NONE', *, *, #111440, .F. ) ;
#67479=CARTESIAN_POINT ( 'NONE',  ( 119.0004301918981184, -3.055000000000002380, 5.291415217122920289 ) ) ;
#67489=CARTESIAN_POINT ( 'NONE',  ( 110.5995968585647802, -6.109999999999997655, -1.637169565754160283 ) ) ;
#67498=CARTESIAN_POINT ( 'NONE',  ( 35.43793019189810423, -6.110000000000001208, 1.637169565754158951 ) ) ;
#67505=CARTESIAN_POINT ( 'NONE',  ( 31.12043019189811233, 3.055000000000001936, -5.291415217122916737 ) ) ;
#67533=CARTESIAN_POINT ( 'NONE',  ( 50.80793019189810167, -6.109999999999998543, 1.637169565754158507 ) ) ;
#67563=EDGE_CURVE ( 'NONE', #33856, #83993, #131751, .T. ) ;
#67565=ORIENTED_EDGE ( 'NONE', *, *, #111236, .F. ) ;
#67572=CARTESIAN_POINT ( 'NONE',  ( 114.9745968585647660, 1.637169565754164280, -6.109999999999997655 ) ) ;
#67574=CARTESIAN_POINT ( 'NONE',  ( 62.78752705046289151, 0.000000000000000000, -7.949999999999998401 ) ) ;
#67580=ORIENTED_EDGE ( 'NONE', *, *, #74032, .F. ) ;
#67616=CARTESIAN_POINT ( 'NONE',  ( 125.5568156377396605, -3.969148909990495078, 6.850047280582228559 ) ) ;
#67617=CARTESIAN_POINT ( 'NONE',  ( 128.8500270504628986, -5.819803920172572198, -5.819803920172572198 ) ) ;
#67637=CARTESIAN_POINT ( 'NONE',  ( 119.2920968585647756, -5.291415217122921177, 3.054999999999999272 ) ) ;
#67647=CARTESIAN_POINT ( 'NONE',  ( 48.35002705046287730, -5.819803920172572198, -5.819803920172572198 ) ) ;
#67652=CARTESIAN_POINT ( 'NONE',  ( 42.70833333333333570, -3.974999999999999201, -6.884901960086287964 ) ) ;
#67664=CARTESIAN_POINT ( 'NONE',  ( 39.08376352523143282, -6.110000000000001208, -3.741295971395164515E-16 ) ) ;
#67681=CARTESIAN_POINT ( 'NONE',  ( 0.000000000000000000, 0.000000000000000000, 7.950000000000000178 ) ) ;
#67688=CARTESIAN_POINT ( 'NONE',  ( 62.62043019189811588, 3.055000000000001936, -5.291415217122916737 ) ) ;
#67691=CARTESIAN_POINT ( 'NONE',  ( 0.000000000000000000, 9.735942053221458872E-16, -7.950000000000000178 ) ) ;
#67718=CARTESIAN_POINT ( 'NONE',  ( 71.07876352523146579, -7.482591942790325086E-16, 6.109999999999998543 ) ) ;
#67726=CARTESIAN_POINT ( 'NONE',  ( 122.3333333333333286, -6.884901960086287964, 3.974999999999998312 ) ) ;
#67737=ORIENTED_EDGE ( 'NONE', *, *, #113563, .T. ) ;
#67742=CARTESIAN_POINT ( 'NONE',  ( 28.29209685856476497, -5.291415217122921177, 3.054999999999999272 ) ) ;
#67791=CARTESIAN_POINT ( 'NONE',  ( 64.97502705046288440, -5.819803920172573086, 5.819803920172573086 ) ) ;
#67801=CARTESIAN_POINT ( 'NONE',  ( 56.78709685856478728, 3.054999999999997939, 5.291415217122920289 ) ) ;
#67805=CARTESIAN_POINT ( 'NONE',  ( 84.99999999999998579, 0.000000000000000000, -7.950000000000000178 ) ) ;
#67826=CARTESIAN_POINT ( 'NONE',  ( 72.26669371712955581, -7.949999999999999289, 2.130196079827424427 ) ) ;
#67830=CARTESIAN_POINT ( 'NONE',  ( 75.08333333333332860, 6.884901960086290629, -3.974999999999994316 ) ) ;
#67842=CARTESIAN_POINT ( 'NONE',  ( 61.83376352523143993, 6.110000000000001208, 1.122388791418549305E-15 ) ) ;
#67861=CARTESIAN_POINT ( 'NONE',  ( 52.64626352523142572, -4.472830434245840259, 4.472830434245839371 ) ) ;
#67867=CARTESIAN_POINT ( 'NONE',  ( 54.81249999999999289, 5.819803920172571310, 5.819803920172576639 ) ) ;
#67873=VECTOR ( 'NONE', #4500, 1000.000000000000000 ) ;
#67878=CARTESIAN_POINT ( 'NONE',  ( 112.9541937171295558, 6.884901960086283523, 3.975000000000002753 ) ) ;
#67887=CYLINDRICAL_SURFACE ( 'NONE', #41339, 6.349999999999997868 ) ;
#67893=VERTEX_POINT ( 'NONE', #31812 ) ;
#67896=CARTESIAN_POINT ( 'NONE',  ( 107.2454301918981088, -5.291415217122918513, -3.055000000000000160 ) ) ;
#67921=CARTESIAN_POINT ( 'NONE',  ( 59.06293019189810423, 1.637169565754157174, 6.110000000000002984 ) ) ;
#67928=CARTESIAN_POINT ( 'NONE',  ( 94.35459685856476142, -1.637169565754161615, 6.110000000000000320 ) ) ;
#67990=ORIENTED_EDGE ( 'NONE', *, *, #68126, .F. ) ;
#67998=CARTESIAN_POINT ( 'NONE',  ( 101.7250270504628844, 5.819803920172573086, -5.819803920172572198 ) ) ;
#68017=CARTESIAN_POINT ( 'NONE',  ( 90.56293019189811844, 1.637169565754157174, 6.110000000000002984 ) ) ;
#68036=( BOUNDED_CURVE ( )  B_SPLINE_CURVE ( 2, ( #72712, #61801, #82140, #128473, #105276, #29146, #5226, #73389, #51631, #5927, #59664, #114706, #95822 ),
 .UNSPECIFIED., .F., .T. ) 
 B_SPLINE_CURVE_WITH_KNOTS ( ( 3, 2, 2, 2, 2, 2, 3 ),
 ( 0.6500000000000000222, 0.6527777777777777901, 0.6555555555555555580, 0.6583333333333333259, 0.6611111111111110938, 0.6638888888888888618, 0.6666666666666666297 ),
 .UNSPECIFIED. ) 
 CURVE ( )  GEOMETRIC_REPRESENTATION_ITEM ( )  RATIONAL_B_SPLINE_CURVE ( ( 1.000000000000000000, 0.9659258262890683122, 1.000000000000000000, 0.9659258262890683122, 1.000000000000000000, 0.9659258262890683122, 1.000000000000000000, 0.9659258262890683122, 1.000000000000000000, 0.9659258262890683122, 1.000000000000000000, 0.9659258262890683122, 1.000000000000000000 ) ) 
 REPRESENTATION_ITEM ( '' )  );
#68042=CARTESIAN_POINT ( 'NONE',  ( 85.31293019189811844, -1.637169565754159617, -6.110000000000001208 ) ) ;
#68054=CARTESIAN_POINT ( 'NONE',  ( 84.05793019189810877, 6.110000000000000320, -1.637169565754156064 ) ) ;
#68089=CARTESIAN_POINT ( 'NONE',  ( 115.7250270504628844, 5.819803920172573974, -5.819803920172573086 ) ) ;
#68101=CARTESIAN_POINT ( 'NONE',  ( 116.0837635252314470, -6.110000000000001208, -3.741295971395164515E-16 ) ) ;
#68126=EDGE_CURVE ( 'NONE', #72906, #143427, #141485, .T. ) ;
#68136=CARTESIAN_POINT ( 'NONE',  ( 81.43293019189809456, 1.637169565754156730, 6.110000000000001208 ) ) ;
#68139=CARTESIAN_POINT ( 'NONE',  ( 99.53752705046289861, -9.735942053221456900E-16, 7.949999999999998401 ) ) ;
#68150=AXIS2_PLACEMENT_3D ( 'NONE', #129362, #74298, #32213 ) ;
#68181=CARTESIAN_POINT ( 'NONE',  ( 111.2500000000000000, -9.735942053221458872E-16, 7.950000000000000178 ) ) ;
#68186=CARTESIAN_POINT ( 'NONE',  ( 89.22916666666667140, 7.950000000000001954, -2.130196079827421762 ) ) ;
#68193=ORIENTED_EDGE ( 'NONE', *, *, #103670, .T. ) ;
#68211=CARTESIAN_POINT ( 'NONE',  ( 117.3962635252314470, 4.472830434245840259, -4.472830434245839371 ) ) ;
#68219=CARTESIAN_POINT ( 'NONE',  ( 110.4537635252314516, -6.109999999999998543, -3.741295971395162543E-16 ) ) ;
#68234=CARTESIAN_POINT ( 'NONE',  ( 27.91209685856478728, 5.291415217122921177, -3.054999999999994831 ) ) ;
#68240=ORIENTED_EDGE ( 'NONE', *, *, #127793, .T. ) ;
#68264=CARTESIAN_POINT ( 'NONE',  ( 46.72459685856477307, -1.637169565754160949, 6.109999999999997655 ) ) ;
#68298=CARTESIAN_POINT ( 'NONE',  ( 107.8287635252314516, 0.000000000000000000, -6.109999999999999432 ) ) ;
#68357=CARTESIAN_POINT ( 'NONE',  ( 121.6254301918981184, 5.291415217122919401, 3.055000000000002824 ) ) ;
#68366=CARTESIAN_POINT ( 'NONE',  ( 50.39169371712955581, 2.130196079827421762, 7.950000000000001066 ) ) ;
#68371=CARTESIAN_POINT ( 'NONE',  ( 49.85416666666665719, -2.130196079827425315, -7.950000000000001066 ) ) ;
#68378=CARTESIAN_POINT ( 'NONE',  ( 39.22959685856475431, -6.110000000000000320, -1.637169565754161393 ) ) ;
#68399=( BOUNDED_CURVE ( )  B_SPLINE_CURVE ( 2, ( #11277, #64273, #21488, #88175, #108441, #8411, #96854, #20028, #55551, #33117, #19338, #53390, #63594 ),
 .UNSPECIFIED., .F., .T. ) 
 B_SPLINE_CURVE_WITH_KNOTS ( ( 3, 2, 2, 2, 2, 2, 3 ),
 ( 0.000000000000000000, 0.002777777777777391474, 0.005555555555554782948, 0.008333333333332174422, 0.01111111111110956590, 0.01388888888888695737, 0.01666666666666434884 ),
 .UNSPECIFIED. ) 
 CURVE ( )  GEOMETRIC_REPRESENTATION_ITEM ( )  RATIONAL_B_SPLINE_CURVE ( ( 1.000000000000000000, 0.9659258262890683122, 1.000000000000000000, 0.9659258262890683122, 1.000000000000000000, 0.9659258262890683122, 1.000000000000000000, 0.9659258262890683122, 1.000000000000000000, 0.9659258262890683122, 1.000000000000000000, 0.9659258262890967339, 0.9999999999999715783 ) ) 
 REPRESENTATION_ITEM ( '' )  );
#68401=CARTESIAN_POINT ( 'NONE',  ( 58.39126352523145158, -4.472830434245839371, -4.472830434245839371 ) ) ;
#68431=CARTESIAN_POINT ( 'NONE',  ( 72.68293019189810877, -1.637169565754158951, -6.109999999999998543 ) ) ;
#68455=CARTESIAN_POINT ( 'NONE',  ( 28.00043019189810067, -3.055000000000002380, 5.291415217122920289 ) ) ;
#68462=EDGE_LOOP ( 'NONE', ( #94386, #93916, #142291, #7665 ) ) ;
#68486=CARTESIAN_POINT ( 'NONE',  ( 25.89892480454907542, 0.000000000000000000, -6.350000000000003197 ) ) ;
#68501=CARTESIAN_POINT ( 'NONE',  ( 52.70376352523144448, 6.109999999999999432, 1.122388791418549108E-15 ) ) ;
#68519=CYLINDRICAL_SURFACE ( 'NONE', #113877, 7.950000000000000178 ) ;
#68523=CARTESIAN_POINT ( 'NONE',  ( 73.28752705046288440, 0.000000000000000000, -7.949999999999998401 ) ) ;
#68528=CARTESIAN_POINT ( 'NONE',  ( 76.68750000000000000, -5.819803920172573086, 5.819803920172572198 ) ) ;
#68537=CARTESIAN_POINT ( 'NONE',  ( 62.70876352523143993, -7.482591942790329030E-16, 6.110000000000001208 ) ) ;
#68538=EDGE_CURVE ( 'NONE', #91497, #74755, #16275, .T. ) ;
#68545=CARTESIAN_POINT ( 'NONE',  ( 86.02083333333331439, 7.949999999999998401, 2.130196079827431532 ) ) ;
#68555=CARTESIAN_POINT ( 'NONE',  ( 52.50043019189811133, -3.055000000000002380, 5.291415217122920289 ) ) ;
#68586=CARTESIAN_POINT ( 'NONE',  ( 101.9954301918981230, 5.291415217122916737, 3.055000000000001936 ) ) ;
#68610=CARTESIAN_POINT ( 'NONE',  ( 49.87543019189810423, -5.291415217122920289, -3.055000000000001492 ) ) ;
#68618=CARTESIAN_POINT ( 'NONE',  ( 92.89626352523143282, 4.472830434245840259, -4.472830434245838482 ) ) ;
#68631=CARTESIAN_POINT ( 'NONE',  ( 126.3495968585647944, 6.109999999999997655, 1.637169565754163836 ) ) ;
#68684=CARTESIAN_POINT ( 'NONE',  ( 107.7041937171295558, -6.884901960086285300, -3.975000000000000089 ) ) ;
#68687=VERTEX_POINT ( 'NONE', #87801 ) ;
#68697=ORIENTED_EDGE ( 'NONE', *, *, #555, .T. ) ;
#68699=CARTESIAN_POINT ( 'NONE',  ( 97.56293019189810423, 1.637169565754157174, 6.110000000000002984 ) ) ;
#68725=CARTESIAN_POINT ( 'NONE',  ( 84.14626352523144703, -4.472830434245840259, 4.472830434245839371 ) ) ;
#68740=CARTESIAN_POINT ( 'NONE',  ( 80.99543019189810877, 5.291415217122916737, 3.055000000000001936 ) ) ;
#68745=ORIENTED_EDGE ( 'NONE', *, *, #97260, .T. ) ;
#68750=CARTESIAN_POINT ( 'NONE',  ( 106.0000000000000000, 0.000000000000000000, -7.950000000000000178 ) ) ;
#68767=CARTESIAN_POINT ( 'NONE',  ( 56.22502705046289151, 5.819803920172573974, -5.819803920172573086 ) ) ;
#68794=CARTESIAN_POINT ( 'NONE',  ( 118.1254301918981184, 5.291415217122919401, 3.055000000000002824 ) ) ;
#68875=CARTESIAN_POINT ( 'NONE',  ( 90.10416666666665719, 2.130196079827422206, 7.950000000000001954 ) ) ;
#68888=CARTESIAN_POINT ( 'NONE',  ( 127.8079301918981230, -6.109999999999998543, 1.637169565754158507 ) ) ;
#68899=CARTESIAN_POINT ( 'NONE',  ( 110.5420968585647756, 5.291415217122923842, -3.054999999999996163 ) ) ;
#68911=CARTESIAN_POINT ( 'NONE',  ( 112.2037635252314516, 6.109999999999998543, 1.122388791418548911E-15 ) ) ;
#68922=CARTESIAN_POINT ( 'NONE',  ( 25.08376352523143638, -6.110000000000001208, -3.741295971395164515E-16 ) ) ;
#68929=CARTESIAN_POINT ( 'NONE',  ( 32.57876352523145158, -7.482591942790325086E-16, 6.109999999999998543 ) ) ;
#68948=CARTESIAN_POINT ( 'NONE',  ( 64.24586038379621300, 3.974999999999996980, 6.884901960086287964 ) ) ;
#68959=EDGE_CURVE ( 'NONE', #2613, #7898, #41282, .T. ) ;
#68960=CARTESIAN_POINT ( 'NONE',  ( 41.03709685856478728, -3.054999999999998828, -5.291415217122919401 ) ) ;
#68986=CARTESIAN_POINT ( 'NONE',  ( 111.0370968585647944, -3.054999999999999272, -5.291415217122919401 ) ) ;
#69028=CARTESIAN_POINT ( 'NONE',  ( 126.2426566364622005, -7.159809133051783014, 0.8799046258456960645 ) ) ;
#69029=CARTESIAN_POINT ( 'NONE',  ( 28.66252705046289151, 7.949999999999998401, 1.460391307983218338E-15 ) ) ;
#69035=CARTESIAN_POINT ( 'NONE',  ( 121.0208333333333144, 7.949999999999999289, 2.130196079827431532 ) ) ;
#69048=CARTESIAN_POINT ( 'NONE',  ( 118.4170968585647756, 3.054999999999998828, 5.291415217122922066 ) ) ;
#69058=CARTESIAN_POINT ( 'NONE',  ( 43.68336038379622011, -2.130196079827426203, 7.949999999999997513 ) ) ;
#69063=CARTESIAN_POINT ( 'NONE',  ( 31.62500000000000000, -7.950000000000000178, -4.867971026610729436E-16 ) ) ;
#69075=CARTESIAN_POINT ( 'NONE',  ( 35.29209685856476852, -5.291415217122921177, 3.054999999999999272 ) ) ;
#69088=CARTESIAN_POINT ( 'NONE',  ( 39.60002705046289151, 5.819803920172570422, 5.819803920172575751 ) ) ;
#69094=ADVANCED_FACE ( 'NONE', ( #85473 ), #65199, .T. ) ;
#69096=CARTESIAN_POINT ( 'NONE',  ( 61.16209685856478728, -5.291415217122919401, 3.054999999999997939 ) ) ;
#69101=DIRECTION ( 'NONE',  ( -1.000000000000000000, -0.000000000000000000, -0.000000000000000000 ) ) ;
#69124=EDGE_CURVE ( 'NONE', #143125, #123729, #31152, .T. ) ;
#69126=CARTESIAN_POINT ( 'NONE',  ( 70.93293019189810877, 1.637169565754156508, 6.110000000000000320 ) ) ;
#69132=CARTESIAN_POINT ( 'NONE',  ( 123.0625000000000000, -5.819803920172573086, -5.819803920172573974 ) ) ;
#69196=CARTESIAN_POINT ( 'NONE',  ( 56.05793019189811588, 6.110000000000001208, -1.637169565754156286 ) ) ;
#69199=CARTESIAN_POINT ( 'NONE',  ( 31.57919371712955581, 3.975000000000002753, -6.884901960086283523 ) ) ;
#69202=CARTESIAN_POINT ( 'NONE',  ( 26.51360224591381254, -6.350000000000003197, -3.888253587292850026E-16 ) ) ;
#69217=DIRECTION ( 'NONE',  ( 0.000000000000000000, 0.000000000000000000, 1.000000000000000000 ) ) ;
#69224=CARTESIAN_POINT ( 'NONE',  ( 77.66252705046289861, 7.949999999999998401, 1.460391307983218338E-15 ) ) ;
#69228=CARTESIAN_POINT ( 'NONE',  ( 74.64583333333331439, 2.130196079827431976, -7.949999999999999289 ) ) ;
#69239=CARTESIAN_POINT ( 'NONE',  ( 69.70876352523144703, -7.482591942790329030E-16, 6.110000000000001208 ) ) ;
#69259=CARTESIAN_POINT ( 'NONE',  ( 51.47959685856477563, 6.109999999999999432, 1.637169565754164280 ) ) ;
#69290=CARTESIAN_POINT ( 'NONE',  ( 105.9329301918981230, 1.637169565754156508, 6.110000000000000320 ) ) ;
#69291=ORIENTED_EDGE ( 'NONE', *, *, #111056, .T. ) ;
#69297=EDGE_CURVE ( 'NONE', #105597, #5049, #39703, .T. ) ;
#69310=CARTESIAN_POINT ( 'NONE',  ( 88.20833333333332860, -3.974999999999999201, -6.884901960086287964 ) ) ;
#69317=CARTESIAN_POINT ( 'NONE',  ( 57.89626352523144703, 4.472830434245840259, -4.472830434245838482 ) ) ;
#69321=CARTESIAN_POINT ( 'NONE',  ( 90.41709685856477563, 3.054999999999998828, 5.291415217122922066 ) ) ;
#69348=EDGE_CURVE ( 'NONE', #29421, #33782, #86878, .T. ) ;
#69392=CARTESIAN_POINT ( 'NONE',  ( 105.9541937171295700, 6.884901960086283523, 3.975000000000002753 ) ) ;
#69407=CARTESIAN_POINT ( 'NONE',  ( 95.95876352523144703, 0.000000000000000000, -6.110000000000001208 ) ) ;
#69432=ORIENTED_EDGE ( 'NONE', *, *, #121014, .F. ) ;
#69435=CARTESIAN_POINT ( 'NONE',  ( 82.10459685856476142, 1.637169565754164946, -6.109999999999999432 ) ) ;
#69448=CARTESIAN_POINT ( 'NONE',  ( 78.22459685856479439, -1.637169565754160949, 6.109999999999997655 ) ) ;
#69480=CARTESIAN_POINT ( 'NONE',  ( 57.10002705046289861, 5.819803920172570422, 5.819803920172575751 ) ) ;
#69503=CARTESIAN_POINT ( 'NONE',  ( 120.3129301918980900, -1.637169565754159617, -6.110000000000001208 ) ) ;
#69506=DIRECTION ( 'NONE',  ( -0.000000000000000000, 1.000000000000000000, 0.000000000000000000 ) ) ;
#69538=CARTESIAN_POINT ( 'NONE',  ( 9.182220855195383891, -8.505056546645496596, 4.232972564478894029 ) ) ;
#69539=CARTESIAN_POINT ( 'NONE',  ( 99.24586038379624142, 3.974999999999996980, 6.884901960086287964 ) ) ;
#69543=ORIENTED_EDGE ( 'NONE', *, *, #133203, .T. ) ;
#69571=VERTEX_POINT ( 'NONE', #122215 ) ;
#69591=ORIENTED_EDGE ( 'NONE', *, *, #105948, .F. ) ;
#69592=CARTESIAN_POINT ( 'NONE',  ( 94.77083333333331439, -7.949999999999999289, -2.130196079827426203 ) ) ;
#69600=CARTESIAN_POINT ( 'NONE',  ( 13.61885681777355472, 9.051170952377558976, -2.893263300195505039 ) ) ;
#69605=CARTESIAN_POINT ( 'NONE',  ( 126.8279612232013562, 4.169058294950168886, 5.151117689787611198 ) ) ;
#69606=CARTESIAN_POINT ( 'NONE',  ( 128.8287635252314658, 0.000000000000000000, -6.109999999999998543 ) ) ;
#69619=CARTESIAN_POINT ( 'NONE',  ( 110.8337635252314470, 6.110000000000001208, 1.122388791418549305E-15 ) ) ;
#69628=CARTESIAN_POINT ( 'NONE',  ( 105.2037635252314516, 6.109999999999998543, 1.122388791418548911E-15 ) ) ;
#69636=CARTESIAN_POINT ( 'NONE',  ( 98.12500000000000000, -7.950000000000000178, -4.867971026610729436E-16 ) ) ;
#69673=VERTEX_POINT ( 'NONE', #125821 ) ;
#69677=CARTESIAN_POINT ( 'NONE',  ( 40.45376352523144448, -6.109999999999998543, -3.741295971395162543E-16 ) ) ;
#69712=CARTESIAN_POINT ( 'NONE',  ( 111.6204301918981088, 3.055000000000002380, -5.291415217122917625 ) ) ;
#69768=CARTESIAN_POINT ( 'NONE',  ( 117.2291666666666572, 7.950000000000001954, -2.130196079827421762 ) ) ;
#69782=CARTESIAN_POINT ( 'NONE',  ( 115.0629301918981042, 1.637169565754157174, 6.110000000000002984 ) ) ;
#69786=CARTESIAN_POINT ( 'NONE',  ( 105.2250270504628986, 5.819803920172573974, -5.819803920172573086 ) ) ;
#69791=CARTESIAN_POINT ( 'NONE',  ( 42.66252705046289151, 7.949999999999998401, 1.460391307983218338E-15 ) ) ;
#69798=CARTESIAN_POINT ( 'NONE',  ( 39.20833333333332860, -3.974999999999999201, -6.884901960086287964 ) ) ;
#69809=CARTESIAN_POINT ( 'NONE',  ( 27.27126352523142572, 4.472830434245839371, 4.472830434245842035 ) ) ;
#69826=CARTESIAN_POINT ( 'NONE',  ( 57.80793019189810877, -6.109999999999998543, 1.637169565754158063 ) ) ;
#69859=CARTESIAN_POINT ( 'NONE',  ( 68.74543019189812298, -5.291415217122918513, -3.055000000000000160 ) ) ;
#69870=CARTESIAN_POINT ( 'NONE',  ( 35.27083333333331439, -7.949999999999998401, -2.130196079827426203 ) ) ;
#69878=ORIENTED_EDGE ( 'NONE', *, *, #28374, .F. ) ;
#69886=CARTESIAN_POINT ( 'NONE',  ( 30.75000000000000000, -9.735942053221458872E-16, 7.950000000000000178 ) ) ;
#69898=CARTESIAN_POINT ( 'NONE',  ( 119.8083603837962272, 7.949999999999996625, 2.130196079827431088 ) ) ;
#69899=AXIS2_PLACEMENT_3D ( 'NONE', #59635, #45371, #116112 ) ;
#69944=CARTESIAN_POINT ( 'NONE',  ( 59.41209685856478728, 5.291415217122922066, -3.054999999999995275 ) ) ;
#69956=AXIS2_PLACEMENT_3D ( 'NONE', #95277, #71405, #82993 ) ;
#69969=CARTESIAN_POINT ( 'NONE',  ( 73.14169371712957002, -2.130196079827424871, -7.949999999999999289 ) ) ;
#69973=CARTESIAN_POINT ( 'NONE',  ( 65.89583333333332860, -2.130196079827427091, 7.949999999999999289 ) ) ;
#69983=CARTESIAN_POINT ( 'NONE',  ( 62.85459685856477563, -1.637169565754161615, 6.110000000000000320 ) ) ;
#70004=EDGE_CURVE ( 'NONE', #24590, #140445, #11122, .T. ) ;
#70008=ORIENTED_EDGE ( 'NONE', *, *, #62571, .F. ) ;
#70017=AXIS2_PLACEMENT_3D ( 'NONE', #31201, #75419, #129779 ) ;
#70034=CARTESIAN_POINT ( 'NONE',  ( 97.62043019189812298, 3.055000000000001936, -5.291415217122916737 ) ) ;
#70064=CARTESIAN_POINT ( 'NONE',  ( 49.43793019189809002, -6.110000000000001208, 1.637169565754158951 ) ) ;
#70087=ORIENTED_EDGE ( 'NONE', *, *, #49407, .F. ) ;
#70117=CARTESIAN_POINT ( 'NONE',  ( 6.534046899938177333, 9.244424685250681506, 2.202405500345624212 ) ) ;
#70136=CARTESIAN_POINT ( 'NONE',  ( 120.8291937171295700, -3.975000000000001865, 6.884901960086284411 ) ) ;
#70139=CARTESIAN_POINT ( 'NONE',  ( 105.5166937171295558, 7.950000000000001066, -2.130196079827421318 ) ) ;
#70157=CARTESIAN_POINT ( 'NONE',  ( 98.29209685856477563, -5.291415217122921177, 3.054999999999999272 ) ) ;
#70166=DIRECTION ( 'NONE',  ( 0.000000000000000000, 0.000000000000000000, -1.000000000000000000 ) ) ;
#70179=CARTESIAN_POINT ( 'NONE',  ( 83.27126352523143282, 4.472830434245839371, 4.472830434245842035 ) ) ;
#70191=CARTESIAN_POINT ( 'NONE',  ( 73.70376352523145158, 6.109999999999998543, 1.122388791418548911E-15 ) ) ;
#70196=EDGE_CURVE ( 'NONE', #49442, #33856, #140615, .T. ) ;
#70240=EDGE_CURVE ( 'NONE', #44417, #114577, #61908, .T. ) ;
#70244=CARTESIAN_POINT ( 'NONE',  ( 116.8129301918981184, -1.637169565754159617, -6.110000000000001208 ) ) ;
#70245=FACE_OUTER_BOUND ( 'NONE', #104598, .T. ) ;
#70249=VECTOR ( 'NONE', #84689, 1000.000000000000000 ) ;
#70284=DIRECTION ( 'NONE',  ( 0.000000000000000000, 0.000000000000000000, 1.000000000000000000 ) ) ;
#70295=FACE_OUTER_BOUND ( 'NONE', #34818, .T. ) ;
#70310=CARTESIAN_POINT ( 'NONE',  ( 31.12043019189811233, 3.055000000000002380, -5.291415217122917625 ) ) ;
#70313=CARTESIAN_POINT ( 'NONE',  ( 47.47502705046287730, -5.819803920172573086, 5.819803920172573086 ) ) ;
#70314=CARTESIAN_POINT ( 'NONE',  ( 88.50000000000000000, 0.000000000000000000, -7.950000000000000178 ) ) ;
#70326=CARTESIAN_POINT ( 'NONE',  ( 95.93750000000000000, 5.819803920172573974, -5.819803920172572198 ) ) ;
#70333=CARTESIAN_POINT ( 'NONE',  ( 10.61372115956010376, 8.432637487761468265, -4.375000000000002665 ) ) ;
#70351=CARTESIAN_POINT ( 'NONE',  ( 107.6254301918981042, 5.291415217122919401, 3.055000000000002824 ) ) ;
#70360=CARTESIAN_POINT ( 'NONE',  ( 102.5787635252314658, -7.482591942790325086E-16, 6.109999999999998543 ) ) ;
#70376=SHAPE_REPRESENTATION_RELATIONSHIP ( 'NONE' , 'NONE' ,  #58954, #70809 ) ;
#70380=ORIENTED_EDGE ( 'NONE', *, *, #98175, .F. ) ;
#70392=AXIS2_PLACEMENT_3D ( 'NONE', #45825, #121905, #88612 ) ;
#70415=CARTESIAN_POINT ( 'NONE',  ( 36.07876352523144448, -7.482591942790325086E-16, 6.109999999999998543 ) ) ;
#70420=CARTESIAN_POINT ( 'NONE',  ( 0.000000000000000000, 9.735942053221458872E-16, -7.950000000000000178 ) ) ;
#70447=CARTESIAN_POINT ( 'NONE',  ( 101.8495968585647660, 6.109999999999997655, 1.637169565754163836 ) ) ;
#70489=CARTESIAN_POINT ( 'NONE',  ( 126.0561293963919667, -6.895973075043523970, 2.684650104021446992 ) ) ;
#70495=ORIENTED_EDGE ( 'NONE', *, *, #73083, .F. ) ;
#70496=CARTESIAN_POINT ( 'NONE',  ( 117.6666666666666714, 6.884901960086285300, 3.975000000000003642 ) ) ;
#70510=CARTESIAN_POINT ( 'NONE',  ( 109.0837635252314470, -6.110000000000001208, -3.741295971395164515E-16 ) ) ;
#70520=CARTESIAN_POINT ( 'NONE',  ( 39.60002705046289151, 5.819803920172570422, 5.819803920172574863 ) ) ;
#70526=CARTESIAN_POINT ( 'NONE',  ( 38.18749999999998579, -5.819803920172573086, 5.819803920172572198 ) ) ;
#70536=CARTESIAN_POINT ( 'NONE',  ( 28.43793019189810423, -6.110000000000001208, 1.637169565754158951 ) ) ;
#70550=CARTESIAN_POINT ( 'NONE',  ( 44.68293019189811588, -1.637169565754158951, -6.109999999999998543 ) ) ;
#70552=CARTESIAN_POINT ( 'NONE',  ( 123.6458333333333286, 2.130196079827412436, -7.950000000000009059 ) ) ;
#70579=CARTESIAN_POINT ( 'NONE',  ( 70.49543019189810877, 5.291415217122916737, 3.055000000000001936 ) ) ;
#70649=CARTESIAN_POINT ( 'NONE',  ( 45.84959685856478018, 6.109999999999997655, 1.637169565754163836 ) ) ;
#70670=CARTESIAN_POINT ( 'NONE',  ( 69.78752705046289861, 0.000000000000000000, -7.949999999999998401 ) ) ;
#70674=ORIENTED_EDGE ( 'NONE', *, *, #126459, .F. ) ;
#70675=CARTESIAN_POINT ( 'NONE',  ( 60.50000000000000000, 0.000000000000000000, -7.950000000000000178 ) ) ;
#70685=CARTESIAN_POINT ( 'NONE',  ( 56.43793019189809712, -6.110000000000001208, 1.637169565754158951 ) ) ;
#70710=CARTESIAN_POINT ( 'NONE',  ( 110.3291937171295700, -3.975000000000001865, 6.884901960086284411 ) ) ;
#70721=CARTESIAN_POINT ( 'NONE',  ( 61.47502705046287730, -5.819803920172573086, 5.819803920172573086 ) ) ;
#70735=CARTESIAN_POINT ( 'NONE',  ( 93.09959685856478018, -6.109999999999997655, -1.637169565754160283 ) ) ;
#70757=CARTESIAN_POINT ( 'NONE',  ( 49.14626352523143282, -4.472830434245840259, 4.472830434245838482 ) ) ;
#70787=CARTESIAN_POINT ( 'NONE',  ( 0.000000000000000000, 0.000000000000000000, 0.000000000000000000 ) ) ;
#70792=CARTESIAN_POINT ( 'NONE',  ( 95.93750000000000000, 5.819803920172574863, -5.819803920172573086 ) ) ;
#70805=CARTESIAN_POINT ( 'NONE',  ( 74.14126352523146579, 4.472830434245837594, 4.472830434245841147 ) ) ;
#70806=CARTESIAN_POINT ( 'NONE',  ( 73.87086038379622721, 6.884901960086289741, -3.974999999999993427 ) ) ;
#70809=ADVANCED_BREP_SHAPE_REPRESENTATION ( '', ( #142006, #127880 ), #12041 ) ;
#70825=CARTESIAN_POINT ( 'NONE',  ( 120.5375270504628844, -9.735942053221456900E-16, 7.949999999999998401 ) ) ;
#70828=CARTESIAN_POINT ( 'NONE',  ( 103.9125270504628844, -7.949999999999998401, -4.867971026610728450E-16 ) ) ;
#70844=CARTESIAN_POINT ( 'NONE',  ( 89.10459685856477563, 1.637169565754164946, -6.109999999999999432 ) ) ;
#70853=CARTESIAN_POINT ( 'NONE',  ( 0.000000000000000000, 0.000000000000000000, 7.950000000000000178 ) ) ;
#70865=CARTESIAN_POINT ( 'NONE',  ( 82.25043019189810423, 3.055000000000002824, -5.291415217122919401 ) ) ;
#70878=CARTESIAN_POINT ( 'NONE',  ( 72.53709685856478018, -3.054999999999998828, -5.291415217122919401 ) ) ;
#70904=CARTESIAN_POINT ( 'NONE',  ( 68.03752705046289861, -9.735942053221456900E-16, 7.949999999999998401 ) ) ;
#70906=EDGE_LOOP ( 'NONE', ( #61741, #1680, #26980, #25441, #52784, #114396, #101745 ) ) ;
#70910=CARTESIAN_POINT ( 'NONE',  ( 0.000000000000000000, 0.000000000000000000, 9.500000000000001776 ) ) ;
#70911=LINE ( 'NONE', #115062, #100057 ) ;
#70922=CARTESIAN_POINT ( 'NONE',  ( 77.43793019189809002, -6.110000000000001208, 1.637169565754158951 ) ) ;
#70928=CARTESIAN_POINT ( 'NONE',  ( 107.1879301918980900, 6.110000000000002984, -1.637169565754156730 ) ) ;
#70958=CARTESIAN_POINT ( 'NONE',  ( 14.67146529891954110, -9.486753853592309937, 0.5779121670573046377 ) ) ;
#70998=CARTESIAN_POINT ( 'NONE',  ( 28.49543019189811233, 5.291415217122917625, 3.055000000000002380 ) ) ;
#71012=CARTESIAN_POINT ( 'NONE',  ( 89.81250000000000000, 5.819803920172571310, 5.819803920172575751 ) ) ;
#71025=CARTESIAN_POINT ( 'NONE',  ( 126.2730375289500557, 6.754077994965395959, -2.478850524292684376 ) ) ;
#71037=CARTESIAN_POINT ( 'NONE',  ( 113.7504301918981042, 3.055000000000002824, -5.291415217122919401 ) ) ;
#71046=CARTESIAN_POINT ( 'NONE',  ( 100.5370968585647802, -3.054999999999998828, -5.291415217122919401 ) ) ;
#71096=CARTESIAN_POINT ( 'NONE',  ( 39.43293019189811588, 1.637169565754156508, 6.110000000000000320 ) ) ;
#71129=CARTESIAN_POINT ( 'NONE',  ( 98.34959685856479439, 6.109999999999997655, 1.637169565754163836 ) ) ;
#71179=ORIENTED_EDGE ( 'NONE', *, *, #112399, .F. ) ;
#71180=CARTESIAN_POINT ( 'NONE',  ( 122.4791666666666714, -7.950000000000001066, 2.130196079827424427 ) ) ;
#71192=CARTESIAN_POINT ( 'NONE',  ( 110.9795968585647756, 6.109999999999999432, 1.637169565754164280 ) ) ;
#71195=CARTESIAN_POINT ( 'NONE',  ( 105.3708603837962272, 6.884901960086289741, -3.974999999999993427 ) ) ;
#71197=CARTESIAN_POINT ( 'NONE',  ( 83.35002705046287019, -5.819803920172573086, -5.819803920172573086 ) ) ;
#71204=CARTESIAN_POINT ( 'NONE',  ( 36.53752705046288440, -9.735942053221456900E-16, 7.949999999999998401 ) ) ;
#71209=CARTESIAN_POINT ( 'NONE',  ( 34.97916666666664298, -7.950000000000001066, 2.130196079827424427 ) ) ;
#71219=CARTESIAN_POINT ( 'NONE',  ( 28.58376352523143993, -6.110000000000001208, -3.741295971395164515E-16 ) ) ;
#71231=FACE_OUTER_BOUND ( 'NONE', #78153, .T. ) ;
#71237=CARTESIAN_POINT ( 'NONE',  ( 52.99543019189811588, 5.291415217122916737, 3.055000000000001936 ) ) ;
#71248=ORIENTED_EDGE ( 'NONE', *, *, #98175, .T. ) ;
#71260=ORIENTED_EDGE ( 'NONE', *, *, #87012, .T. ) ;
#71265=CARTESIAN_POINT ( 'NONE',  ( 65.53709685856478018, -3.054999999999998828, -5.291415217122919401 ) ) ;
#71268=FACE_OUTER_BOUND ( 'NONE', #1249, .T. ) ;
#71276=CARTESIAN_POINT ( 'NONE',  ( 101.0416666666666714, -3.975000000000002753, 6.884901960086286188 ) ) ;
#71337=CARTESIAN_POINT ( 'NONE',  ( 48.76626352523144448, 4.472830434245839371, -4.472830434245839371 ) ) ;
#71359=CARTESIAN_POINT ( 'NONE',  ( 116.9375000000000000, 5.819803920172574863, -5.819803920172573086 ) ) ;
#71360=CARTESIAN_POINT ( 'NONE',  ( 63.66252705046289151, 7.949999999999998401, 1.460391307983218338E-15 ) ) ;
#71365=CARTESIAN_POINT ( 'NONE',  ( 62.97916666666667140, -7.950000000000001066, 2.130196079827424427 ) ) ;
#71370=CARTESIAN_POINT ( 'NONE',  ( 32.64583333333332860, 2.130196079827356037, -7.950000000000043698 ) ) ;
#71372=CARTESIAN_POINT ( 'NONE',  ( 60.66709685856477563, -3.055000000000000160, -5.291415217122921177 ) ) ;
#71374=DIRECTION ( 'NONE',  ( 0.000000000000000000, 0.000000000000000000, 1.000000000000000000 ) ) ;
#71405=DIRECTION ( 'NONE',  ( -1.000000000000000000, -0.000000000000000000, -0.000000000000000000 ) ) ;
#71408=EDGE_CURVE ( 'NONE', #114577, #108642, #125576, .T. ) ;
#71426=CARTESIAN_POINT ( 'NONE',  ( 96.30793019189810877, -6.109999999999998543, 1.637169565754158507 ) ) ;
#71432=CARTESIAN_POINT ( 'NONE',  ( 55.24999999999999289, -9.735942053221458872E-16, 7.950000000000000178 ) ) ;
#71435=EDGE_CURVE ( 'NONE', #49146, #74280, #7224, .T. ) ;
#71447=VERTEX_POINT ( 'NONE', #60453 ) ;
#71452=CARTESIAN_POINT ( 'NONE',  ( 46.22959685856476852, -6.110000000000000320, -1.637169565754161393 ) ) ;
#71466=CARTESIAN_POINT ( 'NONE',  ( 0.000000000000000000, 0.000000000000000000, 0.000000000000000000 ) ) ;
#71471=EDGE_LOOP ( 'NONE', ( #119625, #61117, #99602, #55081 ) ) ;
#71489=CARTESIAN_POINT ( 'NONE',  ( 96.52083333333332860, 7.949999999999998401, 2.130196079827431532 ) ) ;
#71502=CARTESIAN_POINT ( 'NONE',  ( 76.18293019189810877, -1.637169565754159173, -6.109999999999999432 ) ) ;
#71504=CARTESIAN_POINT ( 'NONE',  ( 79.74999999999998579, -9.735942053221458872E-16, 7.950000000000000178 ) ) ;
#71527=CARTESIAN_POINT ( 'NONE',  ( 121.8500270504628844, -5.819803920172573086, -5.819803920172573086 ) ) ;
#71533=CARTESIAN_POINT ( 'NONE',  ( 90.49586038379622721, -3.974999999999998312, -6.884901960086286188 ) ) ;
#71534=CARTESIAN_POINT ( 'NONE',  ( 72.45833333333332860, 3.974999999999997424, 6.884901960086288852 ) ) ;
#71541=ADVANCED_FACE ( 'NONE', ( #82902, #127089 ), #17602, .T. ) ;
#71547=CARTESIAN_POINT ( 'NONE',  ( 80.20876352523143282, -7.482591942790329030E-16, 6.110000000000001208 ) ) ;
#71564=EDGE_CURVE ( 'NONE', #93164, #92088, #86469, .T. ) ;
#71567=CARTESIAN_POINT ( 'NONE',  ( 73.64626352523141861, -4.472830434245840259, 4.472830434245839371 ) ) ;
#71576=EDGE_LOOP ( 'NONE', ( #77514, #95367, #110543, #69878 ) ) ;
#71613=CARTESIAN_POINT ( 'NONE',  ( 0.000000000000000000, 0.000000000000000000, 7.950000000000000178 ) ) ;
#71625=CARTESIAN_POINT ( 'NONE',  ( 73.35459685856476142, -1.637169565754161615, 6.110000000000000320 ) ) ;
#71631=CARTESIAN_POINT ( 'NONE',  ( 107.0420968585647756, 5.291415217122923842, -3.054999999999996163 ) ) ;
#71699=CARTESIAN_POINT ( 'NONE',  ( 106.0000000000000000, 0.000000000000000000, -7.950000000000000178 ) ) ;
#71700=CARTESIAN_POINT ( 'NONE',  ( 126.0791937171295558, 3.975000000000002753, -6.884901960086283523 ) ) ;
#71704=CARTESIAN_POINT ( 'NONE',  ( 83.78752705046288440, 0.000000000000000000, -7.949999999999998401 ) ) ;
#71718=CARTESIAN_POINT ( 'NONE',  ( 86.16666666666667140, 6.884901960086285300, 3.975000000000003642 ) ) ;
#71734=CARTESIAN_POINT ( 'NONE',  ( 126.6594863501952801, 5.928045853110953445, 3.350272726927312483 ) ) ;
#71740=CARTESIAN_POINT ( 'NONE',  ( 79.74999999999998579, -9.735942053221458872E-16, 7.950000000000000178 ) ) ;
#71749=CARTESIAN_POINT ( 'NONE',  ( 111.7087635252314470, -7.482591942790329030E-16, 6.110000000000001208 ) ) ;
#71758=CARTESIAN_POINT ( 'NONE',  ( 101.5579301918981088, 6.110000000000000320, -1.637169565754156064 ) ) ;
#71768=EDGE_LOOP ( 'NONE', ( #70087, #46381 ) ) ;
#71781=CARTESIAN_POINT ( 'NONE',  ( 112.0579301918981230, 6.110000000000000320, -1.637169565754156064 ) ) ;
#71810=CARTESIAN_POINT ( 'NONE',  ( 33.74543019189811588, -5.291415217122918513, -3.055000000000000160 ) ) ;
#71849=CARTESIAN_POINT ( 'NONE',  ( 102.5787635252314658, -7.482591942790327058E-16, 6.109999999999999432 ) ) ;
#71902=CARTESIAN_POINT ( 'NONE',  ( 117.9583333333333286, 3.974999999999997424, 6.884901960086288852 ) ) ;
#71919=CARTESIAN_POINT ( 'NONE',  ( 112.0004301918981042, -3.055000000000002380, 5.291415217122920289 ) ) ;
#71927=CARTESIAN_POINT ( 'NONE',  ( 36.97502705046289861, -5.819803920172572198, 5.819803920172572198 ) ) ;
#71932=CARTESIAN_POINT ( 'NONE',  ( 32.49999999999998579, 0.000000000000000000, -7.950000000000000178 ) ) ;
#71944=CARTESIAN_POINT ( 'NONE',  ( 30.18793019189809357, 6.110000000000002984, -1.637169565754156730 ) ) ;
#71953=CARTESIAN_POINT ( 'NONE',  ( 63.56249999999999289, -5.819803920172573086, -5.819803920172573974 ) ) ;
#71955=CARTESIAN_POINT ( 'NONE',  ( 55.12543019189811133, 5.291415217122919401, 3.055000000000002824 ) ) ;
#71963=CARTESIAN_POINT ( 'NONE',  ( 46.57876352523145158, -7.482591942790325086E-16, 6.109999999999998543 ) ) ;
#71993=CARTESIAN_POINT ( 'NONE',  ( 70.34959685856479439, 6.109999999999996767, 1.637169565754163836 ) ) ;
#72005=CARTESIAN_POINT ( 'NONE',  ( 35.12499999999999289, -7.950000000000000178, -4.867971026610729436E-16 ) ) ;
#72033=B_SPLINE_CURVE_WITH_KNOTS ( 'NONE', 3,
 ( #136974, #125393, #37681, #81181, #4239, #102925, #92733, #14479, #60147, #24632, #25341, #58756, #81918, #113791, #126108, #26077, #26774, #104311, #35561, #60887, #124665, #137702, #102223, #71025, #3566, #115174, #135561, #47861, #27471, #48535, #4981, #79789, #49282, #5711, #71734, #93468, #114484, #15850, #38376, #69605, #82590, #92027, #105048, #136246, #126787 ),
 .UNSPECIFIED., .F., .F.,
 ( 4, 2, 2, 2, 2, 2, 2, 2, 1, 2, 2, 2, 2, 2, 2, 1, 2, 2, 2, 2, 1, 2, 2, 4 ),
 ( 6.981499371183832972E-15, 0.001511458381938139781, 0.002267187572903719191, 0.003022916763869298602, 0.004534375145800453519, 0.006045833527731608002, 0.007557291909662763353, 0.008313021100628342763, 0.009068750291593921306, 0.009824479482559499849, 0.01058020867352508013, 0.01209166705545623548, 0.01360312543738739256, 0.01511458381931854618, 0.01587031301028412125, 0.01662604220124970153, 0.01738177139221527834, 0.01813750058318085515, 0.01964895896511201223, 0.02040468815607758904, 0.02116041734704316932, 0.02191614653800874959, 0.02267187572897432640, 0.02418333411090548696 ),
 .UNSPECIFIED. ) ;
#72081=CARTESIAN_POINT ( 'NONE',  ( 43.22459685856478728, -1.637169565754161171, 6.109999999999998543 ) ) ;
#72104=CARTESIAN_POINT ( 'NONE',  ( 68.91252705046288440, -7.949999999999998401, -4.867971026610728450E-16 ) ) ;
#72108=CARTESIAN_POINT ( 'NONE',  ( 67.50000000000000000, 0.000000000000000000, -7.950000000000000178 ) ) ;
#72118=CARTESIAN_POINT ( 'NONE',  ( 59.79209685856477563, -5.291415217122921177, 3.054999999999999272 ) ) ;
#72146=CARTESIAN_POINT ( 'NONE',  ( 110.6208603837962272, -6.884901960086286188, 3.974999999999997424 ) ) ;
#72167=DIRECTION ( 'NONE',  ( 0.000000000000000000, 0.000000000000000000, 1.000000000000000000 ) ) ;
#72175=CARTESIAN_POINT ( 'NONE',  ( 90.18293019189812298, -1.637169565754158951, -6.109999999999998543 ) ) ;
#72205=CARTESIAN_POINT ( 'NONE',  ( 42.87543019189810423, -5.291415217122920289, -3.055000000000001492 ) ) ;
#72215=FACE_OUTER_BOUND ( 'NONE', #9572, .T. ) ;
#72240=CARTESIAN_POINT ( 'NONE',  ( 66.04166666666667140, -3.975000000000002753, 6.884901960086286188 ) ) ;
#72258=CARTESIAN_POINT ( 'NONE',  ( 73.70376352523145158, 6.109999999999999432, 1.122388791418549108E-15 ) ) ;
#72260=CARTESIAN_POINT ( 'NONE',  ( 74.30836038379624142, 7.949999999999996625, 2.130196079827431088 ) ) ;
#72284=( BOUNDED_CURVE ( )  B_SPLINE_CURVE ( 2, ( #3895, #37295, #3214, #4588, #91667, #82249, #79424, #125009, #92359, #71359, #16211, #134479, #81542 ),
 .UNSPECIFIED., .F., .T. ) 
 B_SPLINE_CURVE_WITH_KNOTS ( ( 3, 2, 2, 2, 2, 2, 3 ),
 ( 0.08333333333333341197, 0.08611111111111116601, 0.08888888888888893391, 0.09166666666666667407, 0.09444444444444442810, 0.09722222222222219601, 0.09999999999999995004 ),
 .UNSPECIFIED. ) 
 CURVE ( )  GEOMETRIC_REPRESENTATION_ITEM ( )  RATIONAL_B_SPLINE_CURVE ( ( 0.9999999999999990008, 0.9659258262890693114, 1.000000000000000000, 0.9659258262890683122, 1.000000000000000000, 0.9659258262890683122, 1.000000000000000000, 0.9659258262890683122, 1.000000000000000000, 0.9659258262890683122, 1.000000000000000000, 0.9659258262890689783, 0.9999999999999993339 ) ) 
 REPRESENTATION_ITEM ( '' )  );
#72285=CARTESIAN_POINT ( 'NONE',  ( 96.91252705046289861, -7.949999999999998401, -4.867971026610728450E-16 ) ) ;
#72286=CARTESIAN_POINT ( 'NONE',  ( 71.29166666666667140, 3.975000000000003642, -6.884901960086285300 ) ) ;
#72300=CARTESIAN_POINT ( 'NONE',  ( 82.54209685856478984, 5.291415217122923842, -3.054999999999996163 ) ) ;
#72319=CARTESIAN_POINT ( 'NONE',  ( 75.39626352523141861, 4.472830434245840259, -4.472830434245839371 ) ) ;
#72376=CARTESIAN_POINT ( 'NONE',  ( 73.06293019189810423, 1.637169565754157174, 6.110000000000002984 ) ) ;
#72381=CARTESIAN_POINT ( 'NONE',  ( 109.3754301918981042, -5.291415217122920289, -3.055000000000001492 ) ) ;
#72396=CARTESIAN_POINT ( 'NONE',  ( 114.4125270504628986, -7.949999999999998401, -4.867971026610728450E-16 ) ) ;
#72411=CARTESIAN_POINT ( 'NONE',  ( 10.61499488414559700, -8.432637487761464712, 4.375000000000002665 ) ) ;
#72439=CARTESIAN_POINT ( 'NONE',  ( 105.2708333333333428, -7.949999999999998401, -2.130196079827426203 ) ) ;
#72445=CARTESIAN_POINT ( 'NONE',  ( 125.6416937171295700, -2.130196079827424871, -7.949999999999999289 ) ) ;
#72459=CARTESIAN_POINT ( 'NONE',  ( 80.77083333333331439, -7.949999999999999289, -2.130196079827426203 ) ) ;
#72487=CARTESIAN_POINT ( 'NONE',  ( 102.0837635252314328, -6.110000000000001208, -3.741295971395164515E-16 ) ) ;
#72498=CARTESIAN_POINT ( 'NONE',  ( 102.1412635252314232, 4.472830434245836706, 4.472830434245840259 ) ) ;
#72527=CARTESIAN_POINT ( 'NONE',  ( 114.2454301918981230, -5.291415217122918513, -3.055000000000000160 ) ) ;
#72552=CARTESIAN_POINT ( 'NONE',  ( 32.87043019189811588, -3.055000000000001492, 5.291415217122917625 ) ) ;
#72592=CARTESIAN_POINT ( 'NONE',  ( 102.4329301918980946, 1.637169565754156730, 6.110000000000001208 ) ) ;
#72614=ORIENTED_EDGE ( 'NONE', *, *, #142907, .T. ) ;
#72630=CARTESIAN_POINT ( 'NONE',  ( 26.88558207307487891, 6.350000000000002309, 1.302735879833260446 ) ) ;
#72637=CARTESIAN_POINT ( 'NONE',  ( 112.4166666666666714, -6.884901960086287076, -3.975000000000000977 ) ) ;
#72649=CARTESIAN_POINT ( 'NONE',  ( 101.7920968585647756, -5.291415217122921177, 3.054999999999999272 ) ) ;
#72662=CARTESIAN_POINT ( 'NONE',  ( 42.07919371712954870, 3.975000000000002753, -6.884901960086283523 ) ) ;
#72663=CARTESIAN_POINT ( 'NONE',  ( 107.7500000000000000, -9.735942053221458872E-16, 7.950000000000000178 ) ) ;
#72668=CARTESIAN_POINT ( 'NONE',  ( 127.3129301918980900, -1.637169565754159617, -6.110000000000001208 ) ) ;
#72679=CARTESIAN_POINT ( 'NONE',  ( 128.6829301918981230, -1.637169565754158951, -6.109999999999998543 ) ) ;
#72690=CARTESIAN_POINT ( 'NONE',  ( 57.75043019189809712, 3.055000000000002824, -5.291415217122919401 ) ) ;
#72692=DIRECTION ( 'NONE',  ( 0.000000000000000000, 0.000000000000000000, 1.000000000000000000 ) ) ;
#72700=CARTESIAN_POINT ( 'NONE',  ( 51.39126352523145158, -4.472830434245839371, -4.472830434245839371 ) ) ;
#72712=CARTESIAN_POINT ( 'NONE',  ( 61.03752705046289151, -9.735942053221456900E-16, 7.949999999999998401 ) ) ;
#72732=CARTESIAN_POINT ( 'NONE',  ( 55.62043019189812298, 3.055000000000001936, -5.291415217122916737 ) ) ;
#72806=CARTESIAN_POINT ( 'NONE',  ( 44.09959685856477307, -6.109999999999998543, -1.637169565754160727 ) ) ;
#72831=CARTESIAN_POINT ( 'NONE',  ( 69.20419371712955581, -6.884901960086285300, -3.975000000000000089 ) ) ;
#72836=CARTESIAN_POINT ( 'NONE',  ( 66.62499999999998579, -7.950000000000000178, -4.867971026610729436E-16 ) ) ;
#72842=CARTESIAN_POINT ( 'NONE',  ( 33.66666666666666430, 6.884901960086285300, 3.975000000000003642 ) ) ;
#72845=CARTESIAN_POINT ( 'NONE',  ( 58.18793019189811133, 6.110000000000002984, -1.637169565754156730 ) ) ;
#72872=CARTESIAN_POINT ( 'NONE',  ( 71.97502705046289861, -5.819803920172573086, 5.819803920172573086 ) ) ;
#72897=CARTESIAN_POINT ( 'NONE',  ( 92.66209685856479439, -5.291415217122919401, 3.054999999999997939 ) ) ;
#72901=DIRECTION ( 'NONE',  ( 0.000000000000000000, 0.000000000000000000, 1.000000000000000000 ) ) ;
#72906=VERTEX_POINT ( 'NONE', #106968 ) ;
#72920=CARTESIAN_POINT ( 'NONE',  ( 45.20876352523143993, -7.482591942790329030E-16, 6.110000000000001208 ) ) ;
#72965=CARTESIAN_POINT ( 'NONE',  ( 72.09959685856479439, -6.109999999999998543, -1.637169565754160727 ) ) ;
#72970=CARTESIAN_POINT ( 'NONE',  ( 0.000000000000000000, 0.000000000000000000, 0.000000000000000000 ) ) ;
#72987=CARTESIAN_POINT ( 'NONE',  ( 94.28752705046289861, 0.000000000000000000, -7.949999999999998401 ) ) ;
#73004=ADVANCED_FACE ( 'NONE', ( #83839 ), #28728, .T. ) ;
#73006=CARTESIAN_POINT ( 'NONE',  ( 85.31293019189811844, -1.637169565754159617, -6.110000000000001208 ) ) ;
#73024=CARTESIAN_POINT ( 'NONE',  ( 74.08376352523143282, -6.110000000000001208, -3.741295971395164515E-16 ) ) ;
#73073=CARTESIAN_POINT ( 'NONE',  ( 68.54209685856477563, 5.291415217122923842, -3.054999999999996163 ) ) ;
#73078=CARTESIAN_POINT ( 'NONE',  ( 110.9795968585647756, 6.109999999999999432, 1.637169565754164280 ) ) ;
#73083=EDGE_CURVE ( 'NONE', #136489, #133461, #11901, .T. ) ;
#73105=CARTESIAN_POINT ( 'NONE',  ( 12.28062291172085274, -8.652526378290415821, 3.924136651621471295 ) ) ;
#73121=CARTESIAN_POINT ( 'NONE',  ( 73.77083333333332860, -7.949999999999998401, -2.130196079827426203 ) ) ;
#73134=CARTESIAN_POINT ( 'NONE',  ( 122.8708603837962272, 6.884901960086289741, -3.974999999999993427 ) ) ;
#73153=CARTESIAN_POINT ( 'NONE',  ( 82.95833333333332860, 3.974999999999997424, 6.884901960086288852 ) ) ;
#73156=CARTESIAN_POINT ( 'NONE',  ( 92.10002705046288440, 5.819803920172570422, 5.819803920172575751 ) ) ;
#73179=CARTESIAN_POINT ( 'NONE',  ( 101.0629301918980900, 1.637169565754157174, 6.110000000000002984 ) ) ;
#73185=CARTESIAN_POINT ( 'NONE',  ( 74.79166666666667140, 3.975000000000003642, -6.884901960086285300 ) ) ;
#73187=CARTESIAN_POINT ( 'NONE',  ( 95.28709685856479439, 3.054999999999997495, 5.291415217122919401 ) ) ;
#73231=AXIS2_PLACEMENT_3D ( 'NONE', #133835, #13445, #80193 ) ;
#73232=CARTESIAN_POINT ( 'NONE',  ( 27.62043019189810877, 3.055000000000001936, -5.291415217122916737 ) ) ;
#73269=CARTESIAN_POINT ( 'NONE',  ( 100.8287635252314516, 0.000000000000000000, -6.109999999999999432 ) ) ;
#73305=CARTESIAN_POINT ( 'NONE',  ( 47.81249999999999289, 5.819803920172571310, 5.819803920172576639 ) ) ;
#73308=CARTESIAN_POINT ( 'NONE',  ( 26.99999999999999645, 5.837062628940091535, 2.500239961634333596 ) ) ;
#73317=CARTESIAN_POINT ( 'NONE',  ( 107.7500000000000000, -9.735942053221458872E-16, 7.950000000000000178 ) ) ;
#73325=( BOUNDED_CURVE ( )  B_SPLINE_CURVE ( 2, ( #50344, #127918, #38049, #16236, #27862, #40209, #28600, #116302, #18381, #51059, #61951, #139525, #61268 ),
 .UNSPECIFIED., .F., .T. ) 
 B_SPLINE_CURVE_WITH_KNOTS ( ( 3, 2, 2, 2, 2, 2, 3 ),
 ( 0.2666666666666666630, 0.2694444444444444309, 0.2722222222222221988, 0.2750000000000000222, 0.2777777777777777901, 0.2805555555555555580, 0.2833333333333333259 ),
 .UNSPECIFIED. ) 
 CURVE ( )  GEOMETRIC_REPRESENTATION_ITEM ( )  RATIONAL_B_SPLINE_CURVE ( ( 1.000000000000000000, 0.9659258262890683122, 1.000000000000000000, 0.9659258262890683122, 1.000000000000000000, 0.9659258262890683122, 1.000000000000000000, 0.9659258262890683122, 1.000000000000000000, 0.9659258262890683122, 1.000000000000000000, 0.9659258262890683122, 1.000000000000000000 ) ) 
 REPRESENTATION_ITEM ( '' )  );
#73332=CARTESIAN_POINT ( 'NONE',  ( 104.7087635252314328, -7.482591942790329030E-16, 6.110000000000001208 ) ) ;
#73340=CARTESIAN_POINT ( 'NONE',  ( 41.78752705046289151, 0.000000000000000000, -7.949999999999998401 ) ) ;
#73347=CARTESIAN_POINT ( 'NONE',  ( 126.1462635252314328, -4.472830434245840259, 4.472830434245839371 ) ) ;
#73357=CARTESIAN_POINT ( 'NONE',  ( 125.4745968585647944, 1.637169565754164058, -6.109999999999996767 ) ) ;
#73368=CARTESIAN_POINT ( 'NONE',  ( 49.14626352523143282, -4.472830434245840259, 4.472830434245839371 ) ) ;
#73371=LINE ( 'NONE', #130946, #25424 ) ;
#73380=CARTESIAN_POINT ( 'NONE',  ( 50.51626352523143737, -4.472830434245839371, 4.472830434245839371 ) ) ;
#73389=CARTESIAN_POINT ( 'NONE',  ( 60.01669371712956291, 7.950000000000000178, -2.130196079827421318 ) ) ;
#73402=CARTESIAN_POINT ( 'NONE',  ( 57.66209685856478728, -5.291415217122919401, 3.054999999999997939 ) ) ;
#73434=CARTESIAN_POINT ( 'NONE',  ( 127.8079301918981230, -6.109999999999999432, 1.637169565754158507 ) ) ;
#73443=CARTESIAN_POINT ( 'NONE',  ( 75.47502705046287019, -5.819803920172573086, 5.819803920172573086 ) ) ;
#73476=CARTESIAN_POINT ( 'NONE',  ( 48.47459685856478728, 1.637169565754164280, -6.109999999999997655 ) ) ;
#73490=CARTESIAN_POINT ( 'NONE',  ( 82.66666666666667140, 6.884901960086285300, 3.975000000000003642 ) ) ;
#73491=CARTESIAN_POINT ( 'NONE',  ( 126.8754301918981184, -5.291415217122920289, -3.055000000000001492 ) ) ;
#73493=EDGE_CURVE ( 'NONE', #98697, #83142, #26188, .T. ) ;
#73502=CARTESIAN_POINT ( 'NONE',  ( 63.95419371712955581, 6.884901960086283523, 3.975000000000002753 ) ) ;
#73507=CARTESIAN_POINT ( 'NONE',  ( 57.14583333333332860, 2.130196079827431976, -7.949999999999999289 ) ) ;
#73516=CARTESIAN_POINT ( 'NONE',  ( 58.62543019189810423, 5.291415217122919401, 3.055000000000002824 ) ) ;
#73541=CARTESIAN_POINT ( 'NONE',  ( 78.80793019189810877, -6.109999999999998543, 1.637169565754158063 ) ) ;
#73567=CARTESIAN_POINT ( 'NONE',  ( 86.39126352523145158, -4.472830434245838482, -4.472830434245838482 ) ) ;
#73590=CARTESIAN_POINT ( 'NONE',  ( 36.89626352523143993, 4.472830434245840259, -4.472830434245838482 ) ) ;
#73633=EDGE_CURVE ( 'NONE', #16751, #129366, #82711, .T. ) ;
#73639=CARTESIAN_POINT ( 'NONE',  ( 73.41209685856478018, 5.291415217122922066, -3.054999999999995275 ) ) ;
#73646=DIRECTION ( 'NONE',  ( 0.000000000000000000, 0.000000000000000000, 1.000000000000000000 ) ) ;
#73666=CARTESIAN_POINT ( 'NONE',  ( 95.45419371712957002, 6.884901960086283523, 3.975000000000002753 ) ) ;
#73678=CARTESIAN_POINT ( 'NONE',  ( 85.89626352523144703, 4.472830434245840259, -4.472830434245839371 ) ) ;
#73683=VECTOR ( 'NONE', #119084, 1000.000000000000000 ) ;
#73685=CARTESIAN_POINT ( 'NONE',  ( 118.0583603837962130, -7.949999999999996625, -2.130196079827426203 ) ) ;
#73697=CARTESIAN_POINT ( 'NONE',  ( 69.56293019189810423, 1.637169565754157174, 6.110000000000002984 ) ) ;
#73706=( BOUNDED_CURVE ( )  B_SPLINE_CURVE ( 2, ( #76714, #10675, #129619, #9989, #31754, #30320, #31056, #75971, #20856, #74558, #65117, #40504, #54255 ),
 .UNSPECIFIED., .F., .F. ) 
 B_SPLINE_CURVE_WITH_KNOTS ( ( 3, 2, 2, 2, 2, 2, 3 ),
 ( 0.7500000000000000000, 0.7527777777777777679, 0.7555555555555555358, 0.7583333333333333037, 0.7611111111111110716, 0.7638888888888888395, 0.7666666666666667185 ),
 .UNSPECIFIED. ) 
 CURVE ( )  GEOMETRIC_REPRESENTATION_ITEM ( )  RATIONAL_B_SPLINE_CURVE ( ( 1.000000000000000000, 0.9659258262890683122, 1.000000000000000000, 0.9659258262890683122, 1.000000000000000000, 0.9659258262890683122, 1.000000000000000000, 0.9659258262890683122, 1.000000000000000000, 0.9659258262890683122, 1.000000000000000000, 0.9659258262890683122, 1.000000000000000000 ) ) 
 REPRESENTATION_ITEM ( '' )  );
#73718=CARTESIAN_POINT ( 'NONE',  ( 53.60002705046289151, 5.819803920172570422, 5.819803920172575751 ) ) ;
#73729=CARTESIAN_POINT ( 'NONE',  ( 69.05836038379621300, -7.949999999999996625, -2.130196079827426203 ) ) ;
#73736=CARTESIAN_POINT ( 'NONE',  ( 27.00000000000000355, -4.083527258847093222, -4.862849486279972488 ) ) ;
#73739=CARTESIAN_POINT ( 'NONE',  ( 51.74999999999999289, -9.735942053221458872E-16, 7.950000000000000178 ) ) ;
#73749=CARTESIAN_POINT ( 'NONE',  ( 75.25043019189811844, 3.055000000000002824, -5.291415217122919401 ) ) ;
#73758=CARTESIAN_POINT ( 'NONE',  ( 112.2920968585647756, -5.291415217122921177, 3.054999999999999272 ) ) ;
#73764=CIRCLE ( 'NONE', #8820, 7.950000000000000178 ) ;
#73807=CARTESIAN_POINT ( 'NONE',  ( 32.08376352523143993, -6.110000000000001208, -3.741295971395164515E-16 ) ) ;
#73811=VERTEX_POINT ( 'NONE', #140633 ) ;
#73826=CARTESIAN_POINT ( 'NONE',  ( 120.2458603837962272, 3.974999999999996980, 6.884901960086287964 ) ) ;
#73839=CARTESIAN_POINT ( 'NONE',  ( 86.60416666666664298, 2.130196079827422206, 7.950000000000001954 ) ) ;
#73847=CARTESIAN_POINT ( 'NONE',  ( 31.28752705046289151, 0.000000000000000000, -7.949999999999998401 ) ) ;
#73852=LINE ( 'NONE', #93466, #139105 ) ;
#73856=EDGE_CURVE ( 'NONE', #76474, #10908, #35826, .T. ) ;
#73868=CARTESIAN_POINT ( 'NONE',  ( 104.2712635252314470, 4.472830434245839371, 4.472830434245842035 ) ) ;
#73879=CARTESIAN_POINT ( 'NONE',  ( 99.51626352523145158, -4.472830434245839371, 4.472830434245839371 ) ) ;
#73926=( BOUNDED_CURVE ( )  B_SPLINE_CURVE ( 2, ( #89810, #656, #78251, #34740, #33346, #76839, #112302, #121012, #99236, #44197, #77547, #22389, #122432 ),
 .UNSPECIFIED., .F., .T. ) 
 B_SPLINE_CURVE_WITH_KNOTS ( ( 3, 2, 2, 2, 2, 2, 3 ),
 ( 0.2000000000000000111, 0.2027777777777777790, 0.2055555555555555469, 0.2083333333333333426, 0.2111111111111111105, 0.2138888888888888784, 0.2166666666666666741 ),
 .UNSPECIFIED. ) 
 CURVE ( )  GEOMETRIC_REPRESENTATION_ITEM ( )  RATIONAL_B_SPLINE_CURVE ( ( 1.000000000000000000, 0.9659258262890683122, 1.000000000000000000, 0.9659258262890683122, 1.000000000000000000, 0.9659258262890683122, 1.000000000000000000, 0.9659258262890683122, 1.000000000000000000, 0.9659258262890683122, 1.000000000000000000, 0.9659258262890683122, 1.000000000000000000 ) ) 
 REPRESENTATION_ITEM ( '' )  );
#73928=CARTESIAN_POINT ( 'NONE',  ( 30.82876352523145158, 0.000000000000000000, -6.109999999999998543 ) ) ;
#73967=CARTESIAN_POINT ( 'NONE',  ( 94.26626352523143737, 4.472830434245839371, -4.472830434245839371 ) ) ;
#73982=CONICAL_SURFACE ( 'NONE', #134210, 7.950000000000000178, 0.7853981633974396193 ) ;
#74008=CARTESIAN_POINT ( 'NONE',  ( 48.10416666666665009, 2.130196079827422206, 7.950000000000001954 ) ) ;
#74019=CARTESIAN_POINT ( 'NONE',  ( 106.8750000000000000, 7.950000000000000178, 1.460391307983218535E-15 ) ) ;
#74031=CARTESIAN_POINT ( 'NONE',  ( 103.5420968585647756, 5.291415217122923842, -3.054999999999996163 ) ) ;
#74032=EDGE_CURVE ( 'NONE', #127835, #18455, #47395, .T. ) ;
#74044=CARTESIAN_POINT ( 'NONE',  ( 125.8545968585647756, -1.637169565754161615, 6.110000000000000320 ) ) ;
#74052=CARTESIAN_POINT ( 'NONE',  ( 121.0995968585647660, -6.109999999999997655, -1.637169565754160283 ) ) ;
#74062=FILL_AREA_STYLE_COLOUR ( '', #35176 ) ;
#74066=CARTESIAN_POINT ( 'NONE',  ( 41.41709685856477563, 3.054999999999998828, 5.291415217122922066 ) ) ;
#74075=CARTESIAN_POINT ( 'NONE',  ( 39.57876352523144448, -7.482591942790325086E-16, 6.109999999999998543 ) ) ;
#74104=EDGE_CURVE ( 'NONE', #74867, #134670, #80275, .T. ) ;
#74105=CARTESIAN_POINT ( 'NONE',  ( 58.39126352523145158, -4.472830434245838482, -4.472830434245838482 ) ) ;
#74129=CARTESIAN_POINT ( 'NONE',  ( 55.05836038379621300, -7.949999999999996625, -2.130196079827426203 ) ) ;
#74140=CARTESIAN_POINT ( 'NONE',  ( 121.0995968585647660, -6.109999999999998543, -1.637169565754160727 ) ) ;
#74182=CARTESIAN_POINT ( 'NONE',  ( 35.64126352523145158, 4.472830434245837594, 4.472830434245841147 ) ) ;
#74209=CARTESIAN_POINT ( 'NONE',  ( 60.60002705046288440, 5.819803920172570422, 5.819803920172574863 ) ) ;
#74214=CARTESIAN_POINT ( 'NONE',  ( 57.29166666666665719, 3.975000000000003642, -6.884901960086285300 ) ) ;
#74220=CARTESIAN_POINT ( 'NONE',  ( 32.93749999999999289, 5.819803920172574863, -5.819803920172573086 ) ) ;
#74221=CARTESIAN_POINT ( 'NONE',  ( 50.02126352523143282, -4.472830434245839371, -4.472830434245840259 ) ) ;
#74248=CARTESIAN_POINT ( 'NONE',  ( 71.51626352523145158, -4.472830434245839371, 4.472830434245839371 ) ) ;
#74277=CARTESIAN_POINT ( 'NONE',  ( 51.85002705046288440, -5.819803920172573086, -5.819803920172573086 ) ) ;
#74280=VERTEX_POINT ( 'NONE', #33870 ) ;
#74283=CARTESIAN_POINT ( 'NONE',  ( 83.32876352523143737, 0.000000000000000000, -6.109999999999998543 ) ) ;
#74292=CIRCLE ( 'NONE', #83518, 1.499999999999999556 ) ;
#74298=DIRECTION ( 'NONE',  ( -1.000000000000000000, -0.000000000000000000, -0.000000000000000000 ) ) ;
#74313=CARTESIAN_POINT ( 'NONE',  ( 40.39626352523143993, 4.472830434245840259, -4.472830434245838482 ) ) ;
#74324=AXIS2_PLACEMENT_3D ( 'NONE', #129475, #54800, #98979 ) ;
#74350=( BOUNDED_CURVE ( )  B_SPLINE_CURVE ( 2, ( #32987, #42428, #83229, #115806, #127432, #39747, #72396, #128177, #16516, #62203, #60804, #17250, #65624 ),
 .UNSPECIFIED., .F., .T. ) 
 B_SPLINE_CURVE_WITH_KNOTS ( ( 3, 2, 2, 2, 2, 2, 3 ),
 ( 0.1333333333333333315, 0.1361111111111110994, 0.1388888888888888951, 0.1416666666666666630, 0.1444444444444444309, 0.1472222222222222265, 0.1499999999999999944 ),
 .UNSPECIFIED. ) 
 CURVE ( )  GEOMETRIC_REPRESENTATION_ITEM ( )  RATIONAL_B_SPLINE_CURVE ( ( 1.000000000000000000, 0.9659258262890683122, 1.000000000000000000, 0.9659258262890683122, 1.000000000000000000, 0.9659258262890683122, 1.000000000000000000, 0.9659258262890683122, 1.000000000000000000, 0.9659258262890683122, 1.000000000000000000, 0.9659258262890683122, 1.000000000000000000 ) ) 
 REPRESENTATION_ITEM ( '' )  );
#74365=CARTESIAN_POINT ( 'NONE',  ( 62.62043019189811588, 3.055000000000002380, -5.291415217122917625 ) ) ;
#74394=CARTESIAN_POINT ( 'NONE',  ( 95.89169371712955581, 2.130196079827421762, 7.950000000000001066 ) ) ;
#74402=DIRECTION ( 'NONE',  ( -1.000000000000000000, -0.000000000000000000, -0.000000000000000000 ) ) ;
#74408=CARTESIAN_POINT ( 'NONE',  ( 71.16709685856477563, -3.055000000000000160, -5.291415217122921177 ) ) ;
#74417=EDGE_CURVE ( 'NONE', #75827, #113019, #136723, .T. ) ;
#74427=ORIENTED_EDGE ( 'NONE', *, *, #35510, .F. ) ;
#74428=CARTESIAN_POINT ( 'NONE',  ( 71.45876352523143282, 0.000000000000000000, -6.110000000000001208 ) ) ;
#74463=EDGE_CURVE ( 'NONE', #120796, #120211, #142467, .T. ) ;
#74485=CARTESIAN_POINT ( 'NONE',  ( 51.02083333333333570, 7.949999999999998401, 2.130196079827431532 ) ) ;
#74492=CARTESIAN_POINT ( 'NONE',  ( 60.81293019189811133, -1.637169565754159617, -6.110000000000001208 ) ) ;
#74498=CARTESIAN_POINT ( 'NONE',  ( 95.08376352523144703, -6.110000000000001208, -3.741295971395164515E-16 ) ) ;
#74540=CARTESIAN_POINT ( 'NONE',  ( 25.66709685856477563, -3.055000000000000160, -5.291415217122921177 ) ) ;
#74557=CARTESIAN_POINT ( 'NONE',  ( 118.2041937171295700, -6.884901960086285300, -3.975000000000000089 ) ) ;
#74558=CARTESIAN_POINT ( 'NONE',  ( 49.22502705046289151, 5.819803920172573974, -5.819803920172573086 ) ) ;
#74601=CARTESIAN_POINT ( 'NONE',  ( 100.9170968585647756, 3.054999999999998828, 5.291415217122922066 ) ) ;
#74610=CARTESIAN_POINT ( 'NONE',  ( 98.64126352523145158, 4.472830434245836706, 4.472830434245840259 ) ) ;
#74612=AXIS2_PLACEMENT_3D ( 'NONE', #143478, #122431, #121011 ) ;
#74666=CARTESIAN_POINT ( 'NONE',  ( 126.0004301918981042, -3.055000000000002380, 5.291415217122920289 ) ) ;
#74704=CARTESIAN_POINT ( 'NONE',  ( 87.55793019189812298, 6.110000000000001208, -1.637169565754156286 ) ) ;
#74754=CARTESIAN_POINT ( 'NONE',  ( 108.9166666666666572, -6.884901960086287076, -3.975000000000000977 ) ) ;
#74755=VERTEX_POINT ( 'NONE', #103910 ) ;
#74768=CARTESIAN_POINT ( 'NONE',  ( 105.7295968585647898, -6.110000000000000320, -1.637169565754161393 ) ) ;
#74782=CARTESIAN_POINT ( 'NONE',  ( 29.58333333333332149, 6.884901960086290629, -3.974999999999994316 ) ) ;
#74797=CARTESIAN_POINT ( 'NONE',  ( 120.2245968585648086, -1.637169565754160949, 6.109999999999997655 ) ) ;
#74803=CARTESIAN_POINT ( 'NONE',  ( 70.51669371712954160, 7.950000000000000178, -2.130196079827421318 ) ) ;
#74809=CARTESIAN_POINT ( 'NONE',  ( 46.22959685856476852, -6.110000000000000320, -1.637169565754161393 ) ) ;
#74816=CARTESIAN_POINT ( 'NONE',  ( 39.72459685856478018, -1.637169565754160949, 6.109999999999997655 ) ) ;
#74844=CARTESIAN_POINT ( 'NONE',  ( 55.47459685856477307, 1.637169565754164280, -6.109999999999996767 ) ) ;
#74853=CYLINDRICAL_SURFACE ( 'NONE', #124596, 7.950000000000000178 ) ;
#74867=VERTEX_POINT ( 'NONE', #130719 ) ;
#74880=CARTESIAN_POINT ( 'NONE',  ( 119.3495968585647944, 6.109999999999997655, 1.637169565754163836 ) ) ;
#74912=CARTESIAN_POINT ( 'NONE',  ( 0.000000000000000000, 1.163414459189985682E-15, -9.500000000000001776 ) ) ;
#74921=CARTESIAN_POINT ( 'NONE',  ( 33.59959685856477307, -6.109999999999998543, -1.637169565754160727 ) ) ;
#74946=CARTESIAN_POINT ( 'NONE',  ( 53.30836038379623432, 7.949999999999997513, 2.130196079827431088 ) ) ;
#74952=CARTESIAN_POINT ( 'NONE',  ( 55.83333333333332860, -6.884901960086287964, 3.974999999999998312 ) ) ;
#74962=CARTESIAN_POINT ( 'NONE',  ( 50.60459685856477563, 1.637169565754164946, -6.109999999999999432 ) ) ;
#74974=CARTESIAN_POINT ( 'NONE',  ( 93.75000000000000000, -9.735942053221458872E-16, 7.950000000000000178 ) ) ;
#74977=CARTESIAN_POINT ( 'NONE',  ( 82.83376352523144703, 6.110000000000001208, 1.122388791418549305E-15 ) ) ;
#74986=CARTESIAN_POINT ( 'NONE',  ( 63.20376352523145158, 6.109999999999998543, 1.122388791418548911E-15 ) ) ;
#74997=VERTEX_POINT ( 'NONE', #53106 ) ;
#75015=CARTESIAN_POINT ( 'NONE',  ( 88.72459685856478018, -1.637169565754160949, 6.109999999999997655 ) ) ;
#75043=CARTESIAN_POINT ( 'NONE',  ( 33.39626352523143993, 4.472830434245840259, -4.472830434245838482 ) ) ;
#75063=CARTESIAN_POINT ( 'NONE',  ( 108.5791937171295700, 3.975000000000002753, -6.884901960086283523 ) ) ;
#75066=VERTEX_POINT ( 'NONE', #132862 ) ;
#75094=CARTESIAN_POINT ( 'NONE',  ( 64.07876352523145158, -7.482591942790327058E-16, 6.109999999999999432 ) ) ;
#75118=CARTESIAN_POINT ( 'NONE',  ( 89.03752705046288440, -9.735942053221456900E-16, 7.949999999999998401 ) ) ;
#75136=CARTESIAN_POINT ( 'NONE',  ( 77.29209685856477563, -5.291415217122921177, 3.054999999999999272 ) ) ;
#75139=VERTEX_POINT ( 'NONE', #32092 ) ;
#75157=CARTESIAN_POINT ( 'NONE',  ( 64.75043019189810423, 3.055000000000002824, -5.291415217122919401 ) ) ;
#75188=CARTESIAN_POINT ( 'NONE',  ( 111.4745968585647802, 1.637169565754164280, -6.109999999999996767 ) ) ;
#75209=CARTESIAN_POINT ( 'NONE',  ( 61.39626352523142572, 4.472830434245840259, -4.472830434245838482 ) ) ;
#75215=CARTESIAN_POINT ( 'NONE',  ( 97.12543019189810423, 5.291415217122919401, 3.055000000000002824 ) ) ;
#75230=CARTESIAN_POINT ( 'NONE',  ( 118.1829301918981230, -1.637169565754158951, -6.109999999999998543 ) ) ;
#75258=CARTESIAN_POINT ( 'NONE',  ( 28.72959685856476497, -6.110000000000000320, -1.637169565754161393 ) ) ;
#75267=DIRECTION ( 'NONE',  ( -1.000000000000000000, -0.000000000000000000, -0.000000000000000000 ) ) ;
#75275=CARTESIAN_POINT ( 'NONE',  ( 113.8291937171295558, -3.975000000000001865, 6.884901960086284411 ) ) ;
#75290=DIRECTION ( 'NONE',  ( 0.000000000000000000, 0.000000000000000000, 1.000000000000000000 ) ) ;
#75305=CARTESIAN_POINT ( 'NONE',  ( 69.83333333333332860, -6.884901960086287964, 3.974999999999998312 ) ) ;
#75310=VERTEX_POINT ( 'NONE', #5676 ) ;
#75312=CARTESIAN_POINT ( 'NONE',  ( 106.1670968585647756, -3.055000000000000160, -5.291415217122921177 ) ) ;
#75322=CARTESIAN_POINT ( 'NONE',  ( 97.03709685856479439, -3.054999999999998828, -5.291415217122919401 ) ) ;
#75335=DIRECTION ( 'NONE',  ( 0.000000000000000000, 0.000000000000000000, 1.000000000000000000 ) ) ;
#75349=CARTESIAN_POINT ( 'NONE',  ( 61.03752705046289151, -9.735942053221456900E-16, 7.949999999999998401 ) ) ;
#75351=CARTESIAN_POINT ( 'NONE',  ( 55.39583333333331439, -2.130196079827351596, 7.950000000000043698 ) ) ;
#75367=CARTESIAN_POINT ( 'NONE',  ( 27.76626352523143737, 4.472830434245838482, -4.472830434245837594 ) ) ;
#75400=CARTESIAN_POINT ( 'NONE',  ( 95.72459685856476597, -1.637169565754161171, 6.109999999999998543 ) ) ;
#75401=CARTESIAN_POINT ( 'NONE',  ( 7.431334631360206444, -8.913301243404507801, -3.293706071196084384 ) ) ;
#75419=DIRECTION ( 'NONE',  ( -1.000000000000000000, -0.000000000000000000, -0.000000000000000000 ) ) ;
#75438=CARTESIAN_POINT ( 'NONE',  ( 32.06249999999999289, -5.819803920172573086, -5.819803920172573974 ) ) ;
#75453=CARTESIAN_POINT ( 'NONE',  ( 112.7083333333333286, -3.974999999999999201, -6.884901960086287964 ) ) ;
#75466=CARTESIAN_POINT ( 'NONE',  ( 99.31293019189810423, -1.637169565754159617, -6.110000000000001208 ) ) ;
#75474=CARTESIAN_POINT ( 'NONE',  ( 31.14169371712956291, -2.130196079827424871, -7.949999999999999289 ) ) ;
#75478=CARTESIAN_POINT ( 'NONE',  ( 25.49999999999999645, 0.000000000000000000, -7.950000000000000178 ) ) ;
#75486=CARTESIAN_POINT ( 'NONE',  ( 119.2037635252314658, 6.109999999999998543, 1.122388791418548911E-15 ) ) ;
#75496=CARTESIAN_POINT ( 'NONE',  ( 47.97959685856477563, 6.109999999999999432, 1.637169565754164280 ) ) ;
#75504=CARTESIAN_POINT ( 'NONE',  ( 35.78709685856478018, 3.054999999999997495, 5.291415217122919401 ) ) ;
#75513=CARTESIAN_POINT ( 'NONE',  ( 79.55836038379622721, -7.949999999999996625, -2.130196079827426203 ) ) ;
#75530=ORIENTED_EDGE ( 'NONE', *, *, #43024, .F. ) ;
#75536=CARTESIAN_POINT ( 'NONE',  ( 56.93293019189810877, 1.637169565754156508, 6.110000000000000320 ) ) ;
#75544=CARTESIAN_POINT ( 'NONE',  ( 0.000000000000000000, 0.000000000000000000, 0.000000000000000000 ) ) ;
#75574=CARTESIAN_POINT ( 'NONE',  ( 123.1412635252314374, 4.472830434245837594, 4.472830434245841147 ) ) ;
#75581=CARTESIAN_POINT ( 'NONE',  ( 66.87086038379622721, 6.884901960086289741, -3.974999999999993427 ) ) ;
#75612=CARTESIAN_POINT ( 'NONE',  ( 126.5282023469572152, -6.688762929388991196, -1.806560149088825895 ) ) ;
#75613=CARTESIAN_POINT ( 'NONE',  ( 39.28709685856478018, 3.054999999999997939, 5.291415217122920289 ) ) ;
#75625=ORIENTED_EDGE ( 'NONE', *, *, #111236, .T. ) ;
#75630=CARTESIAN_POINT ( 'NONE',  ( 82.95833333333332860, 3.974999999999997424, 6.884901960086288852 ) ) ;
#75642=CARTESIAN_POINT ( 'NONE',  ( 55.20419371712956291, -6.884901960086285300, -3.975000000000000089 ) ) ;
#75647=CARTESIAN_POINT ( 'NONE',  ( 58.75000000000000000, -9.735942053221458872E-16, 7.950000000000000178 ) ) ;
#75655=CARTESIAN_POINT ( 'NONE',  ( 43.02126352523142572, -4.472830434245839371, -4.472830434245840259 ) ) ;
#75664=ORIENTED_EDGE ( 'NONE', *, *, #24678, .T. ) ;
#75669=CARTESIAN_POINT ( 'NONE',  ( 82.54209685856478984, 5.291415217122923842, -3.054999999999996163 ) ) ;
#75679=CARTESIAN_POINT ( 'NONE',  ( 68.74543019189812298, -5.291415217122918513, -3.055000000000000160 ) ) ;
#75710=CARTESIAN_POINT ( 'NONE',  ( 81.72459685856476597, -1.637169565754160949, 6.109999999999997655 ) ) ;
#75732=CARTESIAN_POINT ( 'NONE',  ( 32.37543019189810423, -5.291415217122920289, -3.055000000000001492 ) ) ;
#75734=CARTESIAN_POINT ( 'NONE',  ( 92.53752705046289861, -9.735942053221456900E-16, 7.949999999999998401 ) ) ;
#75744=FACE_OUTER_BOUND ( 'NONE', #6708, .T. ) ;
#75790=CARTESIAN_POINT ( 'NONE',  ( 62.47459685856478018, 1.637169565754164280, -6.109999999999997655 ) ) ;
#75816=CARTESIAN_POINT ( 'NONE',  ( 84.51669371712955581, 7.950000000000001066, -2.130196079827421318 ) ) ;
#75827=VERTEX_POINT ( 'NONE', #85223 ) ;
#75829=CARTESIAN_POINT ( 'NONE',  ( 72.47959685856478984, 6.109999999999999432, 1.637169565754164280 ) ) ;
#75850=CARTESIAN_POINT ( 'NONE',  ( 63.43793019189811133, -6.110000000000001208, 1.637169565754158951 ) ) ;
#75872=CARTESIAN_POINT ( 'NONE',  ( 62.10416666666666430, 2.130196079827422206, 7.950000000000001954 ) ) ;
#75879=CARTESIAN_POINT ( 'NONE',  ( 114.3912635252314374, -4.472830434245838482, -4.472830434245838482 ) ) ;
#75898=CARTESIAN_POINT ( 'NONE',  ( 59.50043019189810423, -3.055000000000002380, 5.291415217122920289 ) ) ;
#75904=CARTESIAN_POINT ( 'NONE',  ( 104.2712635252314470, 4.472830434245838482, 4.472830434245842035 ) ) ;
#75921=CARTESIAN_POINT ( 'NONE',  ( 118.0370968585647802, -3.054999999999998828, -5.291415217122919401 ) ) ;
#75928=ADVANCED_FACE ( 'NONE', ( #66360 ), #123612, .T. ) ;
#75931=VERTEX_POINT ( 'NONE', #100411 ) ;
#75942=ADVANCED_FACE ( 'NONE', ( #67067 ), #57635, .T. ) ;
#75947=CARTESIAN_POINT ( 'NONE',  ( 32.66709685856476852, -3.055000000000000160, -5.291415217122921177 ) ) ;
#75955=ORIENTED_EDGE ( 'NONE', *, *, #79741, .T. ) ;
#75962=ORIENTED_EDGE ( 'NONE', *, *, #107835, .F. ) ;
#75970=CARTESIAN_POINT ( 'NONE',  ( 115.8708603837962414, 6.884901960086289741, -3.974999999999993427 ) ) ;
#75971=CARTESIAN_POINT ( 'NONE',  ( 49.51669371712954870, 7.950000000000000178, -2.130196079827421318 ) ) ;
#76001=CARTESIAN_POINT ( 'NONE',  ( 70.12500000000000000, -7.950000000000000178, -4.867971026610729436E-16 ) ) ;
#76008=CARTESIAN_POINT ( 'NONE',  ( 93.33376352523144703, 6.110000000000001208, 1.122388791418549305E-15 ) ) ;
#76017=CARTESIAN_POINT ( 'NONE',  ( 97.47459685856478018, 1.637169565754164058, -6.109999999999996767 ) ) ;
#76043=EDGE_LOOP ( 'NONE', ( #142051, #118071, #120271, #62642 ) ) ;
#76069=ORIENTED_EDGE ( 'NONE', *, *, #48435, .F. ) ;
#76075=CARTESIAN_POINT ( 'NONE',  ( 126.2920968585647614, -5.291415217122921177, 3.054999999999999272 ) ) ;
#76107=CARTESIAN_POINT ( 'NONE',  ( 91.78709685856478018, 3.054999999999997939, 5.291415217122920289 ) ) ;
#76128=EDGE_CURVE ( 'NONE', #133461, #7223, #11624, .T. ) ;
#76162=CARTESIAN_POINT ( 'NONE',  ( 97.68750000000000000, -5.819803920172573086, 5.819803920172572198 ) ) ;
#76187=CARTESIAN_POINT ( 'NONE',  ( 29.39169371712956291, 2.130196079827421762, 7.950000000000001066 ) ) ;
#76191=CARTESIAN_POINT ( 'NONE',  ( 124.6879301918981042, 6.110000000000002984, -1.637169565754156730 ) ) ;
#76198=CARTESIAN_POINT ( 'NONE',  ( 125.6204301918981088, 3.055000000000001936, -5.291415217122916737 ) ) ;
#76206=CARTESIAN_POINT ( 'NONE',  ( 42.58376352523143993, -6.110000000000001208, -3.741295971395164515E-16 ) ) ;
#76215=CARTESIAN_POINT ( 'NONE',  ( 42.05793019189811588, 6.110000000000000320, -1.637169565754156064 ) ) ;
#76249=CARTESIAN_POINT ( 'NONE',  ( 51.82876352523144448, 0.000000000000000000, -6.109999999999998543 ) ) ;
#76254=ORIENTED_EDGE ( 'NONE', *, *, #79132, .F. ) ;
#76258=( BOUNDED_CURVE ( )  B_SPLINE_CURVE ( 2, ( #134525, #66411, #34483, #54821, #99002, #143238, #78000, #43936, #110582, #11261, #114855, #4631, #82986 ),
 .UNSPECIFIED., .F., .F. ) 
 B_SPLINE_CURVE_WITH_KNOTS ( ( 3, 2, 2, 2, 2, 2, 3 ),
 ( 0.03607035673769710266, 0.03611111111111108690, 0.03888888888888748091, 0.04166666666666386798, 0.04444444444444026199, 0.04722222222221665600, 0.04999999999999305000 ),
 .UNSPECIFIED. ) 
 CURVE ( )  GEOMETRIC_REPRESENTATION_ITEM ( )  RATIONAL_B_SPLINE_CURVE ( ( 0.9990148257276658672, 0.9995000782242919879, 1.000000000000000000, 0.9659258262890683122, 1.000000000000000000, 0.9659258262890683122, 1.000000000000000000, 0.9659258262890683122, 1.000000000000000000, 0.9659258262890683122, 1.000000000000000000, 0.9659258262891535773, 0.9999999999999147349 ) ) 
 REPRESENTATION_ITEM ( '' )  );
#76261=CARTESIAN_POINT ( 'NONE',  ( 116.5000000000000000, 0.000000000000000000, -7.950000000000000178 ) ) ;
#76290=CARTESIAN_POINT ( 'NONE',  ( 120.3704301918981230, -3.055000000000001936, 5.291415217122918513 ) ) ;
#76297=CARTESIAN_POINT ( 'NONE',  ( 66.28752705046289861, 0.000000000000000000, -7.949999999999998401 ) ) ;
#76309=EDGE_LOOP ( 'NONE', ( #41093, #82134, #106007, #24076 ) ) ;
#76321=EDGE_LOOP ( 'NONE', ( #54403, #35944, #10299, #79636, #80766, #50638, #137420 ) ) ;
#76326=CARTESIAN_POINT ( 'NONE',  ( 40.30793019189810877, -6.109999999999999432, 1.637169565754158507 ) ) ;
#76339=CARTESIAN_POINT ( 'NONE',  ( 128.8287635252314658, 0.000000000000000000, -6.109999999999998543 ) ) ;
#76352=CARTESIAN_POINT ( 'NONE',  ( 56.66252705046289151, 7.949999999999998401, 1.460391307983218338E-15 ) ) ;
#76358=CARTESIAN_POINT ( 'NONE',  ( 58.02083333333331439, 7.949999999999999289, 2.130196079827431532 ) ) ;
#76361=CIRCLE ( 'NONE', #13809, 8.000000000000001776 ) ;
#76367=CARTESIAN_POINT ( 'NONE',  ( 50.75043019189810423, 3.055000000000002824, -5.291415217122919401 ) ) ;
#76387=CARTESIAN_POINT ( 'NONE',  ( 83.41709685856477563, 3.054999999999998828, 5.291415217122922066 ) ) ;
#76398=CARTESIAN_POINT ( 'NONE',  ( 68.89126352523142316, -4.472830434245839371, -4.472830434245839371 ) ) ;
#76407=DIRECTION ( 'NONE',  ( 0.000000000000000000, 0.000000000000000000, 1.000000000000000000 ) ) ;
#76423=CARTESIAN_POINT ( 'NONE',  ( 52.28752705046288440, 0.000000000000000000, -7.949999999999998401 ) ) ;
#76429=CARTESIAN_POINT ( 'NONE',  ( 87.84959685856478018, 6.109999999999996767, 1.637169565754163836 ) ) ;
#76451=CARTESIAN_POINT ( 'NONE',  ( 122.2875270504628844, 0.000000000000000000, -7.949999999999998401 ) ) ;
#76458=CARTESIAN_POINT ( 'NONE',  ( 36.31293019189809712, -1.637169565754159617, -6.110000000000001208 ) ) ;
#76461=CARTESIAN_POINT ( 'NONE',  ( 45.77083333333332149, -7.949999999999998401, -2.130196079827426203 ) ) ;
#76463=CARTESIAN_POINT ( 'NONE',  ( 90.20419371712957002, -6.884901960086285300, -3.975000000000000089 ) ) ;
#76474=VERTEX_POINT ( 'NONE', #47338 ) ;
#76490=DIRECTION ( 'NONE',  ( 0.2419218955996628451, 0.000000000000000000, -0.9702957262759975832 ) ) ;
#76496=CARTESIAN_POINT ( 'NONE',  ( 97.20419371712955581, -6.884901960086285300, -3.975000000000000089 ) ) ;
#76511=CARTESIAN_POINT ( 'NONE',  ( 53.06250000000000000, -5.819803920172573086, -5.819803920172573974 ) ) ;
#76513=CARTESIAN_POINT ( 'NONE',  ( 68.45376352523143737, -6.109999999999999432, -3.741295971395163529E-16 ) ) ;
#76540=CARTESIAN_POINT ( 'NONE',  ( 86.55836038379621300, -7.949999999999997513, -2.130196079827425759 ) ) ;
#76544=CARTESIAN_POINT ( 'NONE',  ( 83.97916666666665719, -7.950000000000001066, 2.130196079827424427 ) ) ;
#76553=CARTESIAN_POINT ( 'NONE',  ( 78.89626352523143282, 4.472830434245840259, -4.472830434245839371 ) ) ;
#76578=CARTESIAN_POINT ( 'NONE',  ( 62.70876352523143993, -7.482591942790329030E-16, 6.110000000000001208 ) ) ;
#76607=CARTESIAN_POINT ( 'NONE',  ( 60.64583333333332860, 2.130196079827431976, -7.949999999999998401 ) ) ;
#76614=CARTESIAN_POINT ( 'NONE',  ( 108.1204301918981230, 3.055000000000001936, -5.291415217122916737 ) ) ;
#76636=CARTESIAN_POINT ( 'NONE',  ( 65.62543019189810423, 5.291415217122919401, 3.055000000000002824 ) ) ;
#76642=CARTESIAN_POINT ( 'NONE',  ( 102.9587635252314470, 0.000000000000000000, -6.110000000000001208 ) ) ;
#76654=LINE ( 'NONE', #44008, #50677 ) ;
#76658=ORIENTED_EDGE ( 'NONE', *, *, #14540, .T. ) ;
#76659=CARTESIAN_POINT ( 'NONE',  ( 120.0787635252314516, -7.482591942790325086E-16, 6.109999999999998543 ) ) ;
#76676=CARTESIAN_POINT ( 'NONE',  ( 39.06250000000000000, -5.819803920172573086, -5.819803920172573974 ) ) ;
#76689=CARTESIAN_POINT ( 'NONE',  ( 33.25043019189810423, 3.055000000000002824, -5.291415217122919401 ) ) ;
#76701=ORIENTED_EDGE ( 'NONE', *, *, #67174, .F. ) ;
#76713=CARTESIAN_POINT ( 'NONE',  ( 108.1416937171295700, -2.130196079827424871, -7.949999999999999289 ) ) ;
#76714=CARTESIAN_POINT ( 'NONE',  ( 50.53752705046289861, -9.735942053221456900E-16, 7.949999999999998401 ) ) ;
#76750=CARTESIAN_POINT ( 'NONE',  ( 95.22959685856474721, -6.110000000000000320, -1.637169565754161393 ) ) ;
#76763=CARTESIAN_POINT ( 'NONE',  ( 85.37043019189812298, -3.055000000000001492, 5.291415217122917625 ) ) ;
#76799=EDGE_CURVE ( 'NONE', #54290, #19121, #72033, .T. ) ;
#76818=CARTESIAN_POINT ( 'NONE',  ( 124.8337635252314470, 6.110000000000001208, 1.122388791418549305E-15 ) ) ;
#76839=CARTESIAN_POINT ( 'NONE',  ( 107.5583603837962414, -7.949999999999996625, -2.130196079827426203 ) ) ;
#76850=CARTESIAN_POINT ( 'NONE',  ( 86.24543019189812298, -5.291415217122919401, -3.055000000000000604 ) ) ;
#76889=CARTESIAN_POINT ( 'NONE',  ( 30.75000000000000000, -9.735942053221458872E-16, 7.950000000000000178 ) ) ;
#76892=FACE_OUTER_BOUND ( 'NONE', #44577, .T. ) ;
#76902=CARTESIAN_POINT ( 'NONE',  ( 104.5416666666666714, -3.975000000000002753, 6.884901960086286188 ) ) ;
#76922=CARTESIAN_POINT ( 'NONE',  ( 32.74586038379622011, 3.974999999999996980, 6.884901960086287964 ) ) ;
#76927=CARTESIAN_POINT ( 'NONE',  ( 123.9587635252314470, 0.000000000000000000, -6.110000000000001208 ) ) ;
#76939=CARTESIAN_POINT ( 'NONE',  ( 115.1204301918981230, 3.055000000000001936, -5.291415217122916737 ) ) ;
#76947=CARTESIAN_POINT ( 'NONE',  ( 38.06293019189810423, 1.637169565754157174, 6.110000000000002984 ) ) ;
#76955=CARTESIAN_POINT ( 'NONE',  ( 37.24543019189811588, -5.291415217122918513, -3.055000000000000160 ) ) ;
#76990=CARTESIAN_POINT ( 'NONE',  ( 48.62043019189811588, 3.055000000000001936, -5.291415217122916737 ) ) ;
#77020=CARTESIAN_POINT ( 'NONE',  ( 116.1412635252314374, 4.472830434245837594, 4.472830434245841147 ) ) ;
#77060=CARTESIAN_POINT ( 'NONE',  ( 37.53709685856478018, -3.054999999999999272, -5.291415217122919401 ) ) ;
#77079=CARTESIAN_POINT ( 'NONE',  ( 117.6879301918981184, 6.110000000000002984, -1.637169565754156730 ) ) ;
#77089=CARTESIAN_POINT ( 'NONE',  ( 61.03752705046289151, -9.735942053221456900E-16, 7.949999999999998401 ) ) ;
#77095=CARTESIAN_POINT ( 'NONE',  ( 45.47916666666665719, -7.950000000000001066, 2.130196079827424427 ) ) ;
#77105=CARTESIAN_POINT ( 'NONE',  ( 35.14626352523143993, -4.472830434245840259, 4.472830434245839371 ) ) ;
#77122=CARTESIAN_POINT ( 'NONE',  ( 78.31293019189811844, -1.637169565754159617, -6.110000000000001208 ) ) ;
#77131=CARTESIAN_POINT ( 'NONE',  ( 63.93293019189812298, 1.637169565754156508, 6.110000000000000320 ) ) ;
#77155=CARTESIAN_POINT ( 'NONE',  ( 0.000000000000000000, 0.000000000000000000, 0.000000000000000000 ) ) ;
#77162=CARTESIAN_POINT ( 'NONE',  ( 73.26626352523143737, 4.472830434245838482, -4.472830434245837594 ) ) ;
#77170=CARTESIAN_POINT ( 'NONE',  ( 121.8958333333333286, -2.130196079827399558, 7.950000000000016165 ) ) ;
#77185=CARTESIAN_POINT ( 'NONE',  ( 28.43793019189810423, -6.110000000000001208, 1.637169565754158951 ) ) ;
#77236=CARTESIAN_POINT ( 'NONE',  ( 111.6875000000000000, -5.819803920172573974, 5.819803920172573086 ) ) ;
#77241=CARTESIAN_POINT ( 'NONE',  ( 62.18293019189812298, -1.637169565754159173, -6.109999999999999432 ) ) ;
#77253=EDGE_CURVE ( 'NONE', #36177, #77939, #109196, .T. ) ;
#77266=CARTESIAN_POINT ( 'NONE',  ( 86.85002705046289861, -5.819803920172572198, -5.819803920172572198 ) ) ;
#77271=CARTESIAN_POINT ( 'NONE',  ( 71.87500000000000000, 7.950000000000000178, 1.460391307983218535E-15 ) ) ;
#77282=CARTESIAN_POINT ( 'NONE',  ( 76.41709685856476142, 3.054999999999998828, 5.291415217122922066 ) ) ;
#77292=CARTESIAN_POINT ( 'NONE',  ( 127.0000000000000000, 1.664417612029487348, 6.163512901498443775 ) ) ;
#77301=CARTESIAN_POINT ( 'NONE',  ( 63.00043019189810423, -3.055000000000002380, 5.291415217122920289 ) ) ;
#77331=( BOUNDED_CURVE ( )  B_SPLINE_CURVE ( 2, ( #86462, #110308, #31360, #130689, #107475, #63986, #118340, #108156, #75581, #119751, #43651, #97275, #76297 ),
 .UNSPECIFIED., .F., .T. ) 
 B_SPLINE_CURVE_WITH_KNOTS ( ( 3, 2, 2, 2, 2, 2, 3 ),
 ( 0.5833333333333333703, 0.5861111111111111382, 0.5888888888888889062, 0.5916666666666666741, 0.5944444444444444420, 0.5972222222222222099, 0.5999999999999999778 ),
 .UNSPECIFIED. ) 
 CURVE ( )  GEOMETRIC_REPRESENTATION_ITEM ( )  RATIONAL_B_SPLINE_CURVE ( ( 1.000000000000000000, 0.9659258262890683122, 1.000000000000000000, 0.9659258262890683122, 1.000000000000000000, 0.9659258262890683122, 1.000000000000000000, 0.9659258262890683122, 1.000000000000000000, 0.9659258262890683122, 1.000000000000000000, 0.9659258262890683122, 1.000000000000000000 ) ) 
 REPRESENTATION_ITEM ( '' )  );
#77338=CARTESIAN_POINT ( 'NONE',  ( 100.0995968585647944, -6.109999999999997655, -1.637169565754160283 ) ) ;
#77349=LINE ( 'NONE', #27022, #98253 ) ;
#77357=CARTESIAN_POINT ( 'NONE',  ( 88.06249999999998579, -5.819803920172573086, -5.819803920172573974 ) ) ;
#77363=CARTESIAN_POINT ( 'NONE',  ( 68.25043019189810423, 3.055000000000002824, -5.291415217122919401 ) ) ;
#77368=CARTESIAN_POINT ( 'NONE',  ( 96.68793019189811844, 6.110000000000002984, -1.637169565754156730 ) ) ;
#77381=CARTESIAN_POINT ( 'NONE',  ( 125.3287635252314516, 0.000000000000000000, -6.109999999999998543 ) ) ;
#77420=FACE_OUTER_BOUND ( 'NONE', #103991, .T. ) ;
#77432=CARTESIAN_POINT ( 'NONE',  ( 117.0375270504628986, -9.735942053221456900E-16, 7.949999999999998401 ) ) ;
#77468=CARTESIAN_POINT ( 'NONE',  ( 96.54209685856477563, 5.291415217122923842, -3.054999999999996163 ) ) ;
#77473=ORIENTED_EDGE ( 'NONE', *, *, #48435, .T. ) ;
#77475=CARTESIAN_POINT ( 'NONE',  ( 48.54166666666666430, -3.975000000000002753, 6.884901960086286188 ) ) ;
#77477=CARTESIAN_POINT ( 'NONE',  ( 85.95376352523145158, -6.109999999999998543, -3.741295971395162543E-16 ) ) ;
#77482=EDGE_LOOP ( 'NONE', ( #106559, #3796, #136122, #55896 ) ) ;
#77514=ORIENTED_EDGE ( 'NONE', *, *, #16859, .F. ) ;
#77547=CARTESIAN_POINT ( 'NONE',  ( 106.8291937171295700, -3.975000000000001865, 6.884901960086284411 ) ) ;
#77557=CARTESIAN_POINT ( 'NONE',  ( 81.14126352523143737, 4.472830434245837594, 4.472830434245841147 ) ) ;
#77559=CARTESIAN_POINT ( 'NONE',  ( 5.949495903232621785, -9.500232149547882088, -0.2856502682321572784 ) ) ;
#77606=CARTESIAN_POINT ( 'NONE',  ( 104.3958333333333428, -2.130196079827427091, 7.949999999999999289 ) ) ;
#77613=CARTESIAN_POINT ( 'NONE',  ( 88.93750000000000000, 5.819803920172574863, -5.819803920172573086 ) ) ;
#77633=CARTESIAN_POINT ( 'NONE',  ( 119.1462635252314470, -4.472830434245840259, 4.472830434245839371 ) ) ;
#77642=CARTESIAN_POINT ( 'NONE',  ( 117.7454301918981230, -5.291415217122918513, -3.055000000000000160 ) ) ;
#77647=CARTESIAN_POINT ( 'NONE',  ( 97.83333333333332860, -6.884901960086287964, 3.974999999999998312 ) ) ;
#77650=CARTESIAN_POINT ( 'NONE',  ( 39.22959685856475431, -6.110000000000000320, -1.637169565754161393 ) ) ;
#77656=CARTESIAN_POINT ( 'NONE',  ( 28.20376352523144803, 6.109999999999998543, 1.122388791418548911E-15 ) ) ;
#77684=CARTESIAN_POINT ( 'NONE',  ( 44.53709685856478728, -3.054999999999998828, -5.291415217122919401 ) ) ;
#77717=CARTESIAN_POINT ( 'NONE',  ( 107.0995968585648086, -6.109999999999998543, -1.637169565754160727 ) ) ;
#77755=DIRECTION ( 'NONE',  ( -1.000000000000000000, -0.000000000000000000, -0.000000000000000000 ) ) ;
#77759=CARTESIAN_POINT ( 'NONE',  ( 26.59959685856477307, -6.109999999999998543, -1.637169565754160727 ) ) ;
#77772=FACE_OUTER_BOUND ( 'NONE', #122981, .T. ) ;
#77774=CARTESIAN_POINT ( 'NONE',  ( 126.4379301918981042, -6.110000000000001208, 1.637169565754158951 ) ) ;
#77783=CARTESIAN_POINT ( 'NONE',  ( 47.03752705046289151, -9.735942053221456900E-16, 7.949999999999998401 ) ) ;
#77789=VERTEX_POINT ( 'NONE', #3384 ) ;
#77790=CARTESIAN_POINT ( 'NONE',  ( 40.95833333333333570, 3.974999999999997424, 6.884901960086288852 ) ) ;
#77797=CARTESIAN_POINT ( 'NONE',  ( 37.62543019189811133, 5.291415217122919401, 3.055000000000002824 ) ) ;
#77810=CARTESIAN_POINT ( 'NONE',  ( 83.27126352523143282, 4.472830434245838482, 4.472830434245842035 ) ) ;
#77819=CARTESIAN_POINT ( 'NONE',  ( 60.87043019189810877, -3.055000000000001492, 5.291415217122917625 ) ) ;
#77827=SURFACE_SIDE_STYLE ('',( #122011 ) ) ;
#77839=FACE_OUTER_BOUND ( 'NONE', #10964, .T. ) ;
#77845=CARTESIAN_POINT ( 'NONE',  ( 78.80793019189810877, -6.109999999999998543, 1.637169565754158507 ) ) ;
#77933=CARTESIAN_POINT ( 'NONE',  ( 58.24543019189810877, -5.291415217122919401, -3.055000000000000604 ) ) ;
#77939=VERTEX_POINT ( 'NONE', #65502 ) ;
#77955=CARTESIAN_POINT ( 'NONE',  ( 87.28752705046288440, 0.000000000000000000, -7.949999999999998401 ) ) ;
#77961=CARTESIAN_POINT ( 'NONE',  ( 69.83333333333332860, -6.884901960086287964, 3.974999999999998312 ) ) ;
#77972=CARTESIAN_POINT ( 'NONE',  ( 66.64626352523144703, -4.472830434245840259, 4.472830434245839371 ) ) ;
#77975=ORIENTED_EDGE ( 'NONE', *, *, #41029, .T. ) ;
#77981=CARTESIAN_POINT ( 'NONE',  ( 43.58333333333333570, 6.884901960086290629, -3.974999999999994316 ) ) ;
#77989=ORIENTED_EDGE ( 'NONE', *, *, #3551, .F. ) ;
#77992=CARTESIAN_POINT ( 'NONE',  ( 68.10459685856474721, 1.637169565754164946, -6.109999999999999432 ) ) ;
#78000=CARTESIAN_POINT ( 'NONE',  ( 124.9125270504628986, -7.949999999999998401, -4.867971026610728450E-16 ) ) ;
#78001=CARTESIAN_POINT ( 'NONE',  ( 54.95833333333332860, 3.974999999999997424, 6.884901960086288852 ) ) ;
#78008=CARTESIAN_POINT ( 'NONE',  ( 113.5375270504628986, -9.735942053221456900E-16, 7.949999999999998401 ) ) ;
#78028=CARTESIAN_POINT ( 'NONE',  ( 101.5579301918981088, 6.110000000000000320, -1.637169565754156064 ) ) ;
#78053=CARTESIAN_POINT ( 'NONE',  ( 53.37543019189811133, -5.291415217122920289, -3.055000000000001492 ) ) ;
#78060=CARTESIAN_POINT ( 'NONE',  ( 91.29209685856477563, -5.291415217122921177, 3.054999999999999272 ) ) ;
#78077=CARTESIAN_POINT ( 'NONE',  ( 125.0370968585647944, -3.054999999999998828, -5.291415217122919401 ) ) ;
#78099=CARTESIAN_POINT ( 'NONE',  ( 7.033036791254640541, 9.050499037475331576, 2.895286894036863679 ) ) ;
#78105=LINE ( 'NONE', #123760, #104366 ) ;
#78110=CARTESIAN_POINT ( 'NONE',  ( 41.83333333333333570, -6.884901960086287964, 3.974999999999998312 ) ) ;
#78126=CARTESIAN_POINT ( 'NONE',  ( 113.1000270504628986, 5.819803920172570422, 5.819803920172574863 ) ) ;
#78141=CARTESIAN_POINT ( 'NONE',  ( 91.00043019189810423, -3.055000000000002380, 5.291415217122920289 ) ) ;
#78153=EDGE_LOOP ( 'NONE', ( #135932, #36145, #113901, #141077 ) ) ;
#78164=CARTESIAN_POINT ( 'NONE',  ( 90.85459685856477563, -1.637169565754161615, 6.110000000000000320 ) ) ;
#78171=CARTESIAN_POINT ( 'NONE',  ( 85.10002705046289861, 5.819803920172570422, 5.819803920172575751 ) ) ;
#78176=CARTESIAN_POINT ( 'NONE',  ( 81.43293019189809456, 1.637169565754156508, 6.110000000000000320 ) ) ;
#78208=FACE_OUTER_BOUND ( 'NONE', #110050, .T. ) ;
#78217=CARTESIAN_POINT ( 'NONE',  ( 115.5791937171295558, 3.975000000000002753, -6.884901960086283523 ) ) ;
#78229=CARTESIAN_POINT ( 'NONE',  ( 119.8754301918981184, -5.291415217122920289, -3.055000000000001492 ) ) ;
#78251=CARTESIAN_POINT ( 'NONE',  ( 107.9958603837962272, -3.974999999999998312, -6.884901960086286188 ) ) ;
#78261=CARTESIAN_POINT ( 'NONE',  ( 86.39126352523146579, -4.472830434245839371, -4.472830434245839371 ) ) ;
#78264=CARTESIAN_POINT ( 'NONE',  ( 99.39169371712955581, 2.130196079827421762, 7.950000000000000178 ) ) ;
#78305=CARTESIAN_POINT ( 'NONE',  ( 103.3750000000000000, 7.950000000000000178, 1.460391307983218535E-15 ) ) ;
#78328=CARTESIAN_POINT ( 'NONE',  ( 86.85002705046289861, -5.819803920172573086, -5.819803920172573086 ) ) ;
#78332=CARTESIAN_POINT ( 'NONE',  ( 120.4587635252314328, 0.000000000000000000, -6.110000000000001208 ) ) ;
#78338=CARTESIAN_POINT ( 'NONE',  ( 112.6412635252314658, 4.472830434245836706, 4.472830434245840259 ) ) ;
#78349=CARTESIAN_POINT ( 'NONE',  ( 40.39626352523143993, 4.472830434245840259, -4.472830434245839371 ) ) ;
#78355=CARTESIAN_POINT ( 'NONE',  ( 28.49543019189811233, 5.291415217122916737, 3.055000000000001936 ) ) ;
#78389=CARTESIAN_POINT ( 'NONE',  ( 51.53709685856478018, -3.054999999999998828, -5.291415217122919401 ) ) ;
#78399=FACE_OUTER_BOUND ( 'NONE', #66339, .T. ) ;
#78423=CARTESIAN_POINT ( 'NONE',  ( 114.2454301918981230, -5.291415217122919401, -3.055000000000000604 ) ) ;
#78469=CARTESIAN_POINT ( 'NONE',  ( 28.05793019189811233, 6.110000000000001208, -1.637169565754156286 ) ) ;
#78484=CARTESIAN_POINT ( 'NONE',  ( 120.7504301918981184, 3.055000000000002824, -5.291415217122919401 ) ) ;
#78493=CARTESIAN_POINT ( 'NONE',  ( 44.55836038379621300, -7.949999999999997513, -2.130196079827425759 ) ) ;
#78498=CARTESIAN_POINT ( 'NONE',  ( 44.16666666666665719, 6.884901960086285300, 3.975000000000003642 ) ) ;
#78505=CARTESIAN_POINT ( 'NONE',  ( 40.39626352523143993, 4.472830434245840259, -4.472830434245839371 ) ) ;
#78532=CARTESIAN_POINT ( 'NONE',  ( 59.70376352523145158, 6.109999999999998543, 1.122388791418548911E-15 ) ) ;
#78566=CARTESIAN_POINT ( 'NONE',  ( 71.80793019189810877, -6.109999999999998543, 1.637169565754158507 ) ) ;
#78586=CARTESIAN_POINT ( 'NONE',  ( 26.10459685856476852, 1.637169565754164946, -6.109999999999999432 ) ) ;
#78608=CARTESIAN_POINT ( 'NONE',  ( 27.39583333333332504, -2.130196079827427091, 7.949999999999998401 ) ) ;
#78638=CARTESIAN_POINT ( 'NONE',  ( 59.55793019189812298, 6.110000000000001208, -1.637169565754156286 ) ) ;
#78639=LINE ( 'NONE', #143172, #53382 ) ;
#78663=CARTESIAN_POINT ( 'NONE',  ( 71.53752705046289861, -9.735942053221456900E-16, 7.949999999999998401 ) ) ;
#78667=CARTESIAN_POINT ( 'NONE',  ( 72.89583333333331439, -2.130196079827427091, 7.949999999999999289 ) ) ;
#78669=CYLINDRICAL_SURFACE ( 'NONE', #81684, 7.950000000000000178 ) ;
#78677=CARTESIAN_POINT ( 'NONE',  ( 62.27126352523142572, 4.472830434245839371, 4.472830434245842035 ) ) ;
#78694=CARTESIAN_POINT ( 'NONE',  ( 53.52126352523144703, -4.472830434245839371, -4.472830434245840259 ) ) ;
#78730=CARTESIAN_POINT ( 'NONE',  ( 104.3287635252314658, 0.000000000000000000, -6.109999999999998543 ) ) ;
#78734=VERTEX_POINT ( 'NONE', #15857 ) ;
#78749=CARTESIAN_POINT ( 'NONE',  ( 27.64169371712955936, -2.130196079827424871, -7.949999999999998401 ) ) ;
#78760=CARTESIAN_POINT ( 'NONE',  ( 58.62543019189810423, 5.291415217122919401, 3.055000000000002824 ) ) ;
#78768=CARTESIAN_POINT ( 'NONE',  ( 92.02126352523143282, -4.472830434245838482, -4.472830434245840259 ) ) ;
#78809=CARTESIAN_POINT ( 'NONE',  ( 6.851954622386678295, 9.118668024956557261, 2.675793564507496836 ) ) ;
#78843=CARTESIAN_POINT ( 'NONE',  ( 99.10002705046288440, 5.819803920172570422, 5.819803920172574863 ) ) ;
#78863=CARTESIAN_POINT ( 'NONE',  ( 98.14626352523144703, -4.472830434245840259, 4.472830434245839371 ) ) ;
#78889=CARTESIAN_POINT ( 'NONE',  ( 94.79209685856476142, -5.291415217122921177, 3.054999999999999272 ) ) ;
#78904=CARTESIAN_POINT ( 'NONE',  ( 86.09959685856478018, -6.109999999999997655, -1.637169565754160283 ) ) ;
#78932=CARTESIAN_POINT ( 'NONE',  ( 56.37086038379622721, 6.884901960086289741, -3.974999999999993427 ) ) ;
#78953=ADVANCED_FACE ( 'NONE', ( #123813 ), #113614, .T. ) ;
#78958=CARTESIAN_POINT ( 'NONE',  ( 119.1462635252314470, -4.472830434245840259, 4.472830434245838482 ) ) ;
#78990=CARTESIAN_POINT ( 'NONE',  ( 83.91209685856479439, 5.291415217122922066, -3.054999999999995275 ) ) ;
#79016=CARTESIAN_POINT ( 'NONE',  ( 121.7500000000000000, -9.735942053221458872E-16, 7.950000000000000178 ) ) ;
#79027=( BOUNDED_CURVE ( )  B_SPLINE_CURVE ( 2, ( #110401, #118433, #51784 ),
 .UNSPECIFIED., .F., .T. ) 
 B_SPLINE_CURVE_WITH_KNOTS ( ( 3, 3 ),
 ( 0.01666666666666434884, 0.01798785857039796043 ),
 .UNSPECIFIED. ) 
 CURVE ( )  GEOMETRIC_REPRESENTATION_ITEM ( )  RATIONAL_B_SPLINE_CURVE ( ( 1.000000000000028422, 0.9837933319240432795, 0.9830033892749372448 ) ) 
 REPRESENTATION_ITEM ( '' )  );
#79048=CARTESIAN_POINT ( 'NONE',  ( 100.4583333333333286, 3.974999999999997424, 6.884901960086288852 ) ) ;
#79066=CARTESIAN_POINT ( 'NONE',  ( 127.0787635252314516, -7.482591942790325086E-16, 6.109999999999998543 ) ) ;
#79078=CARTESIAN_POINT ( 'NONE',  ( 123.0837635252314470, -6.110000000000001208, -3.741295971395164515E-16 ) ) ;
#79088=CARTESIAN_POINT ( 'NONE',  ( 112.4954301918981230, 5.291415217122916737, 3.055000000000001936 ) ) ;
#79113=DIRECTION ( 'NONE',  ( -1.000000000000000000, -0.000000000000000000, -0.000000000000000000 ) ) ;
#79123=CYLINDRICAL_SURFACE ( 'NONE', #101246, 7.950000000000000178 ) ;
#79132=EDGE_CURVE ( 'NONE', #9583, #94004, #66552, .T. ) ;
#79133=CARTESIAN_POINT ( 'NONE',  ( 48.03709685856477307, -3.054999999999998828, -5.291415217122919401 ) ) ;
#79171=CARTESIAN_POINT ( 'NONE',  ( 106.5162635252314658, -4.472830434245839371, 4.472830434245839371 ) ) ;
#79183=CARTESIAN_POINT ( 'NONE',  ( 121.7500000000000000, -9.735942053221458872E-16, 7.950000000000000178 ) ) ;
#79239=CARTESIAN_POINT ( 'NONE',  ( 123.6670968585647756, -3.055000000000000160, -5.291415217122921177 ) ) ;
#79250=CARTESIAN_POINT ( 'NONE',  ( 50.24586038379622011, 3.974999999999996980, 6.884901960086287964 ) ) ;
#79255=CARTESIAN_POINT ( 'NONE',  ( 47.95833333333332860, 3.974999999999997424, 6.884901960086288852 ) ) ;
#79266=CARTESIAN_POINT ( 'NONE',  ( 34.27126352523143993, 4.472830434245839371, 4.472830434245842035 ) ) ;
#79283=CARTESIAN_POINT ( 'NONE',  ( 0.000000000000000000, 9.735942053221458872E-16, -7.950000000000000178 ) ) ;
#79288=CARTESIAN_POINT ( 'NONE',  ( 55.62043019189812298, 3.055000000000001936, -5.291415217122916737 ) ) ;
#79300=ORIENTED_EDGE ( 'NONE', *, *, #97260, .F. ) ;
#79313=DIRECTION ( 'NONE',  ( 0.000000000000000000, 0.000000000000000000, -1.000000000000000000 ) ) ;
#79314=VERTEX_POINT ( 'NONE', #124327 ) ;
#79318=CARTESIAN_POINT ( 'NONE',  ( 77.93293019189812298, 1.637169565754156508, 6.110000000000000320 ) ) ;
#79322=AXIS2_PLACEMENT_3D ( 'NONE', #41612, #53954, #76407 ) ;
#79327=CARTESIAN_POINT ( 'NONE',  ( 123.3541666666666856, -2.130196079827445299, -7.949999999999990408 ) ) ;
#79348=CARTESIAN_POINT ( 'NONE',  ( 42.80836038379622011, 7.949999999999996625, 2.130196079827431088 ) ) ;
#79398=CARTESIAN_POINT ( 'NONE',  ( 55.62043019189812298, 3.055000000000002380, -5.291415217122917625 ) ) ;
#79418=ORIENTED_EDGE ( 'NONE', *, *, #70196, .F. ) ;
#79424=CARTESIAN_POINT ( 'NONE',  ( 117.3750000000000000, 7.950000000000000178, 1.460391307983218535E-15 ) ) ;
#79425=CARTESIAN_POINT ( 'NONE',  ( 74.89169371712957002, 2.130196079827421762, 7.950000000000001066 ) ) ;
#79430=CARTESIAN_POINT ( 'NONE',  ( 71.00000000000000000, 0.000000000000000000, -7.950000000000000178 ) ) ;
#79440=CARTESIAN_POINT ( 'NONE',  ( 64.45876352523144703, 0.000000000000000000, -6.110000000000001208 ) ) ;
#79449=CARTESIAN_POINT ( 'NONE',  ( 86.16666666666667140, 6.884901960086285300, 3.975000000000003642 ) ) ;
#79459=CARTESIAN_POINT ( 'NONE',  ( 54.10459685856476852, 1.637169565754164946, -6.109999999999999432 ) ) ;
#79493=CARTESIAN_POINT ( 'NONE',  ( 102.1412635252314374, 4.472830434245835818, 4.472830434245840259 ) ) ;
#79512=CARTESIAN_POINT ( 'NONE',  ( 87.47916666666664298, -7.950000000000000178, 2.130196079827424427 ) ) ;
#79520=CARTESIAN_POINT ( 'NONE',  ( 50.16709685856476852, -3.055000000000000160, -5.291415217122921177 ) ) ;
#79526=CARTESIAN_POINT ( 'NONE',  ( 87.79209685856477563, -5.291415217122921177, 3.054999999999999272 ) ) ;
#79538=CARTESIAN_POINT ( 'NONE',  ( 126.6412635252314516, 4.472830434245837594, 4.472830434245841147 ) ) ;
#79563=CARTESIAN_POINT ( 'NONE',  ( 56.99999999999999289, 0.000000000000000000, -7.950000000000000178 ) ) ;
#79579=EDGE_LOOP ( 'NONE', ( #130529, #29310 ) ) ;
#79595=CARTESIAN_POINT ( 'NONE',  ( 106.3916937171295700, 2.130196079827421762, 7.950000000000001066 ) ) ;
#79612=CARTESIAN_POINT ( 'NONE',  ( 92.02126352523143282, -4.472830434245839371, -4.472830434245840259 ) ) ;
#79631=CARTESIAN_POINT ( 'NONE',  ( 102.3083603837962130, 7.949999999999996625, 2.130196079827431088 ) ) ;
#79636=ORIENTED_EDGE ( 'NONE', *, *, #65832, .F. ) ;
#79640=CARTESIAN_POINT ( 'NONE',  ( 83.56293019189811844, 1.637169565754157174, 6.110000000000002984 ) ) ;
#79649=CARTESIAN_POINT ( 'NONE',  ( 102.5000000000000142, 0.000000000000000000, -7.950000000000000178 ) ) ;
#79652=CARTESIAN_POINT ( 'NONE',  ( 75.30793019189809456, -6.109999999999998543, 1.637169565754158063 ) ) ;
#79676=CARTESIAN_POINT ( 'NONE',  ( 57.53752705046289151, -9.735942053221456900E-16, 7.949999999999998401 ) ) ;
#79684=FACE_OUTER_BOUND ( 'NONE', #17990, .T. ) ;
#79694=CARTESIAN_POINT ( 'NONE',  ( 94.33333333333332860, -6.884901960086287964, 3.974999999999998312 ) ) ;
#79698=CARTESIAN_POINT ( 'NONE',  ( 120.1670968585647756, -3.055000000000000160, -5.291415217122921177 ) ) ;
#79729=CARTESIAN_POINT ( 'NONE',  ( 84.78709685856478018, 3.054999999999997939, 5.291415217122920289 ) ) ;
#79741=EDGE_CURVE ( 'NONE', #96308, #49442, #28954, .T. ) ;
#79778=CARTESIAN_POINT ( 'NONE',  ( 87.62500000000001421, -7.950000000000000178, -4.867971026610729436E-16 ) ) ;
#79789=CARTESIAN_POINT ( 'NONE',  ( 126.5612402446580944, 6.599829397831250333, 1.990250523215890688 ) ) ;
#79790=CARTESIAN_POINT ( 'NONE',  ( 128.5370968585647802, -3.054999999999998828, -5.291415217122919401 ) ) ;
#79806=CARTESIAN_POINT ( 'NONE',  ( 108.9379301918981042, -6.110000000000001208, 1.637169565754158951 ) ) ;
#79809=CARTESIAN_POINT ( 'NONE',  ( 100.7500000000000000, -9.735942053221458872E-16, 7.950000000000000178 ) ) ;
#79813=CARTESIAN_POINT ( 'NONE',  ( 112.9329301918981230, 1.637169565754156508, 6.110000000000000320 ) ) ;
#79827=CARTESIAN_POINT ( 'NONE',  ( 30.82876352523145158, 0.000000000000000000, -6.109999999999998543 ) ) ;
#79858=CARTESIAN_POINT ( 'NONE',  ( 40.01626352523143737, -4.472830434245838482, 4.472830434245838482 ) ) ;
#79882=VERTEX_POINT ( 'NONE', #31807 ) ;
#79892=CARTESIAN_POINT ( 'NONE',  ( 111.4745968585647944, 1.637169565754164280, -6.109999999999997655 ) ) ;
#79927=EDGE_CURVE ( 'NONE', #106661, #20647, #109291, .T. ) ;
#79938=CARTESIAN_POINT ( 'NONE',  ( 123.7916666666666714, 3.975000000000003642, -6.884901960086285300 ) ) ;
#79949=CARTESIAN_POINT ( 'NONE',  ( 120.1670968585647756, -3.055000000000000160, -5.291415217122921177 ) ) ;
#79959=CARTESIAN_POINT ( 'NONE',  ( 45.87086038379622721, 6.884901960086289741, -3.974999999999993427 ) ) ;
#79965=CARTESIAN_POINT ( 'NONE',  ( 42.12499999999999289, -7.950000000000000178, -4.867971026610729436E-16 ) ) ;
#79974=CARTESIAN_POINT ( 'NONE',  ( 38.06293019189810423, 1.637169565754157174, 6.110000000000002984 ) ) ;
#79979=CARTESIAN_POINT ( 'NONE',  ( 27.24999999999999645, -9.735942053221458872E-16, 7.950000000000000178 ) ) ;
#79993=CARTESIAN_POINT ( 'NONE',  ( 57.07876352523144448, -7.482591942790325086E-16, 6.109999999999998543 ) ) ;
#80025=CARTESIAN_POINT ( 'NONE',  ( 77.64126352523146579, 4.472830434245835818, 4.472830434245840259 ) ) ;
#80048=APPLICATION_CONTEXT ( 'automotive_design' ) ;
#80049=CARTESIAN_POINT ( 'NONE',  ( 29.16709685856476497, -3.055000000000000160, -5.291415217122921177 ) ) ;
#80071=CARTESIAN_POINT ( 'NONE',  ( 28.41666666666666075, -6.884901960086287076, -3.975000000000000977 ) ) ;
#80093=CARTESIAN_POINT ( 'NONE',  ( 54.01626352523143737, -4.472830434245839371, 4.472830434245839371 ) ) ;
#80115=CARTESIAN_POINT ( 'NONE',  ( 71.10002705046289861, 5.819803920172570422, 5.819803920172574863 ) ) ;
#80121=CARTESIAN_POINT ( 'NONE',  ( 71.43749999999998579, 5.819803920172573974, -5.819803920172572198 ) ) ;
#80133=CARTESIAN_POINT ( 'NONE',  ( 66.20876352523144703, -7.482591942790329030E-16, 6.110000000000001208 ) ) ;
#80142=CARTESIAN_POINT ( 'NONE',  ( 86.31249999999998579, 5.819803920172571310, 5.819803920172576639 ) ) ;
#80150=CARTESIAN_POINT ( 'NONE',  ( 58.47959685856477563, 6.109999999999999432, 1.637169565754164280 ) ) ;
#80180=CARTESIAN_POINT ( 'NONE',  ( 103.3079301918980946, -6.109999999999998543, 1.637169565754158507 ) ) ;
#80193=DIRECTION ( 'NONE',  ( 0.000000000000000000, 0.000000000000000000, 1.000000000000000000 ) ) ;
#80208=CARTESIAN_POINT ( 'NONE',  ( 56.29209685856477563, -5.291415217122921177, 3.054999999999999272 ) ) ;
#80215=CARTESIAN_POINT ( 'NONE',  ( 89.39626352523144703, 4.472830434245840259, -4.472830434245838482 ) ) ;
#80226=CARTESIAN_POINT ( 'NONE',  ( 125.3287635252314516, 0.000000000000000000, -6.109999999999999432 ) ) ;
#80243=( BOUNDED_CURVE ( )  B_SPLINE_CURVE ( 2, ( #91744, #57019, #101193, #135970, #36646, #1831, #90318, #12744, #59851, #112097, #3967, #57722, #25051 ),
 .UNSPECIFIED., .F., .T. ) 
 B_SPLINE_CURVE_WITH_KNOTS ( ( 3, 2, 2, 2, 2, 2, 3 ),
 ( 0.5500000000000000444, 0.5527777777777778123, 0.5555555555555555802, 0.5583333333333333481, 0.5611111111111111160, 0.5638888888888888840, 0.5666666666666666519 ),
 .UNSPECIFIED. ) 
 CURVE ( )  GEOMETRIC_REPRESENTATION_ITEM ( )  RATIONAL_B_SPLINE_CURVE ( ( 1.000000000000000000, 0.9659258262890683122, 1.000000000000000000, 0.9659258262890683122, 1.000000000000000000, 0.9659258262890683122, 1.000000000000000000, 0.9659258262890683122, 1.000000000000000000, 0.9659258262890683122, 1.000000000000000000, 0.9659258262890683122, 1.000000000000000000 ) ) 
 REPRESENTATION_ITEM ( '' )  );
#80275=( BOUNDED_CURVE ( )  B_SPLINE_CURVE ( 2, ( #43316, #20101, #141172, #76676, #41886, #86101, #31020, #8483, #119405, #18667, #87525, #64346, #131753 ),
 .UNSPECIFIED., .F., .F. ) 
 B_SPLINE_CURVE_WITH_KNOTS ( ( 3, 2, 2, 2, 2, 2, 3 ),
 ( 0.8333333333333334814, 0.8361111111111112493, 0.8388888888888890172, 0.8416666666666667851, 0.8444444444444445530, 0.8472222222222223209, 0.8500000000000000888 ),
 .UNSPECIFIED. ) 
 CURVE ( )  GEOMETRIC_REPRESENTATION_ITEM ( )  RATIONAL_B_SPLINE_CURVE ( ( 0.9999999999999986677, 0.9659258262890696445, 1.000000000000000000, 0.9659258262890683122, 1.000000000000000000, 0.9659258262890683122, 1.000000000000000000, 0.9659258262890683122, 1.000000000000000000, 0.9659258262890683122, 1.000000000000000000, 0.9659258262890669799, 1.000000000000001332 ) ) 
 REPRESENTATION_ITEM ( '' )  );
#80278=CARTESIAN_POINT ( 'NONE',  ( 100.2666937171295842, -7.949999999999999289, 2.130196079827424427 ) ) ;
#80295=CARTESIAN_POINT ( 'NONE',  ( 96.68793019189811844, 6.110000000000002984, -1.637169565754156730 ) ) ;
#80310=EDGE_LOOP ( 'NONE', ( #11076, #134157, #14289, #93867 ) ) ;
#80312=CARTESIAN_POINT ( 'NONE',  ( 102.8916937171295416, 2.130196079827421762, 7.950000000000000178 ) ) ;
#80322=CARTESIAN_POINT ( 'NONE',  ( 80.79209685856477563, -5.291415217122921177, 3.054999999999999272 ) ) ;
#80334=CARTESIAN_POINT ( 'NONE',  ( 75.45376352523145158, -6.109999999999998543, -3.741295971395162543E-16 ) ) ;
#80383=CARTESIAN_POINT ( 'NONE',  ( 120.8962635252314470, 4.472830434245840259, -4.472830434245838482 ) ) ;
#80398=CARTESIAN_POINT ( 'NONE',  ( 113.2916666666666714, 3.975000000000003642, -6.884901960086285300 ) ) ;
#80459=CARTESIAN_POINT ( 'NONE',  ( 89.95833333333332860, 3.974999999999997424, 6.884901960086288852 ) ) ;
#80467=CARTESIAN_POINT ( 'NONE',  ( 14.67146220324653250, 9.486753480112833259, 0.5775628020821772513 ) ) ;
#80474=CARTESIAN_POINT ( 'NONE',  ( 126.9329301918981088, 1.637169565754156508, 6.110000000000000320 ) ) ;
#80485=CARTESIAN_POINT ( 'NONE',  ( 107.0420968585647756, 5.291415217122923842, -3.054999999999996163 ) ) ;
#80489=CARTESIAN_POINT ( 'NONE',  ( 99.00000000000000000, 0.000000000000000000, -7.950000000000000178 ) ) ;
#80494=CARTESIAN_POINT ( 'NONE',  ( 103.5995968585647802, -6.109999999999997655, -1.637169565754160283 ) ) ;
#80509=CARTESIAN_POINT ( 'NONE',  ( 27.62043019189810877, 3.055000000000001936, -5.291415217122916737 ) ) ;
#80530=CARTESIAN_POINT ( 'NONE',  ( 63.22502705046288440, 5.819803920172573974, -5.819803920172573086 ) ) ;
#80540=CARTESIAN_POINT ( 'NONE',  ( 37.68293019189810167, -1.637169565754158951, -6.109999999999998543 ) ) ;
#80565=CARTESIAN_POINT ( 'NONE',  ( 153.6500000000000057, 0.000000000000000000, 6.349999999999997868 ) ) ;
#80576=CARTESIAN_POINT ( 'NONE',  ( 110.4537635252314516, -6.109999999999999432, -3.741295971395163529E-16 ) ) ;
#80590=CARTESIAN_POINT ( 'NONE',  ( 121.6041666666666714, 2.130196079827450628, 7.949999999999986855 ) ) ;
#80622=CARTESIAN_POINT ( 'NONE',  ( 117.0833333333333286, 6.884901960086290629, -3.974999999999994316 ) ) ;
#80633=CARTESIAN_POINT ( 'NONE',  ( 114.0420968585647898, 5.291415217122923842, -3.054999999999996163 ) ) ;
#80637=CARTESIAN_POINT ( 'NONE',  ( 106.3916937171295558, 2.130196079827421762, 7.950000000000000178 ) ) ;
#80645=CARTESIAN_POINT ( 'NONE',  ( 46.89169371712956291, 2.130196079827421762, 7.950000000000001066 ) ) ;
#80651=CARTESIAN_POINT ( 'NONE',  ( 39.35416666666665719, -2.130196079827425315, -7.950000000000001066 ) ) ;
#80663=CARTESIAN_POINT ( 'NONE',  ( 26.25043019189810067, 3.055000000000002824, -5.291415217122919401 ) ) ;
#80682=CARTESIAN_POINT ( 'NONE',  ( 61.74543019189811588, -5.291415217122918513, -3.055000000000000160 ) ) ;
#80717=CARTESIAN_POINT ( 'NONE',  ( 62.32876352523145158, 0.000000000000000000, -6.109999999999998543 ) ) ;
#80766=ORIENTED_EDGE ( 'NONE', *, *, #116429, .T. ) ;
#80775=CARTESIAN_POINT ( 'NONE',  ( 120.0000000000000000, 0.000000000000000000, -7.950000000000000178 ) ) ;
#80785=CARTESIAN_POINT ( 'NONE',  ( 59.12043019189810877, 3.055000000000002380, -5.291415217122917625 ) ) ;
#80789=ORIENTED_EDGE ( 'NONE', *, *, #139695, .T. ) ;
#80801=AXIS2_PLACEMENT_3D ( 'NONE', #44908, #97798, #99197 ) ;
#80817=CARTESIAN_POINT ( 'NONE',  ( 73.87086038379622721, 6.884901960086289741, -3.974999999999993427 ) ) ;
#80821=CARTESIAN_POINT ( 'NONE',  ( 64.29166666666665719, 3.975000000000003642, -6.884901960086285300 ) ) ;
#80832=CARTESIAN_POINT ( 'NONE',  ( 68.68793019189809002, 6.110000000000002984, -1.637169565754156730 ) ) ;
#80841=CARTESIAN_POINT ( 'NONE',  ( 44.02083333333332860, 7.949999999999998401, 2.130196079827431532 ) ) ;
#80846=DIRECTION ( 'NONE',  ( -1.000000000000000000, -0.000000000000000000, -0.000000000000000000 ) ) ;
#80875=DIRECTION ( 'NONE',  ( -1.000000000000000000, -0.000000000000000000, -0.000000000000000000 ) ) ;
#80881=CARTESIAN_POINT ( 'NONE',  ( 90.03709685856478018, -3.054999999999998828, -5.291415217122919401 ) ) ;
#80903=CARTESIAN_POINT ( 'NONE',  ( 43.89626352523143282, 4.472830434245840259, -4.472830434245838482 ) ) ;
#80954=CARTESIAN_POINT ( 'NONE',  ( 7.435109797308763646, 8.912112549869320333, -3.296747536672480550 ) ) ;
#80976=CARTESIAN_POINT ( 'NONE',  ( 102.0166937171295558, 7.950000000000001066, -2.130196079827421318 ) ) ;
#80994=CARTESIAN_POINT ( 'NONE',  ( 95.22959685856474721, -6.110000000000000320, -1.637169565754161393 ) ) ;
#81018=FACE_OUTER_BOUND ( 'NONE', #37493, .T. ) ;
#81022=CARTESIAN_POINT ( 'NONE',  ( 87.06293019189807580, 1.637169565754157174, 6.110000000000002984 ) ) ;
#81034=CARTESIAN_POINT ( 'NONE',  ( 75.74543019189810877, -5.291415217122918513, -3.055000000000000160 ) ) ;
#81084=CARTESIAN_POINT ( 'NONE',  ( 94.62500000000000000, -7.950000000000000178, -4.867971026610729436E-16 ) ) ;
#81086=CARTESIAN_POINT ( 'NONE',  ( 115.7920968585647756, -5.291415217122921177, 3.054999999999999272 ) ) ;
#81120=CARTESIAN_POINT ( 'NONE',  ( 98.80836038379622721, 7.949999999999996625, 2.130196079827431088 ) ) ;
#81129=EDGE_LOOP ( 'NONE', ( #96298, #85122, #76701, #133174 ) ) ;
#81145=CARTESIAN_POINT ( 'NONE',  ( 105.1250000000000000, -7.950000000000000178, -4.867971026610729436E-16 ) ) ;
#81150=CARTESIAN_POINT ( 'NONE',  ( 29.95376352523145158, -6.109999999999999432, -3.741295971395163529E-16 ) ) ;
#81169=CARTESIAN_POINT ( 'NONE',  ( 93.31249999999997158, 5.819803920172571310, 5.819803920172575751 ) ) ;
#81175=DIRECTION ( 'NONE',  ( 0.000000000000000000, 0.000000000000000000, 1.000000000000000000 ) ) ;
#81181=CARTESIAN_POINT ( 'NONE',  ( 125.5994534179081796, -2.266258037075818077, -7.520521262005186003 ) ) ;
#81196=CARTESIAN_POINT ( 'NONE',  ( 109.9587635252314470, 0.000000000000000000, -6.110000000000001208 ) ) ;
#81197=ORIENTED_EDGE ( 'NONE', *, *, #130159, .T. ) ;
#81207=CARTESIAN_POINT ( 'NONE',  ( 102.8704301918981230, -3.055000000000001492, 5.291415217122917625 ) ) ;
#81257=CARTESIAN_POINT ( 'NONE',  ( 37.53709685856478018, -3.054999999999998828, -5.291415217122919401 ) ) ;
#81294=CARTESIAN_POINT ( 'NONE',  ( 97.91209685856478018, 5.291415217122922066, -3.054999999999995275 ) ) ;
#81328=DIRECTION ( 'NONE',  ( -1.000000000000000000, -0.000000000000000000, -0.000000000000000000 ) ) ;
#81339=CARTESIAN_POINT ( 'NONE',  ( 125.9649422558287171, -6.613910356672960233, 3.556986441759899975 ) ) ;
#81347=CARTESIAN_POINT ( 'NONE',  ( 121.3124999999999858, 5.819803920172571310, 5.819803920172575751 ) ) ;
#81361=CARTESIAN_POINT ( 'NONE',  ( 113.6045968585647614, 1.637169565754164946, -6.109999999999999432 ) ) ;
#81372=CARTESIAN_POINT ( 'NONE',  ( 35.37086038379622011, 6.884901960086289741, -3.974999999999993427 ) ) ;
#81378=CARTESIAN_POINT ( 'NONE',  ( 39.93750000000000711, 5.819803920172573974, -5.819803920172572198 ) ) ;
#81392=CARTESIAN_POINT ( 'NONE',  ( 30.77126352523143638, 4.472830434245839371, 4.472830434245842035 ) ) ;
#81412=CARTESIAN_POINT ( 'NONE',  ( 48.91209685856478018, 5.291415217122921177, -3.054999999999994831 ) ) ;
#81441=CARTESIAN_POINT ( 'NONE',  ( 68.59959685856478018, -6.109999999999997655, -1.637169565754160283 ) ) ;
#81450=CARTESIAN_POINT ( 'NONE',  ( 35.70833333333332860, -3.974999999999999201, -6.884901960086287964 ) ) ;
#81476=CARTESIAN_POINT ( 'NONE',  ( 118.9333603837970088, 2.130196079837088252, -7.949999999994423305 ) ) ;
#81516=CARTESIAN_POINT ( 'NONE',  ( 49.05793019189810877, 6.110000000000001208, -1.637169565754156286 ) ) ;
#81542=CARTESIAN_POINT ( 'NONE',  ( 116.5000000000000000, 0.000000000000000000, -7.950000000000000178 ) ) ;
#81543=CARTESIAN_POINT ( 'NONE',  ( 74.45419371712955581, 6.884901960086283523, 3.975000000000002753 ) ) ;
#81547=CARTESIAN_POINT ( 'NONE',  ( 65.60416666666665719, 2.130196079827422206, 7.950000000000001954 ) ) ;
#81558=CARTESIAN_POINT ( 'NONE',  ( 59.93793019189809712, -6.110000000000001208, 1.637169565754158951 ) ) ;
#81603=CARTESIAN_POINT ( 'NONE',  ( 97.47459685856478018, 1.637169565754164280, -6.109999999999996767 ) ) ;
#81635=CARTESIAN_POINT ( 'NONE',  ( 44.91709685856476142, 3.054999999999998828, 5.291415217122922066 ) ) ;
#81684=AXIS2_PLACEMENT_3D ( 'NONE', #142511, #65698, #22810 ) ;
#81687=CARTESIAN_POINT ( 'NONE',  ( 78.37043019189812298, -3.055000000000001936, 5.291415217122918513 ) ) ;
#81688=CARTESIAN_POINT ( 'NONE',  ( 79.89583333333331439, -2.130196079827351596, 7.950000000000043698 ) ) ;
#81690=DIRECTION ( 'NONE',  ( 0.000000000000000000, 0.000000000000000000, 1.000000000000000000 ) ) ;
#81709=CARTESIAN_POINT ( 'NONE',  ( 121.9958603837962272, -3.974999999999998312, -6.884901960086286188 ) ) ;
#81712=CARTESIAN_POINT ( 'NONE',  ( 103.3291937171295700, -3.975000000000001865, 6.884901960086284411 ) ) ;
#81731=CARTESIAN_POINT ( 'NONE',  ( 86.18793019189811844, 6.110000000000002984, -1.637169565754156730 ) ) ;
#81749=DIRECTION ( 'NONE',  ( -1.000000000000000000, -0.000000000000000000, -0.000000000000000000 ) ) ;
#81754=CARTESIAN_POINT ( 'NONE',  ( 81.08376352523144703, -6.110000000000001208, -3.741295971395164515E-16 ) ) ;
#81766=CARTESIAN_POINT ( 'NONE',  ( 72.82876352523145158, 0.000000000000000000, -6.109999999999998543 ) ) ;
#81812=CARTESIAN_POINT ( 'NONE',  ( 70.14626352523144703, -4.472830434245840259, 4.472830434245838482 ) ) ;
#81816=CARTESIAN_POINT ( 'NONE',  ( 95.50000000000000000, 0.000000000000000000, -7.950000000000000178 ) ) ;
#81819=CARTESIAN_POINT ( 'NONE',  ( 112.8754301918981042, -5.291415217122920289, -3.055000000000001492 ) ) ;
#81827=CYLINDRICAL_SURFACE ( 'NONE', #121039, 7.950000000000000178 ) ;
#81849=ADVANCED_FACE ( 'NONE', ( #9197 ), #141936, .T. ) ;
#81872=CARTESIAN_POINT ( 'NONE',  ( 74.50000000000000000, 0.000000000000000000, -7.950000000000000178 ) ) ;
#81890=CARTESIAN_POINT ( 'NONE',  ( 127.6833603837962414, -2.130196079827426203, 7.949999999999997513 ) ) ;
#81906=CARTESIAN_POINT ( 'NONE',  ( 91.12500000000000000, -7.950000000000000178, -4.867971026610729436E-16 ) ) ;
#81918=CARTESIAN_POINT ( 'NONE',  ( 125.9070329220101030, 2.912925644401998859, -6.976214294840302088 ) ) ;
#81933=CARTESIAN_POINT ( 'NONE',  ( 108.0629301918980900, 1.637169565754157174, 6.110000000000002984 ) ) ;
#81934=AXIS2_PLACEMENT_3D ( 'NONE', #111549, #12226, #1338 ) ;
#81935=ORIENTED_EDGE ( 'NONE', *, *, #85740, .T. ) ;
#81943=CARTESIAN_POINT ( 'NONE',  ( 105.6412635252314658, 4.472830434245836706, 4.472830434245840259 ) ) ;
#81987=CARTESIAN_POINT ( 'NONE',  ( 36.66209685856478018, -5.291415217122919401, 3.054999999999997939 ) ) ;
#82006=VERTEX_POINT ( 'NONE', #105521 ) ;
#82026=CARTESIAN_POINT ( 'NONE',  ( 97.62043019189812298, 3.055000000000002380, -5.291415217122917625 ) ) ;
#82073=CARTESIAN_POINT ( 'NONE',  ( 117.8125000000000000, 5.819803920172571310, 5.819803920172575751 ) ) ;
#82086=CARTESIAN_POINT ( 'NONE',  ( 109.5212635252314612, -4.472830434245839371, -4.472830434245840259 ) ) ;
#82089=CARTESIAN_POINT ( 'NONE',  ( 0.000000000000000000, 0.000000000000000000, -6.349999999999999645 ) ) ;
#82095=CARTESIAN_POINT ( 'NONE',  ( 37.85002705046288440, -5.819803920172572198, -5.819803920172572198 ) ) ;
#82102=CARTESIAN_POINT ( 'NONE',  ( 35.56249999999999289, -5.819803920172572198, -5.819803920172573086 ) ) ;
#82112=CARTESIAN_POINT ( 'NONE',  ( 25.08376352523143638, -6.110000000000001208, -3.741295971395164515E-16 ) ) ;
#82121=CARTESIAN_POINT ( 'NONE',  ( 62.54166666666666430, -3.975000000000002753, 6.884901960086286188 ) ) ;
#82130=CARTESIAN_POINT ( 'NONE',  ( 49.20376352523145158, 6.109999999999998543, 1.122388791418548911E-15 ) ) ;
#82134=ORIENTED_EDGE ( 'NONE', *, *, #84424, .T. ) ;
#82140=CARTESIAN_POINT ( 'NONE',  ( 60.74586038379622721, 3.974999999999996980, 6.884901960086287964 ) ) ;
#82157=CARTESIAN_POINT ( 'NONE',  ( 63.20376352523145158, 6.109999999999998543, 1.122388791418548911E-15 ) ) ;
#82172=ORIENTED_EDGE ( 'NONE', *, *, #13248, .T. ) ;
#82231=CARTESIAN_POINT ( 'NONE',  ( 48.18293019189812298, -1.637169565754159173, -6.109999999999999432 ) ) ;
#82249=CARTESIAN_POINT ( 'NONE',  ( 117.5208333333333428, 7.949999999999998401, 2.130196079827431532 ) ) ;
#82250=CARTESIAN_POINT ( 'NONE',  ( 69.49586038379622721, -3.974999999999998312, -6.884901960086286188 ) ) ;
#82252=FACE_OUTER_BOUND ( 'NONE', #2287, .T. ) ;
#82255=CARTESIAN_POINT ( 'NONE',  ( 60.93750000000000000, 5.819803920172573974, -5.819803920172572198 ) ) ;
#82264=CARTESIAN_POINT ( 'NONE',  ( 56.58376352523143993, -6.110000000000001208, -3.741295971395164515E-16 ) ) ;
#82276=DIRECTION ( 'NONE',  ( -1.000000000000000000, -0.000000000000000000, -0.000000000000000000 ) ) ;
#82309=CARTESIAN_POINT ( 'NONE',  ( 97.18293019189810877, -1.637169565754158951, -6.109999999999998543 ) ) ;
#82335=CARTESIAN_POINT ( 'NONE',  ( 45.93793019189810423, -6.110000000000001208, 1.637169565754158951 ) ) ;
#82340=( BOUNDED_SURFACE ( )  B_SPLINE_SURFACE ( 1, 2, ( 
 ( #119804, #20495, #128573, #87213, #73491, #66188, #88657, #77774, #34997, #11762, #89350, #100235, #90048, #55311, #24103, #46620, #35732, #121953, #32856, #44453, #155, #111829, #56045, #90801, #135037, #54598, #79239, #123446, #57463, #87920, #21942, #122680, #11035, #23365, #111071, #13188, #132890, #33576, #886, #45174, #68357, #2302, #133582, #121254, #100932, #143017, #78484, #43705, #112529, #98778, #79949, #124121, #22624, #66891, #34262, #134298, #67637, #12491, #110360, #56772, #1589, #24799, #69048, #101645, #99484, #10343, #132163, #77079, #45873, #16030, #94341, #48711, #104499, #82771, #60322, #102395, #39271, #37852, #116087, #16783, #36404, #103089, #5160, #4407, #113228, #69782, #49456, #126960, #138577, #135719, #105219, #48015, #80633, #27650, #83493, #81361, #92185, #25506, #136412, #37107, #137873, #114652, #92917, #59607, #93645, #14649, #71919, #5876, #127707, #125567, #124833, #3724, #26246, #71192, #15323, #50143, #28391, #13904, #38547, #61065, #58204, #47339, #113956, #82086, #58926, #126266, #70510, #3042, #103766, #137149, #26942, #115340, #91508, #64577, #18922, #40005, #19639, #61746, #140693, #105907, #97160, #17491, #542, #11395, #62453, #84898, #40693, #8710, #129109, #74768, #84222, #96449, #118948, #55676, #99876, #20333, #73332, #42136, #31250, #44837, #29788, #110716, #6573, #89027, #74031, #129832, #107360, #41387, #63882, #118216, #108044, #95770, #51579, #133244, #50849, #29094, #72649, #116809, #140018, #63189, #139317, #52963, #8026, #52266, #141425, #95045, #128417, #117499, #85595, #86346, #30535, #130565, #18174, #75466, #119636, #106618, #7313, #1939, #113594, #59268, #70157, #78863, #13552, #36070, #90427, #68699, #103421, #124483, #46243, #134674, #91173, #80295, #14993, #112890, #25157, #3392, #69407, #22988, #4067, #102021, #36752, #80994, #100606, #23748, #14290, #57829, #33923, #133937, #58577, #47683, #48353, #56426, #25885, #112199, #1251, #91845, #92541, #35371, #12843, #89710, #57123, #101300, #102745, #79612, #2684, #123796, #136070, #123071, #125202, #114316, #78141, #24452, #45533, #68017, #46986, #135391, #122314, #67260, #111458, #12142, #34624, #62104, #40364, #70844, #4788, #105563, #137515, #6225, #93985, #139681, #115702, #126603, #38906, #83130, #51224, #128764, #127329, #104122, #83874, #125927, #61421, #26601, #17833, #81731, #62825, #73678, #27294, #5536, #104871, #73006, #49813, #138946, #49091, #17157, #39648, #117853, #18540, #84568, #38207, #106264, #95418, #107005, #138220, #29439, #114994, #7683, #28034, #50501, #72300, #94687, #128078, #116465, #28757, #16405, #60704, #51940, #15672, #93282, #136783, #37494, #117156, #6937, #59960, #82419, #71547, #19987, #140355, #42505, #22129, #141058, #131637, #33073, #142519, #76553, #41764, #8373, #88129, #66383, #118596, #19294, #85978, #110555, #11232, #109870, #75136, #130937, #9079, #54797, #52622, #64961, #77282, #63551, #9836, #53338, #30158, #65706, #120735, #97555, #31606, #107715, #96122, #32324, #43206, #10534, #21442, #87418, #86711, #141808, #64233, #96811, #41047, #119301, #98976, #143213, #108394, #130213, #30904, #75829, #119994, #20706, #43915, #109151, #54106, #132376, #98294, #121453, #74408, #85246, #129471, #33768, #113422, #46072, #2501, #55509, #112723, #114147, #69239, #101124, #1771, #57663, #88860, #100432, #101847, #80832, #36581, #34453, #35196, #46815, #133085, #90249, #22820, #112030, #56257, #91000, #14107, #12681, #1084, #77972, #135224, #11971, #80133, #35914, #135906, #45367, #24982, #134495, #102585, #124312, #58401, #25707, #89541, #3232, #79440, #47522, #23571, #67094, #91683, #125023, #123637, #133771, #122889, #24292, #111278, #69983, #68537, #99696, #122153, #78677, #371, #44664, #67842, #56953, #13384, #84404, #128600, #28586, #137348, #49647, #71372, #116998, #114833, #127155, #139512, #81558, #72118, #115534, #92372, #127906, #39467, #16225, #93825, #26435, #73516, #50332, #105402, #72845, #83699, #6060, #5364, #60516, #126440, #125762, #29274, #38040, #94519, #17667, #82264, #70685, #15509, #93117, #59790, #48914, #138776, #27851, #38737, #61939, #103958, #27134, #136605, #95242, #103261, #37312, #106089, #138052, #6764, #14831, #116288, #59106, #51046, #104697, #82960, #16986, #48186, #4602, #61256, #40197, #3911, #96636, #97361, #119828, #51767, #64060, #85087, #30733, #118416, #20516, #76367, #74962, #63379, #95957, #64777, #74221, #142347, #108957, #54621, #19117, #87237, #108225, #21264, #9649, #53923, #87945, #107547, #120536, #141624, #65521, #85795, #129290, #32138, #98116, #8890, #8208, #41575, #42324, #29982, #98805, #86537, #143040, #140194, #7508, #43726, #106824, #40881, #140875, #52447, #130027, #18365, #53158, #132185, #119135, #43033, #32885, #131461, #109697, #19819, #130766, #10365, #117677, #31433, #75655, #62640, #3072, #47363, #90830, #56073, #111854, #133609, #35754, #33597, #45896, #58231, #180, #134323, #34284, #11061, #46645, #101668, #78505, #12516, #88682, #135746, #112556, #24126, #135061, #2328, #68378, #67664, #122708, #45198, #44477, #91530, #100258, #13217, #79974, #914, #132917, #77797, #11787, #121980, #111095, #57489, #90072, #100956, #124144, #22649, #89376, #55332, #13930, #21966, #99508, #24830, #56796, #69075, #77105, #35024, #121281, #113251, #23389, #1613, #79266, #110387, #66915, #123468, #102425, #66211, #15348, #16053, #38570, #113986, #126290, #3751, #92945, #37137, #82805, #138607, #137181, #125598, #14676, #126986, #136438, #61091, #27675, #116837, #81392, #5898, #26969, #83520, #71944, #116114, #6596, #26272, #39294, #60346, #127734, #4431, #48039, #94363, #16816, #71219, #70536, #103792, #104529, #92212, #17513, #5192, #61769, #58957, #69809, #105934, #25536, #103112, #59636, #114680, #48743, #80663, #115368, #50876, #37878, #105248, #95072, #50170, #28417, #82112 ),
 ( #49484, #72679, #93672, #36430, #124858, #137896, #109531, #95795, #142184, #19663, #97948, #107383, #106650, #53747, #86371, #129857, #29814, #63215, #63902, #7338, #120360, #108065, #76198, #73357, #29117, #21086, #128446, #62472, #18952, #117524, #8052, #40033, #85617, #65350, #40719, #31274, #10203, #42159, #119658, #84925, #51603, #131286, #54468, #18200, #140042, #129137, #139342, #84246, #9469, #118241, #30559, #52287, #42877, #74052, #8734, #96474, #140718, #52990, #41411, #74797, #108778, #20355, #118972, #97183, #141451, #130595, #75486, #64603, #87071, #31972, #89909, #89218, #11606, #66751, #66057, #24654, #77642, #134152, #101500, #121810, #21809, #110219, #33440, #6, #132751, #34848, #111680, #122535, #23961, #10897, #22486, #32708, #35585, #43561, #76939, #13051, #133439, #45736, #98648, #12347, #13755, #112396, #743, #45039, #100801, #132013, #44301, #1451, #123991, #79813, #110924, #78338, #79088, #121111, #68911, #87781, #55163, #57324, #34127, #123292, #142874, #56634, #99342, #2154, #23204, #67489, #68219, #88513, #55893, #46462, #113086, #100091, #90658, #134889, #60166, #135586, #4263, #25364, #114514, #58784, #104337, #16625, #15190, #3591, #36266, #5003, #14499, #82618, #49303, #138426, #102948, #27493, #48561, #105071, #93491, #137725, #28237, #47881, #60909, #81943, #5731, #26101, #69628, #115917, #38399, #92759, #92045, #125415, #126127, #113813, #39111, #26802, #83335, #80494, #91375, #127542, #47194, #124691, #81207, #136272, #70360, #102245, #136997, #72498, #36958, #126809, #116661, #71758, #50000, #59466, #103624, #94182, #58048, #37703, #71046, #115195, #2899, #15876, #31103, #139874, #52120, #73879, #119489, #117349, #129669, #142013, #84074, #74610, #118049, #94888, #130416, #41974, #18758, #96302, #28948, #76017, #52809, #107895, #75322, #86185, #8563, #7882, #63032, #128964, #128271, #86904, #40549, #97007, #20179, #84754, #73187, #18022, #95619, #62303, #51426, #141259, #30367, #41234, #64422, #106462, #29634, #108602, #9281, #53560, #97766, #140547, #107208, #85441, #7145, #131120, #118798, #42704, #31804, #19490, #63737, #17345, #61606, #105756, #6415, #50700, #139153, #39853, #45572, #32525, #143410, #54300, #57163, #65169, #98481, #34668, #110750, #67301, #120193, #33961, #35411, #133967, #22312, #66584, #122352, #10039, #21644, #23031, #1972, #101336, #99163, #99911, #111498, #142706, #11438, #87607, #33275, #120939, #12178, #78904, #77477, #65896, #43397, #56465, #76763, #1287, #100641, #46286, #110052, #89745, #55713, #23788, #123113, #68054, #90470, #10729, #112232, #578, #12883, #88340, #131835, #134717, #20904, #44876, #54999, #44116, #89059, #132581, #109357, #133278, #121643, #78176, #112925, #18394, #68740, #2730, #102785, #13586, #3428, #123831, #25925, #7531, #124523, #115031, #62663, #125959, #59988, #25191, #135426, #73541, #51796, #102056, #47025, #69448, #95978, #140220, #95269, #58613, #114355, #136104, #40219, #36105, #48382, #106853, #91214, #136818, #36785, #57871, #51072, #104159, #81034, #15026, #80334, #79652, #15704, #113632, #14326, #47719, #91882, #6791, #92581, #103459, #139537, #125235, #70191, #59302, #24488, #4098, #37531, #84431, #81766, #26634, #70878, #128625, #29298, #117703, #86561, #130793, #43061, #74248, #85817, #87261, #66237, #21986, #19845, #20547, #131483, #118443, #31458, #8231, #97388, #41605, #32163, #143063, #141651, #130057, #19143, #76398, #75679, #98144, #21291, #110410, #119848, #120560, #10390, #65549, #30007, #11086, #108982, #43755, #87971, #107570, #30755, #109720, #64804, #40903, #140906, #54645, #98833, #55359, #63404, #32910, #119159, #52474, #132215, #99535, #8916, #64081, #96660, #108249, #53188, #77131, #42350, #9679, #53947, #121305, #74986, #85110, #129318, #142368, #67688, #22671, #34307, #133630, #101694, #1636, #80682, #36452, #44506, #24851, #69096, #47381, #77819, #11809, #112581, #937, #13240, #100980, #3095, #122736, #78532, #45917, #90101, #58253, #135766, #134347, #111121, #90853, #132941, #68401, #33620, #113277, #88707, #69826, #124882, #23413, #12540, #111876, #79993, #56817, #2352, #56096, #24146, #57510, #45223, #46664, #35046, #91549, #79288, #123492, #135085, #35774, #102442, #25559, #124171, #100286, #13952, #122004, #114005, #66940, #14694, #89399, #58974, #203, #92966, #115383, #71237, #39318, #16073, #105267, #114697, #127003, #5916, #84269, #128462, #50900, #103806, #72700, #61791, #29137, #60369, #139363, #37159, #73380, #104549, #16837, #137914, #27700, #94379, #5216, #50193, #126305, #82130, #40051, #81412, #59652, #117542, #95093, #26992, #49507, #26293, #138627, #93688, #38591, #83542, #18219, #103128, #4454, #82827, #127751, #71963, #116137, #3769, #28439, #61116, #116857, #17533, #105953, #48053, #6612, #92231, #136458, #125615, #70550, #15367, #48762, #137202, #37898, #129156, #52308, #9489, #97207, #62494, #18971, #97968, #31987, #87793, #84946, #54481, #140736, #29831, #76215, #132033, #30579, #41430, #118262, #85639, #129878, #87089, #63917, #141471, #8751, #142203, #107404, #120378, #98662, #32724, #74816, #74075, #96494, #118994, #20376, #108088, #142893, #43576, #106670, #131305, #21104, #109545, #140062, #63236, #8067, #42893, #65366, #76955, #19679, #121126, #53008, #42176, #10223, #7359, #86389, #130619, #31292, #75504, #119674, #51622, #64616, #108800, #53765, #95815, #40738, #35601, #58066, #47209, #89232, #44320, #55907, #11626, #123306, #23224, #102261, #2912, #66071, #46482, #90673, #68929, #99355, #33458, #134165, #22504, #34864, #122547, #24668, #759, #100108, #67505, #111693, #79827, #13768, #12365, #132768, #112408, #10916, #89922, #55181, #134904, #110233, #91390, #135596, #45059, #34145, #133456, #101515, #78355, #23973, #77656, #45754, #68234, #36279, #80509, #113102, #66767, #124003, #21828, #23, #56649, #88528, #121825 ) ),
 .UNSPECIFIED., .F., .F., .F. ) 
 B_SPLINE_SURFACE_WITH_KNOTS ( ( 2, 2 ),
 ( 3, 2, 2, 2, 2, 2, 2, 2, 2, 2, 2, 2, 2, 2, 2, 2, 2, 2, 2, 2, 2, 2, 2, 2, 2, 2, 2, 2, 2, 2, 2, 2, 2, 2, 2, 2, 2, 2, 2, 2, 2, 2, 2, 2, 2, 2, 2, 2, 2, 2, 2, 2, 2, 2, 2, 2, 2, 2, 2, 2, 2, 2, 2, 2, 2, 2, 2, 2, 2, 2, 2, 2, 2, 2, 2, 2, 2, 2, 2, 2, 2, 2, 2, 2, 2, 2, 2, 2, 2, 2, 2, 2, 2, 2, 2, 2, 2, 2, 2, 2, 2, 2, 2, 2, 2, 2, 2, 2, 2, 2, 2, 2, 2, 2, 2, 2, 2, 2, 2, 2, 2, 2, 2, 2, 2, 2, 2, 2, 2, 2, 2, 2, 2, 2, 2, 2, 2, 2, 2, 2, 2, 2, 2, 2, 2, 2, 2, 2, 2, 2, 2, 2, 2, 2, 2, 2, 2, 2, 2, 2, 2, 2, 2, 2, 2, 2, 2, 2, 2, 2, 2, 2, 2, 2, 2, 2, 2, 2, 2, 2, 2, 2, 2, 2, 2, 2, 2, 2, 2, 2, 2, 2, 2, 2, 2, 2, 2, 2, 2, 2, 2, 2, 2, 2, 2, 2, 2, 2, 2, 2, 2, 2, 2, 2, 2, 2, 2, 2, 2, 2, 2, 2, 2, 2, 2, 2, 2, 2, 2, 2, 2, 2, 2, 2, 2, 2, 2, 2, 2, 2, 2, 2, 2, 2, 2, 2, 2, 2, 2, 2, 2, 2, 2, 2, 2, 2, 2, 2, 2, 2, 2, 2, 2, 2, 2, 2, 2, 2, 2, 2, 2, 2, 2, 2, 2, 2, 2, 2, 2, 2, 2, 2, 2, 2, 2, 2, 2, 2, 2, 2, 2, 2, 2, 2, 2, 2, 2, 2, 2, 2, 2, 2, 2, 2, 2, 2, 2, 2, 2, 2, 2, 2, 2, 2, 2, 2, 2, 2, 2, 2, 2, 2, 2, 2, 2, 2, 2, 2, 2, 2, 2, 2, 2, 2, 2, 2, 2, 2, 2, 2, 2, 2, 2, 2, 2, 2, 2, 2, 2, 2, 2, 3 ),
 ( 0.000000000000000000, 1.000000000000000000 ),
 ( 0.000000000000000000, 0.002777777777777777884, 0.005555555555555555768, 0.008333333333333333218, 0.01111111111111111154, 0.01388888888888888812, 0.01666666666666666644, 0.01944444444444444475, 0.02222222222222222307, 0.02500000000000000139, 0.02777777777777777624, 0.03055555555555555455, 0.03333333333333333287, 0.03611111111111110772, 0.03888888888888888951, 0.04166666666666666435, 0.04444444444444444614, 0.04722222222222222099, 0.05000000000000000278, 0.05277777777777777762, 0.05555555555555555247, 0.05833333333333333426, 0.06111111111111110911, 0.06388888888888888395, 0.06666666666666666574, 0.06944444444444444753, 0.07222222222222221544, 0.07499999999999999722, 0.07777777777777777901, 0.08055555555555556080, 0.08333333333333332871, 0.08611111111111111049, 0.08888888888888889228, 0.09166666666666666019, 0.09444444444444444198, 0.09722222222222222376, 0.1000000000000000056, 0.1027777777777777735, 0.1055555555555555552, 0.1083333333333333370, 0.1111111111111111049, 0.1138888888888888867, 0.1166666666666666685, 0.1194444444444444503, 0.1222222222222222182, 0.1250000000000000000, 0.1277777777777777679, 0.1305555555555555636, 0.1333333333333333315, 0.1361111111111110994, 0.1388888888888888951, 0.1416666666666666630, 0.1444444444444444309, 0.1472222222222222265, 0.1499999999999999944, 0.1527777777777777901, 0.1555555555555555580, 0.1583333333333333259, 0.1611111111111111216, 0.1638888888888888895, 0.1666666666666666574, 0.1694444444444444531, 0.1722222222222222210, 0.1749999999999999889, 0.1777777777777777846, 0.1805555555555555525, 0.1833333333333333204, 0.1861111111111111160, 0.1888888888888888840, 0.1916666666666666796, 0.1944444444444444475, 0.1972222222222222154, 0.2000000000000000111, 0.2027777777777777790, 0.2055555555555555469, 0.2083333333333333426, 0.2111111111111111105, 0.2138888888888888784, 0.2166666666666666741, 0.2194444444444444420, 0.2222222222222222099, 0.2250000000000000056, 0.2277777777777777735, 0.2305555555555555691, 0.2333333333333333370, 0.2361111111111111049, 0.2388888888888889006, 0.2416666666666666685, 0.2444444444444444364, 0.2472222222222222321, 0.2500000000000000000, 0.2527777777777777679, 0.2555555555555555358, 0.2583333333333333592, 0.2611111111111111271, 0.2638888888888888951, 0.2666666666666666630, 0.2694444444444444309, 0.2722222222222221988, 0.2750000000000000222, 0.2777777777777777901, 0.2805555555555555580, 0.2833333333333333259, 0.2861111111111110938, 0.2888888888888888618, 0.2916666666666666852, 0.2944444444444444531, 0.2972222222222222210, 0.2999999999999999889, 0.3027777777777777568, 0.3055555555555555802, 0.3083333333333333481, 0.3111111111111111160, 0.3138888888888888840, 0.3166666666666666519, 0.3194444444444444198, 0.3222222222222222432, 0.3250000000000000111, 0.3277777777777777790, 0.3305555555555555469, 0.3333333333333333148, 0.3361111111111111382, 0.3388888888888889062, 0.3416666666666666741, 0.3444444444444444420, 0.3472222222222222099, 0.3499999999999999778, 0.3527777777777778012, 0.3555555555555555691, 0.3583333333333333370, 0.3611111111111111049, 0.3638888888888888729, 0.3666666666666666408, 0.3694444444444444642, 0.3722222222222222321, 0.3750000000000000000, 0.3777777777777777679, 0.3805555555555555358, 0.3833333333333333592, 0.3861111111111111271, 0.3888888888888888951, 0.3916666666666666630, 0.3944444444444444309, 0.3972222222222221988, 0.4000000000000000222, 0.4027777777777777901, 0.4055555555555555580, 0.4083333333333333259, 0.4111111111111110938, 0.4138888888888888618, 0.4166666666666666852, 0.4194444444444444531, 0.4222222222222222210, 0.4249999999999999889, 0.4277777777777777568, 0.4305555555555555802, 0.4333333333333333481, 0.4361111111111111160, 0.4388888888888888840, 0.4416666666666666519, 0.4444444444444444198, 0.4472222222222222432, 0.4500000000000000111, 0.4527777777777777790, 0.4555555555555555469, 0.4583333333333333148, 0.4611111111111111382, 0.4638888888888889062, 0.4666666666666666741, 0.4694444444444444420, 0.4722222222222222099, 0.4749999999999999778, 0.4777777777777778012, 0.4805555555555555691, 0.4833333333333333370, 0.4861111111111111049, 0.4888888888888888729, 0.4916666666666666408, 0.4944444444444444642, 0.4972222222222222321, 0.5000000000000000000, 0.5027777777777777679, 0.5055555555555555358, 0.5083333333333333037, 0.5111111111111110716, 0.5138888888888888395, 0.5166666666666667185, 0.5194444444444444864, 0.5222222222222222543, 0.5250000000000000222, 0.5277777777777777901, 0.5305555555555555580, 0.5333333333333333259, 0.5361111111111110938, 0.5388888888888888618, 0.5416666666666666297, 0.5444444444444443976, 0.5472222222222222765, 0.5500000000000000444, 0.5527777777777778123, 0.5555555555555555802, 0.5583333333333333481, 0.5611111111111111160, 0.5638888888888888840, 0.5666666666666666519, 0.5694444444444444198, 0.5722222222222221877, 0.5749999999999999556, 0.5777777777777777235, 0.5805555555555556024, 0.5833333333333333703, 0.5861111111111111382, 0.5888888888888889062, 0.5916666666666666741, 0.5944444444444444420, 0.5972222222222222099, 0.5999999999999999778, 0.6027777777777777457, 0.6055555555555555136, 0.6083333333333332815, 0.6111111111111111605, 0.6138888888888889284, 0.6166666666666666963, 0.6194444444444444642, 0.6222222222222222321, 0.6250000000000000000, 0.6277777777777777679, 0.6305555555555555358, 0.6333333333333333037, 0.6361111111111110716, 0.6388888888888888395, 0.6416666666666667185, 0.6444444444444444864, 0.6472222222222222543, 0.6500000000000000222, 0.6527777777777777901, 0.6555555555555555580, 0.6583333333333333259, 0.6611111111111110938, 0.6638888888888888618, 0.6666666666666666297, 0.6694444444444443976, 0.6722222222222222765, 0.6750000000000000444, 0.6777777777777778123, 0.6805555555555555802, 0.6833333333333333481, 0.6861111111111111160, 0.6888888888888888840, 0.6916666666666666519, 0.6944444444444444198, 0.6972222222222221877, 0.6999999999999999556, 0.7027777777777777235, 0.7055555555555556024, 0.7083333333333333703, 0.7111111111111111382, 0.7138888888888889062, 0.7166666666666666741, 0.7194444444444444420, 0.7222222222222222099, 0.7249999999999999778, 0.7277777777777777457, 0.7305555555555555136, 0.7333333333333332815, 0.7361111111111111605, 0.7388888888888889284, 0.7416666666666666963, 0.7444444444444444642, 0.7472222222222222321, 0.7500000000000000000, 0.7527777777777777679, 0.7555555555555555358, 0.7583333333333333037, 0.7611111111111110716, 0.7638888888888888395, 0.7666666666666667185, 0.7694444444444444864, 0.7722222222222222543, 0.7750000000000000222, 0.7777777777777777901, 0.7805555555555555580, 0.7833333333333333259, 0.7861111111111110938, 0.7888888888888888618, 0.7916666666666666297, 0.7944444444444443976, 0.7972222222222222765, 0.8000000000000000444, 0.8027777777777778123, 0.8055555555555555802, 0.8083333333333333481, 0.8111111111111111160, 0.8138888888888888840, 0.8166666666666666519, 0.8194444444444444198, 0.8222222222222221877, 0.8249999999999999556, 0.8277777777777777235, 0.8305555555555556024, 0.8333333333333333703, 0.8361111111111111382, 0.8388888888888889062, 0.8416666666666666741, 0.8444444444444444420, 0.8472222222222222099, 0.8499999999999999778, 0.8527777777777777457, 0.8555555555555555136, 0.8583333333333332815, 0.8611111111111111605, 0.8638888888888889284, 0.8666666666666666963, 0.8694444444444444642, 0.8722222222222222321, 0.8750000000000000000, 0.8777777777777777679, 0.8805555555555555358, 0.8833333333333333037, 0.8861111111111110716, 0.8888888888888888395, 0.8916666666666667185, 0.8944444444444444864, 0.8972222222222222543, 0.9000000000000000222, 0.9027777777777777901, 0.9055555555555555580, 0.9083333333333333259, 0.9111111111111110938, 0.9138888888888888618, 0.9166666666666666297, 0.9194444444444443976, 0.9222222222222222765, 0.9250000000000000444, 0.9277777777777778123, 0.9305555555555555802, 0.9333333333333333481, 0.9361111111111111160, 0.9388888888888888840, 0.9416666666666666519, 0.9444444444444444198, 0.9472222222222221877, 0.9499999999999999556, 0.9527777777777777235, 0.9555555555555556024, 0.9583333333333333703, 0.9611111111111111382, 0.9638888888888889062, 0.9666666666666666741, 0.9694444444444444420, 0.9722222222222222099, 0.9749999999999999778 ),
 .UNSPECIFIED. ) 
 GEOMETRIC_REPRESENTATION_ITEM ( )  RATIONAL_B_SPLINE_SURFACE ( (
 ( 1.000000000000000000, 0.9659258262890683122, 1.000000000000000000, 0.9659258262890683122, 1.000000000000000000, 0.9659258262890683122, 1.000000000000000000, 0.9659258262890683122, 1.000000000000000000, 0.9659258262890683122, 1.000000000000000000, 0.9659258262890683122, 1.000000000000000000, 0.9659258262890683122, 1.000000000000000000, 0.9659258262890683122, 1.000000000000000000, 0.9659258262890683122, 1.000000000000000000, 0.9659258262890683122, 1.000000000000000000, 0.9659258262890683122, 1.000000000000000000, 0.9659258262890683122, 1.000000000000000000, 0.9659258262890683122, 1.000000000000000000, 0.9659258262890683122, 1.000000000000000000, 0.9659258262890683122, 1.000000000000000000, 0.9659258262890683122, 1.000000000000000000, 0.9659258262890683122, 1.000000000000000000, 0.9659258262890683122, 1.000000000000000000, 0.9659258262890683122, 1.000000000000000000, 0.9659258262890683122, 1.000000000000000000, 0.9659258262890683122, 1.000000000000000000, 0.9659258262890683122, 1.000000000000000000, 0.9659258262890683122, 1.000000000000000000, 0.9659258262890683122, 1.000000000000000000, 0.9659258262890683122, 1.000000000000000000, 0.9659258262890683122, 1.000000000000000000, 0.9659258262890683122, 1.000000000000000000, 0.9659258262890683122, 1.000000000000000000, 0.9659258262890683122, 1.000000000000000000, 0.9659258262890683122, 1.000000000000000000, 0.9659258262890683122, 1.000000000000000000, 0.9659258262890683122, 1.000000000000000000, 0.9659258262890683122, 1.000000000000000000, 0.9659258262890683122, 1.000000000000000000, 0.9659258262890683122, 1.000000000000000000, 0.9659258262890683122, 1.000000000000000000, 0.9659258262890683122, 1.000000000000000000, 0.9659258262890683122, 1.000000000000000000, 0.9659258262890683122, 1.000000000000000000, 0.9659258262890683122, 1.000000000000000000, 0.9659258262890683122, 1.000000000000000000, 0.9659258262890683122, 1.000000000000000000, 0.9659258262890683122, 1.000000000000000000, 0.9659258262890683122, 1.000000000000000000, 0.9659258262890683122, 1.000000000000000000, 0.9659258262890683122, 1.000000000000000000, 0.9659258262890683122, 1.000000000000000000, 0.9659258262890683122, 1.000000000000000000, 0.9659258262890683122, 1.000000000000000000, 0.9659258262890683122, 1.000000000000000000, 0.9659258262890683122, 1.000000000000000000, 0.9659258262890683122, 1.000000000000000000, 0.9659258262890683122, 1.000000000000000000, 0.9659258262890683122, 1.000000000000000000, 0.9659258262890683122, 1.000000000000000000, 0.9659258262890683122, 1.000000000000000000, 0.9659258262890683122, 1.000000000000000000, 0.9659258262890683122, 1.000000000000000000, 0.9659258262890683122, 1.000000000000000000, 0.9659258262890683122, 1.000000000000000000, 0.9659258262890683122, 1.000000000000000000, 0.9659258262890683122, 1.000000000000000000, 0.9659258262890683122, 1.000000000000000000, 0.9659258262890683122, 1.000000000000000000, 0.9659258262890683122, 1.000000000000000000, 0.9659258262890683122, 1.000000000000000000, 0.9659258262890683122, 1.000000000000000000, 0.9659258262890683122, 1.000000000000000000, 0.9659258262890683122, 1.000000000000000000, 0.9659258262890683122, 1.000000000000000000, 0.9659258262890683122, 1.000000000000000000, 0.9659258262890683122, 1.000000000000000000, 0.9659258262890683122, 1.000000000000000000, 0.9659258262890683122, 1.000000000000000000, 0.9659258262890683122, 1.000000000000000000, 0.9659258262890683122, 1.000000000000000000, 0.9659258262890683122, 1.000000000000000000, 0.9659258262890683122, 1.000000000000000000, 0.9659258262890683122, 1.000000000000000000, 0.9659258262890683122, 1.000000000000000000, 0.9659258262890683122, 1.000000000000000000, 0.9659258262890683122, 1.000000000000000000, 0.9659258262890683122, 1.000000000000000000, 0.9659258262890683122, 1.000000000000000000, 0.9659258262890683122, 1.000000000000000000, 0.9659258262890683122, 1.000000000000000000, 0.9659258262890683122, 1.000000000000000000, 0.9659258262890683122, 1.000000000000000000, 0.9659258262890683122, 1.000000000000000000, 0.9659258262890683122, 1.000000000000000000, 0.9659258262890683122, 1.000000000000000000, 0.9659258262890683122, 1.000000000000000000, 0.9659258262890683122, 1.000000000000000000, 0.9659258262890683122, 1.000000000000000000, 0.9659258262890683122, 1.000000000000000000, 0.9659258262890683122, 1.000000000000000000, 0.9659258262890683122, 1.000000000000000000, 0.9659258262890683122, 1.000000000000000000, 0.9659258262890683122, 1.000000000000000000, 0.9659258262890683122, 1.000000000000000000, 0.9659258262890683122, 1.000000000000000000, 0.9659258262890683122, 1.000000000000000000, 0.9659258262890683122, 1.000000000000000000, 0.9659258262890683122, 1.000000000000000000, 0.9659258262890683122, 1.000000000000000000, 0.9659258262890683122, 1.000000000000000000, 0.9659258262890683122, 1.000000000000000000, 0.9659258262890683122, 1.000000000000000000, 0.9659258262890683122, 1.000000000000000000, 0.9659258262890683122, 1.000000000000000000, 0.9659258262890683122, 1.000000000000000000, 0.9659258262890683122, 1.000000000000000000, 0.9659258262890683122, 1.000000000000000000, 0.9659258262890683122, 1.000000000000000000, 0.9659258262890683122, 1.000000000000000000, 0.9659258262890683122, 1.000000000000000000, 0.9659258262890683122, 1.000000000000000000, 0.9659258262890683122, 1.000000000000000000, 0.9659258262890683122, 1.000000000000000000, 0.9659258262890683122, 1.000000000000000000, 0.9659258262890683122, 1.000000000000000000, 0.9659258262890683122, 1.000000000000000000, 0.9659258262890683122, 1.000000000000000000, 0.9659258262890683122, 1.000000000000000000, 0.9659258262890683122, 1.000000000000000000, 0.9659258262890683122, 1.000000000000000000, 0.9659258262890683122, 1.000000000000000000, 0.9659258262890683122, 1.000000000000000000, 0.9659258262890683122, 1.000000000000000000, 0.9659258262890683122, 1.000000000000000000, 0.9659258262890683122, 1.000000000000000000, 0.9659258262890683122, 1.000000000000000000, 0.9659258262890683122, 1.000000000000000000, 0.9659258262890683122, 1.000000000000000000, 0.9659258262890683122, 1.000000000000000000, 0.9659258262890683122, 1.000000000000000000, 0.9659258262890683122, 1.000000000000000000, 0.9659258262890683122, 1.000000000000000000, 0.9659258262890683122, 1.000000000000000000, 0.9659258262890683122, 1.000000000000000000, 0.9659258262890683122, 1.000000000000000000, 0.9659258262890683122, 1.000000000000000000, 0.9659258262890683122, 1.000000000000000000, 0.9659258262890683122, 1.000000000000000000, 0.9659258262890683122, 1.000000000000000000, 0.9659258262890683122, 1.000000000000000000, 0.9659258262890683122, 1.000000000000000000, 0.9659258262890683122, 1.000000000000000000, 0.9659258262890683122, 1.000000000000000000, 0.9659258262890683122, 1.000000000000000000, 0.9659258262890683122, 1.000000000000000000, 0.9659258262890683122, 1.000000000000000000, 0.9659258262890683122, 1.000000000000000000, 0.9659258262890683122, 1.000000000000000000, 0.9659258262890683122, 1.000000000000000000, 0.9659258262890683122, 1.000000000000000000, 0.9659258262890683122, 1.000000000000000000, 0.9659258262890683122, 1.000000000000000000, 0.9659258262890683122, 1.000000000000000000, 0.9659258262890683122, 1.000000000000000000, 0.9659258262890683122, 1.000000000000000000, 0.9659258262890683122, 1.000000000000000000, 0.9659258262890683122, 1.000000000000000000, 0.9659258262890683122, 1.000000000000000000, 0.9659258262890683122, 1.000000000000000000, 0.9659258262890683122, 1.000000000000000000, 0.9659258262890683122, 1.000000000000000000, 0.9659258262890683122, 1.000000000000000000, 0.9659258262890683122, 1.000000000000000000, 0.9659258262890683122, 1.000000000000000000, 0.9659258262890683122, 1.000000000000000000, 0.9659258262890683122, 1.000000000000000000, 0.9659258262890683122, 1.000000000000000000, 0.9659258262890683122, 1.000000000000000000, 0.9659258262890683122, 1.000000000000000000, 0.9659258262890683122, 1.000000000000000000, 0.9659258262890683122, 1.000000000000000000, 0.9659258262890683122, 1.000000000000000000, 0.9659258262890683122, 1.000000000000000000, 0.9659258262890683122, 1.000000000000000000, 0.9659258262890683122, 1.000000000000000000, 0.9659258262890683122, 1.000000000000000000, 0.9659258262890683122, 1.000000000000000000, 0.9659258262890683122, 1.000000000000000000, 0.9659258262890683122, 1.000000000000000000, 0.9659258262890683122, 1.000000000000000000, 0.9659258262890683122, 1.000000000000000000, 0.9659258262890683122, 1.000000000000000000, 0.9659258262890683122, 1.000000000000000000, 0.9659258262890683122, 1.000000000000000000, 0.9659258262890683122, 1.000000000000000000, 0.9659258262890683122, 1.000000000000000000, 0.9659258262890683122, 1.000000000000000000, 0.9659258262890683122, 1.000000000000000000, 0.9659258262890683122, 1.000000000000000000, 0.9659258262890683122, 1.000000000000000000, 0.9659258262890683122, 1.000000000000000000, 0.9659258262890683122, 1.000000000000000000, 0.9659258262890683122, 1.000000000000000000, 0.9659258262890683122, 1.000000000000000000, 0.9659258262890683122, 1.000000000000000000, 0.9659258262890683122, 1.000000000000000000, 0.9659258262890683122, 1.000000000000000000, 0.9659258262890683122, 1.000000000000000000, 0.9659258262890683122, 1.000000000000000000, 0.9659258262890683122, 1.000000000000000000, 0.9659258262890683122, 1.000000000000000000, 0.9659258262890683122, 1.000000000000000000, 0.9659258262890683122, 1.000000000000000000, 0.9659258262890683122, 1.000000000000000000, 0.9659258262890683122, 1.000000000000000000, 0.9659258262890683122, 1.000000000000000000, 0.9659258262890683122, 1.000000000000000000, 0.9659258262890683122, 1.000000000000000000, 0.9659258262890683122, 1.000000000000000000, 0.9659258262890683122, 1.000000000000000000, 0.9659258262890683122, 1.000000000000000000, 0.9659258262890683122, 1.000000000000000000, 0.9659258262890683122, 1.000000000000000000, 0.9659258262890683122, 1.000000000000000000, 0.9659258262890683122, 1.000000000000000000, 0.9659258262890683122, 1.000000000000000000, 0.9659258262890683122, 1.000000000000000000, 0.9659258262890683122, 1.000000000000000000, 0.9659258262890683122, 1.000000000000000000, 0.9659258262890683122, 1.000000000000000000, 0.9659258262890683122, 1.000000000000000000, 0.9659258262890683122, 1.000000000000000000, 0.9659258262890683122, 1.000000000000000000, 0.9659258262890683122, 1.000000000000000000, 0.9659258262890683122, 1.000000000000000000, 0.9659258262890683122, 1.000000000000000000, 0.9659258262890683122, 1.000000000000000000, 0.9659258262890683122, 1.000000000000000000, 0.9659258262890683122, 1.000000000000000000, 0.9659258262890683122, 1.000000000000000000, 0.9659258262890683122, 1.000000000000000000, 0.9659258262890683122, 1.000000000000000000, 0.9659258262890683122, 1.000000000000000000, 0.9659258262890683122, 1.000000000000000000, 0.9659258262890683122, 1.000000000000000000, 0.9659258262890683122, 1.000000000000000000, 0.9659258262890683122, 1.000000000000000000, 0.9659258262890683122, 1.000000000000000000, 0.9659258262890683122, 1.000000000000000000, 0.9659258262890683122, 1.000000000000000000, 0.9659258262890683122, 1.000000000000000000, 0.9659258262890683122, 1.000000000000000000, 0.9659258262890683122, 1.000000000000000000, 0.9659258262890683122, 1.000000000000000000, 0.9659258262890683122, 1.000000000000000000, 0.9659258262890683122, 1.000000000000000000, 0.9659258262890683122, 1.000000000000000000, 0.9659258262890683122, 1.000000000000000000, 0.9659258262890683122, 1.000000000000000000, 0.9659258262890683122, 1.000000000000000000, 0.9659258262890683122, 1.000000000000000000, 0.9659258262890683122, 1.000000000000000000, 0.9659258262890683122, 1.000000000000000000, 0.9659258262890683122, 1.000000000000000000, 0.9659258262890683122, 1.000000000000000000, 0.9659258262890683122, 1.000000000000000000, 0.9659258262890683122, 1.000000000000000000, 0.9659258262890683122, 1.000000000000000000, 0.9659258262890683122, 1.000000000000000000, 0.9659258262890683122, 1.000000000000000000, 0.9659258262890683122, 1.000000000000000000, 0.9659258262890683122, 1.000000000000000000, 0.9659258262890683122, 1.000000000000000000, 0.9659258262890683122, 1.000000000000000000, 0.9659258262890683122, 1.000000000000000000, 0.9659258262890683122, 1.000000000000000000, 0.9659258262890683122, 1.000000000000000000, 0.9659258262890683122, 1.000000000000000000, 0.9659258262890683122, 1.000000000000000000, 0.9659258262890683122, 1.000000000000000000, 0.9659258262890683122, 1.000000000000000000, 0.9659258262890683122, 1.000000000000000000, 0.9659258262890683122, 1.000000000000000000, 0.9659258262890683122, 1.000000000000000000, 0.9659258262890683122, 1.000000000000000000, 0.9659258262890683122, 1.000000000000000000, 0.9659258262890683122, 1.000000000000000000, 0.9659258262890683122, 1.000000000000000000, 0.9659258262890683122, 1.000000000000000000, 0.9659258262890683122, 1.000000000000000000, 0.9659258262890683122, 1.000000000000000000, 0.9659258262890683122, 1.000000000000000000, 0.9659258262890683122, 1.000000000000000000, 0.9659258262890683122, 1.000000000000000000, 0.9659258262890683122, 1.000000000000000000, 0.9659258262890683122, 1.000000000000000000, 0.9659258262890683122, 1.000000000000000000, 0.9659258262890683122, 1.000000000000000000, 0.9659258262890683122, 1.000000000000000000, 0.9659258262890683122, 1.000000000000000000, 0.9659258262890683122, 1.000000000000000000, 0.9659258262890683122, 1.000000000000000000, 0.9659258262890683122, 1.000000000000000000, 0.9659258262890683122, 1.000000000000000000, 0.9659258262890683122, 1.000000000000000000, 0.9659258262890683122, 1.000000000000000000, 0.9659258262890683122, 1.000000000000000000, 0.9659258262890683122, 1.000000000000000000, 0.9659258262890683122, 1.000000000000000000, 0.9659258262890683122, 1.000000000000000000, 0.9659258262890683122, 1.000000000000000000, 0.9659258262890683122, 1.000000000000000000, 0.9659258262890683122, 1.000000000000000000, 0.9659258262890683122, 1.000000000000000000, 0.9659258262890683122, 1.000000000000000000, 0.9659258262890683122, 1.000000000000000000, 0.9659258262890683122, 1.000000000000000000, 0.9659258262890683122, 1.000000000000000000, 0.9659258262890683122, 1.000000000000000000, 0.9659258262890683122, 1.000000000000000000, 0.9659258262890683122, 1.000000000000000000, 0.9659258262890683122, 1.000000000000000000, 0.9659258262890683122, 1.000000000000000000, 0.9659258262890683122, 1.000000000000000000, 0.9659258262890683122, 1.000000000000000000, 0.9659258262890683122, 1.000000000000000000, 0.9659258262890683122, 1.000000000000000000, 0.9659258262890683122, 1.000000000000000000, 0.9659258262890683122, 1.000000000000000000, 0.9659258262890683122, 1.000000000000000000, 0.9659258262890683122, 1.000000000000000000, 0.9659258262890683122, 1.000000000000000000, 0.9659258262890683122, 1.000000000000000000, 0.9659258262890683122, 1.000000000000000000, 0.9659258262890683122, 1.000000000000000000, 0.9659258262890683122, 1.000000000000000000, 0.9659258262890683122, 1.000000000000000000, 0.9659258262890683122, 1.000000000000000000, 0.9659258262890683122, 1.000000000000000000, 0.9659258262890683122, 1.000000000000000000, 0.9659258262890683122, 1.000000000000000000, 0.9659258262890683122, 1.000000000000000000, 0.9659258262890683122, 1.000000000000000000, 0.9659258262890683122, 1.000000000000000000, 0.9659258262890683122, 1.000000000000000000, 0.9659258262890683122, 1.000000000000000000, 0.9659258262890683122, 1.000000000000000000, 0.9659258262890683122, 1.000000000000000000, 0.9659258262890683122, 1.000000000000000000, 0.9659258262890683122, 1.000000000000000000, 0.9659258262890683122, 1.000000000000000000, 0.9659258262890683122, 1.000000000000000000, 0.9659258262890683122, 1.000000000000000000, 0.9659258262890683122, 1.000000000000000000, 0.9659258262890683122, 1.000000000000000000),
 ( 1.000000000000000000, 0.9659258262890683122, 1.000000000000000000, 0.9659258262890683122, 1.000000000000000000, 0.9659258262890683122, 1.000000000000000000, 0.9659258262890683122, 1.000000000000000000, 0.9659258262890683122, 1.000000000000000000, 0.9659258262890683122, 1.000000000000000000, 0.9659258262890683122, 1.000000000000000000, 0.9659258262890683122, 1.000000000000000000, 0.9659258262890683122, 1.000000000000000000, 0.9659258262890683122, 1.000000000000000000, 0.9659258262890683122, 1.000000000000000000, 0.9659258262890683122, 1.000000000000000000, 0.9659258262890683122, 1.000000000000000000, 0.9659258262890683122, 1.000000000000000000, 0.9659258262890683122, 1.000000000000000000, 0.9659258262890683122, 1.000000000000000000, 0.9659258262890683122, 1.000000000000000000, 0.9659258262890683122, 1.000000000000000000, 0.9659258262890683122, 1.000000000000000000, 0.9659258262890683122, 1.000000000000000000, 0.9659258262890683122, 1.000000000000000000, 0.9659258262890683122, 1.000000000000000000, 0.9659258262890683122, 1.000000000000000000, 0.9659258262890683122, 1.000000000000000000, 0.9659258262890683122, 1.000000000000000000, 0.9659258262890683122, 1.000000000000000000, 0.9659258262890683122, 1.000000000000000000, 0.9659258262890683122, 1.000000000000000000, 0.9659258262890683122, 1.000000000000000000, 0.9659258262890683122, 1.000000000000000000, 0.9659258262890683122, 1.000000000000000000, 0.9659258262890683122, 1.000000000000000000, 0.9659258262890683122, 1.000000000000000000, 0.9659258262890683122, 1.000000000000000000, 0.9659258262890683122, 1.000000000000000000, 0.9659258262890683122, 1.000000000000000000, 0.9659258262890683122, 1.000000000000000000, 0.9659258262890683122, 1.000000000000000000, 0.9659258262890683122, 1.000000000000000000, 0.9659258262890683122, 1.000000000000000000, 0.9659258262890683122, 1.000000000000000000, 0.9659258262890683122, 1.000000000000000000, 0.9659258262890683122, 1.000000000000000000, 0.9659258262890683122, 1.000000000000000000, 0.9659258262890683122, 1.000000000000000000, 0.9659258262890683122, 1.000000000000000000, 0.9659258262890683122, 1.000000000000000000, 0.9659258262890683122, 1.000000000000000000, 0.9659258262890683122, 1.000000000000000000, 0.9659258262890683122, 1.000000000000000000, 0.9659258262890683122, 1.000000000000000000, 0.9659258262890683122, 1.000000000000000000, 0.9659258262890683122, 1.000000000000000000, 0.9659258262890683122, 1.000000000000000000, 0.9659258262890683122, 1.000000000000000000, 0.9659258262890683122, 1.000000000000000000, 0.9659258262890683122, 1.000000000000000000, 0.9659258262890683122, 1.000000000000000000, 0.9659258262890683122, 1.000000000000000000, 0.9659258262890683122, 1.000000000000000000, 0.9659258262890683122, 1.000000000000000000, 0.9659258262890683122, 1.000000000000000000, 0.9659258262890683122, 1.000000000000000000, 0.9659258262890683122, 1.000000000000000000, 0.9659258262890683122, 1.000000000000000000, 0.9659258262890683122, 1.000000000000000000, 0.9659258262890683122, 1.000000000000000000, 0.9659258262890683122, 1.000000000000000000, 0.9659258262890683122, 1.000000000000000000, 0.9659258262890683122, 1.000000000000000000, 0.9659258262890683122, 1.000000000000000000, 0.9659258262890683122, 1.000000000000000000, 0.9659258262890683122, 1.000000000000000000, 0.9659258262890683122, 1.000000000000000000, 0.9659258262890683122, 1.000000000000000000, 0.9659258262890683122, 1.000000000000000000, 0.9659258262890683122, 1.000000000000000000, 0.9659258262890683122, 1.000000000000000000, 0.9659258262890683122, 1.000000000000000000, 0.9659258262890683122, 1.000000000000000000, 0.9659258262890683122, 1.000000000000000000, 0.9659258262890683122, 1.000000000000000000, 0.9659258262890683122, 1.000000000000000000, 0.9659258262890683122, 1.000000000000000000, 0.9659258262890683122, 1.000000000000000000, 0.9659258262890683122, 1.000000000000000000, 0.9659258262890683122, 1.000000000000000000, 0.9659258262890683122, 1.000000000000000000, 0.9659258262890683122, 1.000000000000000000, 0.9659258262890683122, 1.000000000000000000, 0.9659258262890683122, 1.000000000000000000, 0.9659258262890683122, 1.000000000000000000, 0.9659258262890683122, 1.000000000000000000, 0.9659258262890683122, 1.000000000000000000, 0.9659258262890683122, 1.000000000000000000, 0.9659258262890683122, 1.000000000000000000, 0.9659258262890683122, 1.000000000000000000, 0.9659258262890683122, 1.000000000000000000, 0.9659258262890683122, 1.000000000000000000, 0.9659258262890683122, 1.000000000000000000, 0.9659258262890683122, 1.000000000000000000, 0.9659258262890683122, 1.000000000000000000, 0.9659258262890683122, 1.000000000000000000, 0.9659258262890683122, 1.000000000000000000, 0.9659258262890683122, 1.000000000000000000, 0.9659258262890683122, 1.000000000000000000, 0.9659258262890683122, 1.000000000000000000, 0.9659258262890683122, 1.000000000000000000, 0.9659258262890683122, 1.000000000000000000, 0.9659258262890683122, 1.000000000000000000, 0.9659258262890683122, 1.000000000000000000, 0.9659258262890683122, 1.000000000000000000, 0.9659258262890683122, 1.000000000000000000, 0.9659258262890683122, 1.000000000000000000, 0.9659258262890683122, 1.000000000000000000, 0.9659258262890683122, 1.000000000000000000, 0.9659258262890683122, 1.000000000000000000, 0.9659258262890683122, 1.000000000000000000, 0.9659258262890683122, 1.000000000000000000, 0.9659258262890683122, 1.000000000000000000, 0.9659258262890683122, 1.000000000000000000, 0.9659258262890683122, 1.000000000000000000, 0.9659258262890683122, 1.000000000000000000, 0.9659258262890683122, 1.000000000000000000, 0.9659258262890683122, 1.000000000000000000, 0.9659258262890683122, 1.000000000000000000, 0.9659258262890683122, 1.000000000000000000, 0.9659258262890683122, 1.000000000000000000, 0.9659258262890683122, 1.000000000000000000, 0.9659258262890683122, 1.000000000000000000, 0.9659258262890683122, 1.000000000000000000, 0.9659258262890683122, 1.000000000000000000, 0.9659258262890683122, 1.000000000000000000, 0.9659258262890683122, 1.000000000000000000, 0.9659258262890683122, 1.000000000000000000, 0.9659258262890683122, 1.000000000000000000, 0.9659258262890683122, 1.000000000000000000, 0.9659258262890683122, 1.000000000000000000, 0.9659258262890683122, 1.000000000000000000, 0.9659258262890683122, 1.000000000000000000, 0.9659258262890683122, 1.000000000000000000, 0.9659258262890683122, 1.000000000000000000, 0.9659258262890683122, 1.000000000000000000, 0.9659258262890683122, 1.000000000000000000, 0.9659258262890683122, 1.000000000000000000, 0.9659258262890683122, 1.000000000000000000, 0.9659258262890683122, 1.000000000000000000, 0.9659258262890683122, 1.000000000000000000, 0.9659258262890683122, 1.000000000000000000, 0.9659258262890683122, 1.000000000000000000, 0.9659258262890683122, 1.000000000000000000, 0.9659258262890683122, 1.000000000000000000, 0.9659258262890683122, 1.000000000000000000, 0.9659258262890683122, 1.000000000000000000, 0.9659258262890683122, 1.000000000000000000, 0.9659258262890683122, 1.000000000000000000, 0.9659258262890683122, 1.000000000000000000, 0.9659258262890683122, 1.000000000000000000, 0.9659258262890683122, 1.000000000000000000, 0.9659258262890683122, 1.000000000000000000, 0.9659258262890683122, 1.000000000000000000, 0.9659258262890683122, 1.000000000000000000, 0.9659258262890683122, 1.000000000000000000, 0.9659258262890683122, 1.000000000000000000, 0.9659258262890683122, 1.000000000000000000, 0.9659258262890683122, 1.000000000000000000, 0.9659258262890683122, 1.000000000000000000, 0.9659258262890683122, 1.000000000000000000, 0.9659258262890683122, 1.000000000000000000, 0.9659258262890683122, 1.000000000000000000, 0.9659258262890683122, 1.000000000000000000, 0.9659258262890683122, 1.000000000000000000, 0.9659258262890683122, 1.000000000000000000, 0.9659258262890683122, 1.000000000000000000, 0.9659258262890683122, 1.000000000000000000, 0.9659258262890683122, 1.000000000000000000, 0.9659258262890683122, 1.000000000000000000, 0.9659258262890683122, 1.000000000000000000, 0.9659258262890683122, 1.000000000000000000, 0.9659258262890683122, 1.000000000000000000, 0.9659258262890683122, 1.000000000000000000, 0.9659258262890683122, 1.000000000000000000, 0.9659258262890683122, 1.000000000000000000, 0.9659258262890683122, 1.000000000000000000, 0.9659258262890683122, 1.000000000000000000, 0.9659258262890683122, 1.000000000000000000, 0.9659258262890683122, 1.000000000000000000, 0.9659258262890683122, 1.000000000000000000, 0.9659258262890683122, 1.000000000000000000, 0.9659258262890683122, 1.000000000000000000, 0.9659258262890683122, 1.000000000000000000, 0.9659258262890683122, 1.000000000000000000, 0.9659258262890683122, 1.000000000000000000, 0.9659258262890683122, 1.000000000000000000, 0.9659258262890683122, 1.000000000000000000, 0.9659258262890683122, 1.000000000000000000, 0.9659258262890683122, 1.000000000000000000, 0.9659258262890683122, 1.000000000000000000, 0.9659258262890683122, 1.000000000000000000, 0.9659258262890683122, 1.000000000000000000, 0.9659258262890683122, 1.000000000000000000, 0.9659258262890683122, 1.000000000000000000, 0.9659258262890683122, 1.000000000000000000, 0.9659258262890683122, 1.000000000000000000, 0.9659258262890683122, 1.000000000000000000, 0.9659258262890683122, 1.000000000000000000, 0.9659258262890683122, 1.000000000000000000, 0.9659258262890683122, 1.000000000000000000, 0.9659258262890683122, 1.000000000000000000, 0.9659258262890683122, 1.000000000000000000, 0.9659258262890683122, 1.000000000000000000, 0.9659258262890683122, 1.000000000000000000, 0.9659258262890683122, 1.000000000000000000, 0.9659258262890683122, 1.000000000000000000, 0.9659258262890683122, 1.000000000000000000, 0.9659258262890683122, 1.000000000000000000, 0.9659258262890683122, 1.000000000000000000, 0.9659258262890683122, 1.000000000000000000, 0.9659258262890683122, 1.000000000000000000, 0.9659258262890683122, 1.000000000000000000, 0.9659258262890683122, 1.000000000000000000, 0.9659258262890683122, 1.000000000000000000, 0.9659258262890683122, 1.000000000000000000, 0.9659258262890683122, 1.000000000000000000, 0.9659258262890683122, 1.000000000000000000, 0.9659258262890683122, 1.000000000000000000, 0.9659258262890683122, 1.000000000000000000, 0.9659258262890683122, 1.000000000000000000, 0.9659258262890683122, 1.000000000000000000, 0.9659258262890683122, 1.000000000000000000, 0.9659258262890683122, 1.000000000000000000, 0.9659258262890683122, 1.000000000000000000, 0.9659258262890683122, 1.000000000000000000, 0.9659258262890683122, 1.000000000000000000, 0.9659258262890683122, 1.000000000000000000, 0.9659258262890683122, 1.000000000000000000, 0.9659258262890683122, 1.000000000000000000, 0.9659258262890683122, 1.000000000000000000, 0.9659258262890683122, 1.000000000000000000, 0.9659258262890683122, 1.000000000000000000, 0.9659258262890683122, 1.000000000000000000, 0.9659258262890683122, 1.000000000000000000, 0.9659258262890683122, 1.000000000000000000, 0.9659258262890683122, 1.000000000000000000, 0.9659258262890683122, 1.000000000000000000, 0.9659258262890683122, 1.000000000000000000, 0.9659258262890683122, 1.000000000000000000, 0.9659258262890683122, 1.000000000000000000, 0.9659258262890683122, 1.000000000000000000, 0.9659258262890683122, 1.000000000000000000, 0.9659258262890683122, 1.000000000000000000, 0.9659258262890683122, 1.000000000000000000, 0.9659258262890683122, 1.000000000000000000, 0.9659258262890683122, 1.000000000000000000, 0.9659258262890683122, 1.000000000000000000, 0.9659258262890683122, 1.000000000000000000, 0.9659258262890683122, 1.000000000000000000, 0.9659258262890683122, 1.000000000000000000, 0.9659258262890683122, 1.000000000000000000, 0.9659258262890683122, 1.000000000000000000, 0.9659258262890683122, 1.000000000000000000, 0.9659258262890683122, 1.000000000000000000, 0.9659258262890683122, 1.000000000000000000, 0.9659258262890683122, 1.000000000000000000, 0.9659258262890683122, 1.000000000000000000, 0.9659258262890683122, 1.000000000000000000, 0.9659258262890683122, 1.000000000000000000, 0.9659258262890683122, 1.000000000000000000, 0.9659258262890683122, 1.000000000000000000, 0.9659258262890683122, 1.000000000000000000, 0.9659258262890683122, 1.000000000000000000, 0.9659258262890683122, 1.000000000000000000, 0.9659258262890683122, 1.000000000000000000, 0.9659258262890683122, 1.000000000000000000, 0.9659258262890683122, 1.000000000000000000, 0.9659258262890683122, 1.000000000000000000, 0.9659258262890683122, 1.000000000000000000, 0.9659258262890683122, 1.000000000000000000, 0.9659258262890683122, 1.000000000000000000, 0.9659258262890683122, 1.000000000000000000, 0.9659258262890683122, 1.000000000000000000, 0.9659258262890683122, 1.000000000000000000, 0.9659258262890683122, 1.000000000000000000, 0.9659258262890683122, 1.000000000000000000, 0.9659258262890683122, 1.000000000000000000, 0.9659258262890683122, 1.000000000000000000, 0.9659258262890683122, 1.000000000000000000, 0.9659258262890683122, 1.000000000000000000, 0.9659258262890683122, 1.000000000000000000, 0.9659258262890683122, 1.000000000000000000, 0.9659258262890683122, 1.000000000000000000, 0.9659258262890683122, 1.000000000000000000, 0.9659258262890683122, 1.000000000000000000, 0.9659258262890683122, 1.000000000000000000, 0.9659258262890683122, 1.000000000000000000, 0.9659258262890683122, 1.000000000000000000, 0.9659258262890683122, 1.000000000000000000, 0.9659258262890683122, 1.000000000000000000, 0.9659258262890683122, 1.000000000000000000, 0.9659258262890683122, 1.000000000000000000, 0.9659258262890683122, 1.000000000000000000, 0.9659258262890683122, 1.000000000000000000, 0.9659258262890683122, 1.000000000000000000, 0.9659258262890683122, 1.000000000000000000, 0.9659258262890683122, 1.000000000000000000, 0.9659258262890683122, 1.000000000000000000, 0.9659258262890683122, 1.000000000000000000, 0.9659258262890683122, 1.000000000000000000, 0.9659258262890683122, 1.000000000000000000, 0.9659258262890683122, 1.000000000000000000, 0.9659258262890683122, 1.000000000000000000, 0.9659258262890683122, 1.000000000000000000, 0.9659258262890683122, 1.000000000000000000, 0.9659258262890683122, 1.000000000000000000, 0.9659258262890683122, 1.000000000000000000, 0.9659258262890683122, 1.000000000000000000, 0.9659258262890683122, 1.000000000000000000, 0.9659258262890683122, 1.000000000000000000, 0.9659258262890683122, 1.000000000000000000, 0.9659258262890683122, 1.000000000000000000, 0.9659258262890683122, 1.000000000000000000, 0.9659258262890683122, 1.000000000000000000, 0.9659258262890683122, 1.000000000000000000, 0.9659258262890683122, 1.000000000000000000, 0.9659258262890683122, 1.000000000000000000, 0.9659258262890683122, 1.000000000000000000, 0.9659258262890683122, 1.000000000000000000, 0.9659258262890683122, 1.000000000000000000, 0.9659258262890683122, 1.000000000000000000, 0.9659258262890683122, 1.000000000000000000, 0.9659258262890683122, 1.000000000000000000, 0.9659258262890683122, 1.000000000000000000, 0.9659258262890683122, 1.000000000000000000, 0.9659258262890683122, 1.000000000000000000, 0.9659258262890683122, 1.000000000000000000, 0.9659258262890683122, 1.000000000000000000, 0.9659258262890683122, 1.000000000000000000, 0.9659258262890683122, 1.000000000000000000, 0.9659258262890683122, 1.000000000000000000, 0.9659258262890683122, 1.000000000000000000, 0.9659258262890683122, 1.000000000000000000, 0.9659258262890683122, 1.000000000000000000, 0.9659258262890683122, 1.000000000000000000, 0.9659258262890683122, 1.000000000000000000, 0.9659258262890683122, 1.000000000000000000, 0.9659258262890683122, 1.000000000000000000, 0.9659258262890683122, 1.000000000000000000, 0.9659258262890683122, 1.000000000000000000, 0.9659258262890683122, 1.000000000000000000, 0.9659258262890683122, 1.000000000000000000, 0.9659258262890683122, 1.000000000000000000) ) ) 
 REPRESENTATION_ITEM ( '' )  SURFACE ( )  );
#82348=CYLINDRICAL_SURFACE ( 'NONE', #63652, 4.375000000000001776 ) ;
#82387=CARTESIAN_POINT ( 'NONE',  ( 71.07876352523146579, -7.482591942790327058E-16, 6.109999999999999432 ) ) ;
#82404=VERTEX_POINT ( 'NONE', #85042 ) ;
#82406=CARTESIAN_POINT ( 'NONE',  ( 91.07919371712955581, 3.975000000000002753, -6.884901960086283523 ) ) ;
#82419=CARTESIAN_POINT ( 'NONE',  ( 80.35459685856474721, -1.637169565754161615, 6.110000000000000320 ) ) ;
#82427=CARTESIAN_POINT ( 'NONE',  ( 118.3500270504628986, -5.819803920172573086, -5.819803920172573086 ) ) ;
#82442=CARTESIAN_POINT ( 'NONE',  ( 79.62543019189810423, 5.291415217122919401, 3.055000000000002824 ) ) ;
#82485=CARTESIAN_POINT ( 'NONE',  ( 27.00000000000001066, -4.901040733167808305, -4.492499863940687455 ) ) ;
#82497=CARTESIAN_POINT ( 'NONE',  ( 71.31293019189810423, -1.637169565754159617, -6.110000000000001208 ) ) ;
#82499=CARTESIAN_POINT ( 'NONE',  ( 94.91666666666665719, -6.884901960086287076, -3.975000000000000977 ) ) ;
#82501=CARTESIAN_POINT ( 'NONE',  ( 112.5837635252314470, -6.110000000000001208, -3.741295971395164515E-16 ) ) ;
#82548=CARTESIAN_POINT ( 'NONE',  ( 73.18749999999997158, -5.819803920172573974, 5.819803920172573086 ) ) ;
#82565=CARTESIAN_POINT ( 'NONE',  ( 107.7500000000000000, -9.735942053221458872E-16, 7.950000000000000178 ) ) ;
#82566=CARTESIAN_POINT ( 'NONE',  ( 122.7250270504628844, 5.819803920172573086, -5.819803920172572198 ) ) ;
#82579=CARTESIAN_POINT ( 'NONE',  ( 84.85416666666668561, -2.130196079827425315, -7.950000000000001066 ) ) ;
#82590=CARTESIAN_POINT ( 'NONE',  ( 126.8620668341126674, 3.744568938377744960, 5.426115537218553442 ) ) ;
#82605=CARTESIAN_POINT ( 'NONE',  ( 112.2920968585647756, -5.291415217122921177, 3.054999999999999272 ) ) ;
#82607=VERTEX_POINT ( 'NONE', #45154 ) ;
#82610=AXIS2_PLACEMENT_3D ( 'NONE', #27669, #106641, #50164 ) ;
#82616=( BOUNDED_CURVE ( )  B_SPLINE_CURVE ( 2, ( #55967, #100166, #815, #111752, #56698, #100861, #61504, #6306, #126021, #116557, #28126, #83222, #126697 ),
 .UNSPECIFIED., .F., .F. ) 
 B_SPLINE_CURVE_WITH_KNOTS ( ( 3, 2, 2, 2, 2, 2, 3 ),
 ( 0.8833333333333333037, 0.8861111111111110716, 0.8888888888888888395, 0.8916666666666667185, 0.8944444444444444864, 0.8972222222222222543, 0.9000000000000000222 ),
 .UNSPECIFIED. ) 
 CURVE ( )  GEOMETRIC_REPRESENTATION_ITEM ( )  RATIONAL_B_SPLINE_CURVE ( ( 1.000000000000000000, 0.9659258262890683122, 1.000000000000000000, 0.9659258262890683122, 1.000000000000000000, 0.9659258262890683122, 1.000000000000000000, 0.9659258262890683122, 1.000000000000000000, 0.9659258262890683122, 1.000000000000000000, 0.9659258262890683122, 1.000000000000000000 ) ) 
 REPRESENTATION_ITEM ( '' )  );
#82618=CARTESIAN_POINT ( 'NONE',  ( 107.3912635252314516, -4.472830434245839371, -4.472830434245839371 ) ) ;
#82674=CARTESIAN_POINT ( 'NONE',  ( 40.16209685856478018, -5.291415217122919401, 3.054999999999997939 ) ) ;
#82708=CARTESIAN_POINT ( 'NONE',  ( 101.7037635252314374, 6.109999999999999432, 1.122388791418549108E-15 ) ) ;
#82711=LINE ( 'NONE', #5815, #122983 ) ;
#82752=CARTESIAN_POINT ( 'NONE',  ( 27.78752705046289151, 0.000000000000000000, -7.949999999999998401 ) ) ;
#82757=CARTESIAN_POINT ( 'NONE',  ( 118.9791666666666430, -7.950000000000001066, 2.130196079827424427 ) ) ;
#82771=CARTESIAN_POINT ( 'NONE',  ( 116.8129301918981184, -1.637169565754159617, -6.110000000000001208 ) ) ;
#82777=CARTESIAN_POINT ( 'NONE',  ( 82.76669371712954160, -7.949999999999998401, 2.130196079827423983 ) ) ;
#82779=AXIS2_PLACEMENT_3D ( 'NONE', #101372, #46328, #102821 ) ;
#82783=CARTESIAN_POINT ( 'NONE',  ( 35.07919371712955581, 3.975000000000002753, -6.884901960086283523 ) ) ;
#82791=CARTESIAN_POINT ( 'NONE',  ( 37.45833333333332860, 3.974999999999997424, 6.884901960086288852 ) ) ;
#82805=CARTESIAN_POINT ( 'NONE',  ( 32.22959685856477563, -6.110000000000000320, -1.637169565754161393 ) ) ;
#82816=CARTESIAN_POINT ( 'NONE',  ( 59.64626352523142572, -4.472830434245840259, 4.472830434245839371 ) ) ;
#82817=EDGE_CURVE ( 'NONE', #66568, #44417, #55545, .T. ) ;
#82827=CARTESIAN_POINT ( 'NONE',  ( 46.87043019189811588, -3.055000000000001492, 5.291415217122917625 ) ) ;
#82847=VERTEX_POINT ( 'NONE', #97897 ) ;
#82853=CARTESIAN_POINT ( 'NONE',  ( 69.91209685856478018, 5.291415217122921177, -3.054999999999994831 ) ) ;
#82902=FACE_BOUND ( 'NONE', #98263, .T. ) ;
#82910=DIRECTION ( 'NONE',  ( -1.000000000000000000, -0.000000000000000000, -0.000000000000000000 ) ) ;
#82927=CARTESIAN_POINT ( 'NONE',  ( 50.22459685856477307, -1.637169565754161171, 6.109999999999998543 ) ) ;
#82943=CARTESIAN_POINT ( 'NONE',  ( 103.7666937171295416, -7.949999999999998401, 2.130196079827423983 ) ) ;
#82944=CARTESIAN_POINT ( 'NONE',  ( 68.32919371712955581, -3.975000000000001865, 6.884901960086284411 ) ) ;
#82950=CARTESIAN_POINT ( 'NONE',  ( 65.16666666666667140, 6.884901960086285300, 3.975000000000003642 ) ) ;
#82957=CARTESIAN_POINT ( 'NONE',  ( 33.37499999999998579, 7.950000000000000178, 1.460391307983218535E-15 ) ) ;
#82960=CARTESIAN_POINT ( 'NONE',  ( 53.08376352523143282, -6.110000000000001208, -3.741295971395164515E-16 ) ) ;
#82986=CARTESIAN_POINT ( 'NONE',  ( 124.0375270504628986, -9.735942053221456900E-16, 7.949999999999998401 ) ) ;
#82993=DIRECTION ( 'NONE',  ( 0.000000000000000000, 0.000000000000000000, 1.000000000000000000 ) ) ;
#82999=CARTESIAN_POINT ( 'NONE',  ( 61.18336038379621300, -2.130196079827426203, 7.949999999999996625 ) ) ;
#83014=CARTESIAN_POINT ( 'NONE',  ( 93.97459685856478018, 1.637169565754164280, -6.109999999999996767 ) ) ;
#83038=CARTESIAN_POINT ( 'NONE',  ( 44.77126352523143282, 4.472830434245838482, 4.472830434245842035 ) ) ;
#83074=CARTESIAN_POINT ( 'NONE',  ( 26.45376352523144803, -6.109999999999998543, -3.741295971395162543E-16 ) ) ;
#83079=VERTEX_POINT ( 'NONE', #141039 ) ;
#83080=ORIENTED_EDGE ( 'NONE', *, *, #42734, .F. ) ;
#83083=CARTESIAN_POINT ( 'NONE',  ( 94.43336038379622721, 2.130196079827431532, -7.949999999999996625 ) ) ;
#83087=CARTESIAN_POINT ( 'NONE',  ( 78.51626352523145158, -4.472830434245839371, 4.472830434245839371 ) ) ;
#83089=CARTESIAN_POINT ( 'NONE',  ( 80.04166666666665719, -3.975000000000002753, 6.884901960086286188 ) ) ;
#83095=ORIENTED_EDGE ( 'NONE', *, *, #125081, .T. ) ;
#83109=ORIENTED_EDGE ( 'NONE', *, *, #71408, .T. ) ;
#83110=AXIS2_PLACEMENT_3D ( 'NONE', #52934, #55843, #8686 ) ;
#83113=CARTESIAN_POINT ( 'NONE',  ( 95.74586038379622721, 3.974999999999996980, 6.884901960086287964 ) ) ;
#83114=CARTESIAN_POINT ( 'NONE',  ( 71.58333333333332860, 6.884901960086290629, -3.974999999999994316 ) ) ;
#83128=CARTESIAN_POINT ( 'NONE',  ( 46.16252705046289151, 7.949999999999998401, 1.460391307983218338E-15 ) ) ;
#83130=CARTESIAN_POINT ( 'NONE',  ( 87.64626352523141861, -4.472830434245840259, 4.472830434245839371 ) ) ;
#83142=VERTEX_POINT ( 'NONE', #98272 ) ;
#83149=CARTESIAN_POINT ( 'NONE',  ( 72.91709685856477563, 3.054999999999998828, 5.291415217122922066 ) ) ;
#83177=CARTESIAN_POINT ( 'NONE',  ( 52.72502705046289151, 5.819803920172573974, -5.819803920172573086 ) ) ;
#83208=CARTESIAN_POINT ( 'NONE',  ( 75.83376352523144703, 6.110000000000001208, 1.122388791418549305E-15 ) ) ;
#83214=CARTESIAN_POINT ( 'NONE',  ( 105.1462635252314470, -4.472830434245840259, 4.472830434245838482 ) ) ;
#83222=CARTESIAN_POINT ( 'NONE',  ( 34.93336038379622011, 2.130196079827431532, -7.949999999999996625 ) ) ;
#83228=VERTEX_POINT ( 'NONE', #98955 ) ;
#83229=CARTESIAN_POINT ( 'NONE',  ( 114.9958603837962272, -3.974999999999998312, -6.884901960086286188 ) ) ;
#83230=ORIENTED_EDGE ( 'NONE', *, *, #84150, .F. ) ;
#83232=CARTESIAN_POINT ( 'NONE',  ( 114.7500000000000000, -9.735942053221458872E-16, 7.950000000000000178 ) ) ;
#83236=ORIENTED_EDGE ( 'NONE', *, *, #120413, .F. ) ;
#83237=EDGE_CURVE ( 'NONE', #102725, #20835, #131614, .T. ) ;
#83278=CARTESIAN_POINT ( 'NONE',  ( 117.6208603837962272, -6.884901960086286188, 3.974999999999997424 ) ) ;
#83297=CARTESIAN_POINT ( 'NONE',  ( 79.02083333333332860, 7.949999999999999289, 2.130196079827431532 ) ) ;
#83303=CARTESIAN_POINT ( 'NONE',  ( 30.26669371712955936, -7.949999999999998401, 2.130196079827423983 ) ) ;
#83325=CARTESIAN_POINT ( 'NONE',  ( 100.4795968585647614, 6.109999999999999432, 1.637169565754164280 ) ) ;
#83332=EDGE_CURVE ( 'NONE', #77939, #36177, #138981, .T. ) ;
#83335=CARTESIAN_POINT ( 'NONE',  ( 103.7454301918981230, -5.291415217122918513, -3.055000000000000160 ) ) ;
#83359=CARTESIAN_POINT ( 'NONE',  ( 115.1204301918981230, 3.055000000000001936, -5.291415217122916737 ) ) ;
#83385=CARTESIAN_POINT ( 'NONE',  ( 26.89126352523144092, -4.472830434245838482, -4.472830434245838482 ) ) ;
#83402=VERTEX_POINT ( 'NONE', #48168 ) ;
#83425=CARTESIAN_POINT ( 'NONE',  ( 104.0370968585647802, -3.054999999999999272, -5.291415217122919401 ) ) ;
#83428=DIRECTION ( 'NONE',  ( -1.000000000000000000, -0.000000000000000000, -0.000000000000000000 ) ) ;
#83461=CARTESIAN_POINT ( 'NONE',  ( 47.52083333333332860, 7.949999999999998401, 2.130196079827431532 ) ) ;
#83473=CARTESIAN_POINT ( 'NONE',  ( 115.1874999999999716, -5.819803920172573086, 5.819803920172572198 ) ) ;
#83493=CARTESIAN_POINT ( 'NONE',  ( 113.7504301918981042, 3.055000000000002824, -5.291415217122919401 ) ) ;
#83503=CARTESIAN_POINT ( 'NONE',  ( 38.28752705046288440, 0.000000000000000000, -7.949999999999998401 ) ) ;
#83508=CARTESIAN_POINT ( 'NONE',  ( 31.91666666666666430, -6.884901960086287076, -3.975000000000000977 ) ) ;
#83513=CARTESIAN_POINT ( 'NONE',  ( 40.03752705046288440, -9.735942053221456900E-16, 7.949999999999998401 ) ) ;
#83518=AXIS2_PLACEMENT_3D ( 'NONE', #124539, #1991, #111513 ) ;
#83520=CARTESIAN_POINT ( 'NONE',  ( 30.33376352523143993, 6.110000000000001208, 1.122388791418549305E-15 ) ) ;
#83530=CARTESIAN_POINT ( 'NONE',  ( 63.41666666666666430, -6.884901960086287076, -3.975000000000000977 ) ) ;
#83533=CARTESIAN_POINT ( 'NONE',  ( 54.68793019189810423, 6.110000000000002984, -1.637169565754156730 ) ) ;
#83542=CARTESIAN_POINT ( 'NONE',  ( 47.45376352523145158, -6.109999999999998543, -3.741295971395162543E-16 ) ) ;
#83572=CARTESIAN_POINT ( 'NONE',  ( 67.43293019189810877, 1.637169565754156508, 6.110000000000000320 ) ) ;
#83574=CARTESIAN_POINT ( 'NONE',  ( 0.000000000000000000, 0.000000000000000000, 0.000000000000000000 ) ) ;
#83580=CARTESIAN_POINT ( 'NONE',  ( 34.97916666666665009, -7.950000000000000178, 2.130196079827424427 ) ) ;
#83581=CARTESIAN_POINT ( 'NONE',  ( 101.7708333333333428, -7.949999999999998401, -2.130196079827426203 ) ) ;
#83631=DIRECTION ( 'NONE',  ( 0.000000000000000000, 0.000000000000000000, 1.000000000000000000 ) ) ;
#83660=CARTESIAN_POINT ( 'NONE',  ( 42.49543019189810877, 5.291415217122917625, 3.055000000000002380 ) ) ;
#83684=CARTESIAN_POINT ( 'NONE',  ( 61.62086038379622721, -6.884901960086286188, 3.974999999999997424 ) ) ;
#83688=CARTESIAN_POINT ( 'NONE',  ( 64.14583333333334281, 2.130196079827431976, -7.949999999999999289 ) ) ;
#83699=CARTESIAN_POINT ( 'NONE',  ( 58.04209685856477563, 5.291415217122923842, -3.054999999999996163 ) ) ;
#83754=CARTESIAN_POINT ( 'NONE',  ( 90.32876352523145158, 0.000000000000000000, -6.109999999999998543 ) ) ;
#83774=ORIENTED_EDGE ( 'NONE', *, *, #70004, .T. ) ;
#83777=CARTESIAN_POINT ( 'NONE',  ( 49.00043019189810423, -3.055000000000002380, 5.291415217122920289 ) ) ;
#83797=DIRECTION ( 'NONE',  ( -1.000000000000000000, -0.000000000000000000, -0.000000000000000000 ) ) ;
#83833=CARTESIAN_POINT ( 'NONE',  ( 76.47459685856476597, 1.637169565754164280, -6.109999999999997655 ) ) ;
#83839=FACE_OUTER_BOUND ( 'NONE', #142568, .T. ) ;
#83859=CARTESIAN_POINT ( 'NONE',  ( 97.93336038379622721, 2.130196079827431532, -7.949999999999997513 ) ) ;
#83871=CARTESIAN_POINT ( 'NONE',  ( 46.45419371712955581, 6.884901960086283523, 3.975000000000002753 ) ) ;
#83874=CARTESIAN_POINT ( 'NONE',  ( 86.91709685856477563, 3.054999999999998828, 5.291415217122922066 ) ) ;
#83893=CARTESIAN_POINT ( 'NONE',  ( 69.70876352523144703, -7.482591942790329030E-16, 6.110000000000001208 ) ) ;
#83909=EDGE_CURVE ( 'NONE', #133316, #96308, #37854, .T. ) ;
#83924=CARTESIAN_POINT ( 'NONE',  ( 53.16252705046288440, 7.949999999999998401, 1.460391307983218338E-15 ) ) ;
#83951=CARTESIAN_POINT ( 'NONE',  ( 68.68793019189809002, 6.110000000000002984, -1.637169565754156730 ) ) ;
#83956=CARTESIAN_POINT ( 'NONE',  ( 105.2920968585647756, -5.291415217122921177, 3.054999999999999272 ) ) ;
#83973=CARTESIAN_POINT ( 'NONE',  ( 1.500000000000000000, 9.797174393178827630E-16, 8.000000000000001776 ) ) ;
#83990=CARTESIAN_POINT ( 'NONE',  ( 13.61880637382470383, -9.051169013344379621, 2.893211955101936628 ) ) ;
#83993=VERTEX_POINT ( 'NONE', #98622 ) ;
#84008=CARTESIAN_POINT ( 'NONE',  ( 72.89583333333331439, -2.130196079827427091, 7.949999999999998401 ) ) ;
#84025=CARTESIAN_POINT ( 'NONE',  ( 124.1833603837961988, -2.130196079827426203, 7.949999999999997513 ) ) ;
#84040=CARTESIAN_POINT ( 'NONE',  ( 82.37500000000000000, 7.950000000000000178, 1.460391307983218535E-15 ) ) ;
#84047=CARTESIAN_POINT ( 'NONE',  ( 30.99586038379621655, -3.974999999999998312, -6.884901960086286188 ) ) ;
#84064=CARTESIAN_POINT ( 'NONE',  ( 102.2295968585647614, -6.110000000000000320, -1.637169565754161393 ) ) ;
#84072=CARTESIAN_POINT ( 'NONE',  ( 74.64583333333331439, 2.130196079827431976, -7.949999999999998401 ) ) ;
#84074=CARTESIAN_POINT ( 'NONE',  ( 98.78709685856479439, 3.054999999999997495, 5.291415217122919401 ) ) ;
#84099=CARTESIAN_POINT ( 'NONE',  ( 113.9537635252314516, -6.109999999999998543, -3.741295971395162543E-16 ) ) ;
#84113=CARTESIAN_POINT ( 'NONE',  ( 36.58333333333332860, 6.884901960086290629, -3.974999999999994316 ) ) ;
#84114=ORIENTED_EDGE ( 'NONE', *, *, #28303, .F. ) ;
#84122=CARTESIAN_POINT ( 'NONE',  ( 31.55793019189810522, 6.110000000000000320, -1.637169565754156064 ) ) ;
#84150=EDGE_CURVE ( 'NONE', #129167, #46218, #110121, .T. ) ;
#84161=CARTESIAN_POINT ( 'NONE',  ( 105.9329301918981088, 1.637169565754156730, 6.110000000000001208 ) ) ;
#84210=CARTESIAN_POINT ( 'NONE',  ( 114.7500000000000000, -9.735942053221458872E-16, 7.950000000000000178 ) ) ;
#84212=ORIENTED_EDGE ( 'NONE', *, *, #10376, .F. ) ;
#84222=CARTESIAN_POINT ( 'NONE',  ( 105.5837635252314328, -6.110000000000001208, -3.741295971395164515E-16 ) ) ;
#84231=CARTESIAN_POINT ( 'NONE',  ( 41.20419371712954870, -6.884901960086285300, -3.975000000000000089 ) ) ;
#84237=CARTESIAN_POINT ( 'NONE',  ( 26.66666666666665719, 6.884901960086285300, 3.975000000000003642 ) ) ;
#84246=CARTESIAN_POINT ( 'NONE',  ( 121.9745968585647802, 1.637169565754164058, -6.109999999999996767 ) ) ;
#84257=CARTESIAN_POINT ( 'NONE',  ( 43.16709685856477563, -3.055000000000000160, -5.291415217122921177 ) ) ;
#84269=CARTESIAN_POINT ( 'NONE',  ( 51.97459685856478728, 1.637169565754164058, -6.109999999999996767 ) ) ;
#84281=CARTESIAN_POINT ( 'NONE',  ( 44.41252705046289151, -7.949999999999998401, -4.867971026610728450E-16 ) ) ;
#84296=CARTESIAN_POINT ( 'NONE',  ( 52.12043019189811588, 3.055000000000001936, -5.291415217122916737 ) ) ;
#84306=CARTESIAN_POINT ( 'NONE',  ( 35.56249999999999289, -5.819803920172573086, -5.819803920172573974 ) ) ;
#84351=( BOUNDED_CURVE ( )  B_SPLINE_CURVE ( 2, ( #86315, #130537, #51547 ),
 .UNSPECIFIED., .F., .T. ) 
 B_SPLINE_CURVE_WITH_KNOTS ( ( 3, 3 ),
 ( 0.9499999999999999556, 0.9523725280802812776 ),
 .UNSPECIFIED. ) 
 CURVE ( )  GEOMETRIC_REPRESENTATION_ITEM ( )  RATIONAL_B_SPLINE_CURVE ( ( 1.000000000000000000, 0.9708969037810349922, 0.9915083049239592494 ) ) 
 REPRESENTATION_ITEM ( '' )  );
#84372=CARTESIAN_POINT ( 'NONE',  ( 42.34959685856478018, 6.109999999999997655, 1.637169565754163836 ) ) ;
#84393=CARTESIAN_POINT ( 'NONE',  ( 68.03752705046289861, -9.735942053221456900E-16, 7.949999999999998401 ) ) ;
#84397=CARTESIAN_POINT ( 'NONE',  ( 51.74999999999999289, -9.735942053221458872E-16, 7.950000000000000178 ) ) ;
#84404=CARTESIAN_POINT ( 'NONE',  ( 61.39626352523143993, 4.472830434245840259, -4.472830434245839371 ) ) ;
#84424=EDGE_CURVE ( 'NONE', #2806, #53423, #50885, .T. ) ;
#84428=EDGE_LOOP ( 'NONE', ( #136041, #17965 ) ) ;
#84430=CARTESIAN_POINT ( 'NONE',  ( 88.89169371712954160, 2.130196079827421762, 7.950000000000000178 ) ) ;
#84431=CARTESIAN_POINT ( 'NONE',  ( 72.97459685856478018, 1.637169565754164058, -6.109999999999996767 ) ) ;
#84460=CARTESIAN_POINT ( 'NONE',  ( 83.03709685856478018, -3.054999999999998828, -5.291415217122919401 ) ) ;
#84483=CARTESIAN_POINT ( 'NONE',  ( 33.68793019189809712, 6.110000000000002984, -1.637169565754156730 ) ) ;
#84511=CARTESIAN_POINT ( 'NONE',  ( 66.62499999999998579, -7.950000000000000178, -4.867971026610729436E-16 ) ) ;
#84532=CARTESIAN_POINT ( 'NONE',  ( 71.95376352523145158, -6.109999999999999432, -3.741295971395163529E-16 ) ) ;
#84554=CARTESIAN_POINT ( 'NONE',  ( 96.76669371712954160, -7.949999999999999289, 2.130196079827424427 ) ) ;
#84568=CARTESIAN_POINT ( 'NONE',  ( 84.14626352523144703, -4.472830434245840259, 4.472830434245839371 ) ) ;
#84586=CARTESIAN_POINT ( 'NONE',  ( 72.47959685856478984, 6.109999999999999432, 1.637169565754164280 ) ) ;
#84597=ORIENTED_EDGE ( 'NONE', *, *, #46585, .T. ) ;
#84634=CARTESIAN_POINT ( 'NONE',  ( 72.18793019189810423, 6.110000000000002984, -1.637169565754156730 ) ) ;
#84641=CARTESIAN_POINT ( 'NONE',  ( 113.3129301918981042, -1.637169565754159617, -6.110000000000001208 ) ) ;
#84650=CARTESIAN_POINT ( 'NONE',  ( 91.27083333333332860, -7.949999999999998401, -2.130196079827426203 ) ) ;
#84651=CARTESIAN_POINT ( 'NONE',  ( 77.51669371712954160, 7.950000000000000178, -2.130196079827421318 ) ) ;
#84684=CARTESIAN_POINT ( 'NONE',  ( 33.54209685856476852, 5.291415217122923842, -3.054999999999996163 ) ) ;
#84689=DIRECTION ( 'NONE',  ( -1.000000000000000000, -0.000000000000000000, -0.000000000000000000 ) ) ;
#84701=CARTESIAN_POINT ( 'NONE',  ( 93.26669371712955581, -7.949999999999998401, 2.130196079827423983 ) ) ;
#84703=CARTESIAN_POINT ( 'NONE',  ( 122.2875270504628844, 0.000000000000000000, -7.949999999999998401 ) ) ;
#84715=( BOUNDED_CURVE ( )  B_SPLINE_CURVE ( 2, ( #88337, #55712, #86901, #32524, #99162, #132579, #63736, #10727, #131119, #142012, #77475, #41969, #121641 ),
 .UNSPECIFIED., .F., .F. ) 
 B_SPLINE_CURVE_WITH_KNOTS ( ( 3, 2, 2, 2, 2, 2, 3 ),
 ( 0.7333333333333333925, 0.7361111111111112715, 0.7388888888888890394, 0.7416666666666666963, 0.7444444444444444642, 0.7472222222222222321, 0.7500000000000000000 ),
 .UNSPECIFIED. ) 
 CURVE ( )  GEOMETRIC_REPRESENTATION_ITEM ( )  RATIONAL_B_SPLINE_CURVE ( ( 0.9999999999999986677, 0.9659258262890696445, 1.000000000000000000, 0.9659258262890683122, 1.000000000000000000, 0.9659258262890683122, 1.000000000000000000, 0.9659258262890683122, 1.000000000000000000, 0.9659258262890683122, 1.000000000000000000, 0.9659258262890683122, 1.000000000000000000 ) ) 
 REPRESENTATION_ITEM ( '' )  );
#84717=CARTESIAN_POINT ( 'NONE',  ( 78.87500000000000000, 7.950000000000000178, 1.460391307983218535E-15 ) ) ;
#84742=CARTESIAN_POINT ( 'NONE',  ( 105.1462635252314612, -4.472830434245840259, 4.472830434245839371 ) ) ;
#84754=CARTESIAN_POINT ( 'NONE',  ( 95.43293019189809456, 1.637169565754156508, 6.110000000000000320 ) ) ;
#84819=ORIENTED_EDGE ( 'NONE', *, *, #3223, .F. ) ;
#84839=CARTESIAN_POINT ( 'NONE',  ( 88.87043019189810877, -3.055000000000001936, 5.291415217122918513 ) ) ;
#84854=FACE_OUTER_BOUND ( 'NONE', #142530, .T. ) ;
#84875=CARTESIAN_POINT ( 'NONE',  ( 46.64583333333333570, 2.130196079827508360, -7.949999999999954881 ) ) ;
#84880=CARTESIAN_POINT ( 'NONE',  ( 26.77392480454907897, 6.350000000000003197, 1.166476076187854416E-15 ) ) ;
#84884=EDGE_CURVE ( 'NONE', #96223, #82006, #85979, .T. ) ;
#84887=CARTESIAN_POINT ( 'NONE',  ( 107.1666666666666572, 6.884901960086285300, 3.975000000000003642 ) ) ;
#84898=CARTESIAN_POINT ( 'NONE',  ( 106.3129301918981042, -1.637169565754159617, -6.110000000000001208 ) ) ;
#84903=DIRECTION ( 'NONE',  ( -1.000000000000000000, -0.000000000000000000, -0.000000000000000000 ) ) ;
#84913=CARTESIAN_POINT ( 'NONE',  ( 27.68749999999998579, -5.819803920172573086, 5.819803920172572198 ) ) ;
#84925=CARTESIAN_POINT ( 'NONE',  ( 123.1412635252314374, 4.472830434245836706, 4.472830434245840259 ) ) ;
#84934=CARTESIAN_POINT ( 'NONE',  ( 48.41709685856476852, 3.054999999999998828, 5.291415217122922066 ) ) ;
#84946=CARTESIAN_POINT ( 'NONE',  ( 42.64126352523145158, 4.472830434245836706, 4.472830434245840259 ) ) ;
#84954=ORIENTED_EDGE ( 'NONE', *, *, #73083, .T. ) ;
#84974=CARTESIAN_POINT ( 'NONE',  ( 58.53709685856478728, -3.054999999999998828, -5.291415217122919401 ) ) ;
#85003=CARTESIAN_POINT ( 'NONE',  ( 124.5995968585647944, -6.109999999999998543, -1.637169565754160727 ) ) ;
#85012=CARTESIAN_POINT ( 'NONE',  ( 75.32919371712957002, -3.975000000000001865, 6.884901960086284411 ) ) ;
#85027=ORIENTED_EDGE ( 'NONE', *, *, #39376, .T. ) ;
#85042=CARTESIAN_POINT ( 'NONE',  ( 26.99999999999999645, 5.837062628940091535, 2.500239961634333596 ) ) ;
#85047=CARTESIAN_POINT ( 'NONE',  ( 35.93293019189811588, 1.637169565754156730, 6.110000000000001208 ) ) ;
#85070=DIRECTION ( 'NONE',  ( 0.000000000000000000, 0.000000000000000000, 1.000000000000000000 ) ) ;
#85072=CARTESIAN_POINT ( 'NONE',  ( 58.41252705046289151, -7.949999999999998401, -4.867971026610728450E-16 ) ) ;
#85077=CARTESIAN_POINT ( 'NONE',  ( 52.33333333333332860, -6.884901960086287964, 3.974999999999998312 ) ) ;
#85083=VERTEX_POINT ( 'NONE', #80565 ) ;
#85087=CARTESIAN_POINT ( 'NONE',  ( 51.33376352523143282, 6.110000000000001208, 1.122388791418549305E-15 ) ) ;
#85110=CARTESIAN_POINT ( 'NONE',  ( 63.05793019189810877, 6.110000000000000320, -1.637169565754156064 ) ) ;
#85122=ORIENTED_EDGE ( 'NONE', *, *, #98737, .T. ) ;
#85123=CARTESIAN_POINT ( 'NONE',  ( 65.75000000000000000, -9.735942053221458872E-16, 7.950000000000000178 ) ) ;
#85130=CARTESIAN_POINT ( 'NONE',  ( 40.32919371712954870, -3.975000000000001865, 6.884901960086284411 ) ) ;
#85140=CARTESIAN_POINT ( 'NONE',  ( 82.01626352523143737, -4.472830434245838482, 4.472830434245838482 ) ) ;
#85142=DIRECTION ( 'NONE',  ( 1.000000000000000000, 0.000000000000000000, 0.000000000000000000 ) ) ;
#85148=FACE_OUTER_BOUND ( 'NONE', #63144, .T. ) ;
#85153=( BOUNDED_CURVE ( )  B_SPLINE_CURVE ( 2, ( #102366, #110513, #86667, #76511, #54754, #33724, #130893, #99649, #14617, #103058, #33022, #119951, #10495 ),
 .UNSPECIFIED., .F., .T. ) 
 B_SPLINE_CURVE_WITH_KNOTS ( ( 3, 2, 2, 2, 2, 2, 3 ),
 ( 0.7000000000000000666, 0.7027777777777778345, 0.7055555555555557135, 0.7083333333333334814, 0.7111111111111112493, 0.7138888888888890172, 0.7166666666666667851 ),
 .UNSPECIFIED. ) 
 CURVE ( )  GEOMETRIC_REPRESENTATION_ITEM ( )  RATIONAL_B_SPLINE_CURVE ( ( 0.9999999999999986677, 0.9659258262890696445, 1.000000000000000000, 0.9659258262890683122, 1.000000000000000000, 0.9659258262890683122, 1.000000000000000000, 0.9659258262890683122, 1.000000000000000000, 0.9659258262890683122, 1.000000000000000000, 0.9659258262890669799, 1.000000000000001332 ) ) 
 REPRESENTATION_ITEM ( '' )  );
#85158=CARTESIAN_POINT ( 'NONE',  ( 39.08376352523143282, -6.110000000000001208, -3.741295971395164515E-16 ) ) ;
#85161=CARTESIAN_POINT ( 'NONE',  ( 46.20833333333332149, -3.974999999999999201, -6.884901960086287964 ) ) ;
#85206=CARTESIAN_POINT ( 'NONE',  ( 66.84959685856479439, 6.109999999999997655, 1.637169565754163836 ) ) ;
#85223=CARTESIAN_POINT ( 'NONE',  ( 53.49999999999999289, 0.000000000000000000, -7.950000000000000178 ) ) ;
#85234=CARTESIAN_POINT ( 'NONE',  ( 92.39169371712955581, 2.130196079827421762, 7.950000000000001066 ) ) ;
#85240=CARTESIAN_POINT ( 'NONE',  ( 150.3000000000000114, 0.000000000000000000, 0.000000000000000000 ) ) ;
#85242=LINE ( 'NONE', #16398, #97664 ) ;
#85246=CARTESIAN_POINT ( 'NONE',  ( 71.02126352523144703, -4.472830434245839371, -4.472830434245840259 ) ) ;
#85261=CARTESIAN_POINT ( 'NONE',  ( 60.35416666666666430, -2.130196079827425759, -7.950000000000000178 ) ) ;
#85264=CARTESIAN_POINT ( 'NONE',  ( 77.00043019189811844, -3.055000000000002380, 5.291415217122920289 ) ) ;
#85288=CARTESIAN_POINT ( 'NONE',  ( 52.57919371712956291, 3.975000000000002753, -6.884901960086283523 ) ) ;
#85308=CARTESIAN_POINT ( 'NONE',  ( 26.99999999999998579, -5.652181678087170091, -4.022882452454510371 ) ) ;
#85321=CARTESIAN_POINT ( 'NONE',  ( 61.54209685856476852, 5.291415217122923842, -3.054999999999996163 ) ) ;
#85328=CARTESIAN_POINT ( 'NONE',  ( 102.0837635252314328, -6.110000000000001208, -3.741295971395164515E-16 ) ) ;
#85336=CARTESIAN_POINT ( 'NONE',  ( 78.39169371712955581, 2.130196079827421762, 7.950000000000000178 ) ) ;
#85360=ADVANCED_FACE ( 'NONE', ( #10798 ), #111570, .F. ) ;
#85376=CARTESIAN_POINT ( 'NONE',  ( 34.41709685856476852, 3.054999999999998828, 5.291415217122922066 ) ) ;
#85394=CARTESIAN_POINT ( 'NONE',  ( 119.3708603837962272, 6.884901960086289741, -3.974999999999993427 ) ) ;
#85397=DIRECTION ( 'NONE',  ( 1.000000000000000000, 0.000000000000000000, 0.000000000000000000 ) ) ;
#85422=CARTESIAN_POINT ( 'NONE',  ( 39.93750000000000000, 5.819803920172574863, -5.819803920172573086 ) ) ;
#85431=CARTESIAN_POINT ( 'NONE',  ( 103.6879301918981042, 6.110000000000002984, -1.637169565754156730 ) ) ;
#85438=CARTESIAN_POINT ( 'NONE',  ( 76.25000000000000000, -9.735942053221458872E-16, 7.950000000000000178 ) ) ;
#85441=CARTESIAN_POINT ( 'NONE',  ( 92.80793019189812298, -6.109999999999998543, 1.637169565754158063 ) ) ;
#85446=CARTESIAN_POINT ( 'NONE',  ( 127.2293817626157164, 0.000000000000000000, -7.030000000000000249 ) ) ;
#85473=FACE_OUTER_BOUND ( 'NONE', #80310, .T. ) ;
#85525=CARTESIAN_POINT ( 'NONE',  ( 94.12043019189810877, 3.055000000000002380, -5.291415217122917625 ) ) ;
#85547=CYLINDRICAL_SURFACE ( 'NONE', #70017, 7.950000000000000178 ) ;
#85571=CARTESIAN_POINT ( 'NONE',  ( 47.08333333333332149, 6.884901960086290629, -3.974999999999994316 ) ) ;
#85583=CARTESIAN_POINT ( 'NONE',  ( 109.9375000000000000, 5.819803920172573974, -5.819803920172572198 ) ) ;
#85595=CARTESIAN_POINT ( 'NONE',  ( 100.0420968585647756, 5.291415217122923842, -3.054999999999996163 ) ) ;
#85602=CARTESIAN_POINT ( 'NONE',  ( 0.000000000000000000, 9.735942053221458872E-16, -7.950000000000000178 ) ) ;
#85603=CARTESIAN_POINT ( 'NONE',  ( 32.60002705046289151, 5.819803920172570422, 5.819803920172574863 ) ) ;
#85608=CARTESIAN_POINT ( 'NONE',  ( 126.7295968585647614, -6.110000000000000320, -1.637169565754161393 ) ) ;
#85617=CARTESIAN_POINT ( 'NONE',  ( 124.1620968585647944, -5.291415217122919401, 3.054999999999997939 ) ) ;
#85631=CARTESIAN_POINT ( 'NONE',  ( 46.66709685856476852, -3.055000000000000160, -5.291415217122921177 ) ) ;
#85639=CARTESIAN_POINT ( 'NONE',  ( 41.32876352523144448, 0.000000000000000000, -6.109999999999998543 ) ) ;
#85670=CARTESIAN_POINT ( 'NONE',  ( 59.70376352523145158, 6.109999999999998543, 1.122388791418548911E-15 ) ) ;
#85703=CARTESIAN_POINT ( 'NONE',  ( 124.1620968585647944, -5.291415217122919401, 3.054999999999998384 ) ) ;
#85740=EDGE_CURVE ( 'NONE', #5013, #78734, #93210, .T. ) ;
#85751=CARTESIAN_POINT ( 'NONE',  ( 126.8603669610315308, -5.004565729002734109, -4.329968208352205750 ) ) ;
#85752=CARTESIAN_POINT ( 'NONE',  ( 41.62043019189810877, 3.055000000000002380, -5.291415217122917625 ) ) ;
#85782=CARTESIAN_POINT ( 'NONE',  ( 57.24586038379622721, 3.974999999999996980, 6.884901960086287964 ) ) ;
#85788=CARTESIAN_POINT ( 'NONE',  ( 50.58333333333332860, 6.884901960086290629, -3.974999999999994316 ) ) ;
#85795=CARTESIAN_POINT ( 'NONE',  ( 47.83376352523143993, 6.110000000000001208, 1.122388791418549305E-15 ) ) ;
#85809=CARTESIAN_POINT ( 'NONE',  ( 86.33376352523144703, 6.110000000000001208, 1.122388791418549305E-15 ) ) ;
#85817=CARTESIAN_POINT ( 'NONE',  ( 71.37043019189812298, -3.055000000000001492, 5.291415217122917625 ) ) ;
#85829=ORIENTED_EDGE ( 'NONE', *, *, #21569, .T. ) ;
#85832=CARTESIAN_POINT ( 'NONE',  ( 64.43749999999998579, 5.819803920172574863, -5.819803920172573086 ) ) ;
#85845=CARTESIAN_POINT ( 'NONE',  ( 51.41252705046289861, -7.949999999999998401, -4.867971026610728450E-16 ) ) ;
#85850=ORIENTED_EDGE ( 'NONE', *, *, #33969, .F. ) ;
#85851=CARTESIAN_POINT ( 'NONE',  ( 88.57876352523145158, -7.482591942790325086E-16, 6.109999999999998543 ) ) ;
#85878=CARTESIAN_POINT ( 'NONE',  ( 35.43793019189810423, -6.110000000000001208, 1.637169565754158951 ) ) ;
#85880=ORIENTED_EDGE ( 'NONE', *, *, #18443, .F. ) ;
#85908=ADVANCED_FACE ( 'NONE', ( #123001 ), #12781, .F. ) ;
#85933=CARTESIAN_POINT ( 'NONE',  ( 61.01626352523143737, -4.472830434245839371, 4.472830434245839371 ) ) ;
#85941=DIRECTION ( 'NONE',  ( -1.000000000000000000, -0.000000000000000000, -0.000000000000000000 ) ) ;
#85964=CARTESIAN_POINT ( 'NONE',  ( 84.66252705046289861, 7.949999999999998401, 1.460391307983218338E-15 ) ) ;
#85978=CARTESIAN_POINT ( 'NONE',  ( 77.87543019189810423, -5.291415217122920289, -3.055000000000001492 ) ) ;
#85979=CIRCLE ( 'NONE', #127698, 8.000000000000001776 ) ;
#85984=PLANE ( 'NONE',  #74324 ) ;
#85993=CARTESIAN_POINT ( 'NONE',  ( 77.41666666666665719, -6.884901960086287076, -3.975000000000000977 ) ) ;
#85997=CARTESIAN_POINT ( 'NONE',  ( 73.06293019189811844, 1.637169565754157174, 6.110000000000002984 ) ) ;
#86000=DIRECTION ( 'NONE',  ( -1.000000000000000000, -0.000000000000000000, -0.000000000000000000 ) ) ;
#86004=CARTESIAN_POINT ( 'NONE',  ( 59.28752705046289151, 0.000000000000000000, -7.949999999999998401 ) ) ;
#86045=CARTESIAN_POINT ( 'NONE',  ( 57.68336038379621300, -2.130196079827426203, 7.949999999999996625 ) ) ;
#86056=CARTESIAN_POINT ( 'NONE',  ( 49.99999999999998579, 0.000000000000000000, -7.950000000000000178 ) ) ;
#86063=CARTESIAN_POINT ( 'NONE',  ( 61.97959685856476852, 6.109999999999999432, 1.637169565754164280 ) ) ;
#86069=CARTESIAN_POINT ( 'NONE',  ( 99.75043019189810423, 3.055000000000002824, -5.291415217122919401 ) ) ;
#86088=CARTESIAN_POINT ( 'NONE',  ( 120.6620968585647802, -5.291415217122919401, 3.054999999999997939 ) ) ;
#86101=CARTESIAN_POINT ( 'NONE',  ( 38.77083333333331439, -7.949999999999998401, -2.130196079827426203 ) ) ;
#86113=DIRECTION ( 'NONE',  ( 0.000000000000000000, 0.000000000000000000, -1.000000000000000000 ) ) ;
#86114=CARTESIAN_POINT ( 'NONE',  ( 29.16709685856476497, -3.055000000000000160, -5.291415217122921177 ) ) ;
#86134=CARTESIAN_POINT ( 'NONE',  ( 92.97502705046289861, -5.819803920172573086, 5.819803920172573086 ) ) ;
#86136=CARTESIAN_POINT ( 'NONE',  ( 109.7458603837962272, 3.974999999999996980, 6.884901960086287964 ) ) ;
#86156=CARTESIAN_POINT ( 'NONE',  ( 92.24586038379622721, 3.974999999999996980, 6.884901960086287964 ) ) ;
#86164=CARTESIAN_POINT ( 'NONE',  ( 92.58333333333332860, 6.884901960086290629, -3.974999999999994316 ) ) ;
#86177=CARTESIAN_POINT ( 'NONE',  ( 99.89626352523141861, 4.472830434245840259, -4.472830434245839371 ) ) ;
#86185=CARTESIAN_POINT ( 'NONE',  ( 96.89126352523143737, -4.472830434245839371, -4.472830434245839371 ) ) ;
#86191=CARTESIAN_POINT ( 'NONE',  ( 115.7708333333333428, -7.949999999999998401, -2.130196079827426203 ) ) ;
#86228=B_SPLINE_CURVE_WITH_KNOTS ( 'NONE', 3,
 ( #143224, #77292, #43924, #33776 ),
 .UNSPECIFIED., .F., .F.,
 ( 4, 4 ),
 ( 0.0007011148265759370056, 0.001001374831347506215 ),
 .UNSPECIFIED. ) ;
#86238=EDGE_LOOP ( 'NONE', ( #134377, #96137, #25012, #114071 ) ) ;
#86245=CARTESIAN_POINT ( 'NONE',  ( 28.49543019189811233, 5.291415217122916737, 3.055000000000001936 ) ) ;
#86282=CARTESIAN_POINT ( 'NONE',  ( 88.14126352523143737, 4.472830434245837594, 4.472830434245841147 ) ) ;
#86283=CARTESIAN_POINT ( 'NONE',  ( 9.745384874281414866, -8.447767063957357436, -4.346192636695838551 ) ) ;
#86299=AXIS2_PLACEMENT_3D ( 'NONE', #121551, #22226, #66488 ) ;
#86315=CARTESIAN_POINT ( 'NONE',  ( 27.24999999999999645, -9.735942053221458872E-16, 7.950000000000000178 ) ) ;
#86333=CARTESIAN_POINT ( 'NONE',  ( 111.5416666666666572, -3.975000000000002753, 6.884901960086286188 ) ) ;
#86346=CARTESIAN_POINT ( 'NONE',  ( 99.89626352523141861, 4.472830434245840259, -4.472830434245839371 ) ) ;
#86360=CARTESIAN_POINT ( 'NONE',  ( 26.37499999999999645, 7.950000000000000178, 1.460391307983218535E-15 ) ) ;
#86371=CARTESIAN_POINT ( 'NONE',  ( 126.7870968585647944, 3.054999999999997495, 5.291415217122919401 ) ) ;
#86382=CARTESIAN_POINT ( 'NONE',  ( 49.43793019189809002, -6.110000000000001208, 1.637169565754158951 ) ) ;
#86389=CARTESIAN_POINT ( 'NONE',  ( 36.22459685856478728, -1.637169565754160949, 6.109999999999997655 ) ) ;
#86421=CARTESIAN_POINT ( 'NONE',  ( 55.76626352523145158, 4.472830434245838482, -4.472830434245837594 ) ) ;
#86428=DIRECTION ( 'NONE',  ( -1.000000000000000000, -0.000000000000000000, -0.000000000000000000 ) ) ;
#86432=DIRECTION ( 'NONE',  ( -1.000000000000000000, -0.000000000000000000, -0.000000000000000000 ) ) ;
#86455=CARTESIAN_POINT ( 'NONE',  ( 121.3912635252314374, -4.472830434245839371, -4.472830434245839371 ) ) ;
#86462=CARTESIAN_POINT ( 'NONE',  ( 68.03752705046289861, -9.735942053221456900E-16, 7.949999999999998401 ) ) ;
#86469=LINE ( 'NONE', #142284, #60415 ) ;
#86494=CARTESIAN_POINT ( 'NONE',  ( 34.32876352523143737, 0.000000000000000000, -6.109999999999999432 ) ) ;
#86523=CARTESIAN_POINT ( 'NONE',  ( 57.10002705046289861, 5.819803920172570422, 5.819803920172574863 ) ) ;
#86528=CARTESIAN_POINT ( 'NONE',  ( 57.58333333333333570, 6.884901960086290629, -3.974999999999994316 ) ) ;
#86537=CARTESIAN_POINT ( 'NONE',  ( 46.37543019189810423, -5.291415217122920289, -3.055000000000001492 ) ) ;
#86551=CARTESIAN_POINT ( 'NONE',  ( 85.60459685856477563, 1.637169565754164946, -6.109999999999999432 ) ) ;
#86561=CARTESIAN_POINT ( 'NONE',  ( 71.95376352523145158, -6.109999999999998543, -3.741295971395162543E-16 ) ) ;
#86594=CARTESIAN_POINT ( 'NONE',  ( 80.99543019189810877, 5.291415217122916737, 3.055000000000001936 ) ) ;
#86613=CARTESIAN_POINT ( 'NONE',  ( 123.7458603837962272, 3.974999999999996980, 6.884901960086287964 ) ) ;
#86621=CARTESIAN_POINT ( 'NONE',  ( 37.33376352523143282, 6.110000000000001208, 1.122388791418549305E-15 ) ) ;
#86624=( BOUNDED_CURVE ( )  B_SPLINE_CURVE ( 2, ( #130167, #33722, #110510, #67046, #1036, #125535, #47987, #64911, #56909, #77236, #101080, #92155, #111231 ),
 .UNSPECIFIED., .F., .T. ) 
 B_SPLINE_CURVE_WITH_KNOTS ( ( 3, 2, 2, 2, 2, 2, 3 ),
 ( 0.1333333333333333037, 0.1361111111111110716, 0.1388888888888888673, 0.1416666666666666630, 0.1444444444444444309, 0.1472222222222222265, 0.1499999999999999944 ),
 .UNSPECIFIED. ) 
 CURVE ( )  GEOMETRIC_REPRESENTATION_ITEM ( )  RATIONAL_B_SPLINE_CURVE ( ( 1.000000000000000444, 0.9659258262890679791, 1.000000000000000000, 0.9659258262890683122, 1.000000000000000000, 0.9659258262890683122, 1.000000000000000000, 0.9659258262890683122, 1.000000000000000000, 0.9659258262890683122, 1.000000000000000000, 0.9659258262890683122, 1.000000000000000000 ) ) 
 REPRESENTATION_ITEM ( '' )  );
#86635=LINE ( 'NONE', #32236, #141977 ) ;
#86642=CARTESIAN_POINT ( 'NONE',  ( 108.4333603837962272, 2.130196079827431532, -7.949999999999996625 ) ) ;
#86667=CARTESIAN_POINT ( 'NONE',  ( 53.20833333333332860, -3.974999999999999201, -6.884901960086287964 ) ) ;
#86669=CARTESIAN_POINT ( 'NONE',  ( 67.87043019189812298, -3.055000000000001936, 5.291415217122918513 ) ) ;
#86696=CARTESIAN_POINT ( 'NONE',  ( 82.76669371712952739, -7.949999999999999289, 2.130196079827424427 ) ) ;
#86701=ADVANCED_FACE ( 'NONE', ( #124011 ), #2922, .T. ) ;
#86711=CARTESIAN_POINT ( 'NONE',  ( 74.08376352523143282, -6.110000000000001208, -3.741295971395164515E-16 ) ) ;
#86723=CARTESIAN_POINT ( 'NONE',  ( 76.39583333333332860, -2.130196079827427091, 7.949999999999998401 ) ) ;
#86728=CARTESIAN_POINT ( 'NONE',  ( 67.22959685856476142, -6.110000000000000320, -1.637169565754161393 ) ) ;
#86732=CYLINDRICAL_SURFACE ( 'NONE', #19813, 7.950000000000000178 ) ;
#86760=CARTESIAN_POINT ( 'NONE',  ( 114.8287635252314516, 0.000000000000000000, -6.109999999999998543 ) ) ;
#86769=CARTESIAN_POINT ( 'NONE',  ( 68.62086038379622721, -6.884901960086286188, 3.974999999999997424 ) ) ;
#86784=CARTESIAN_POINT ( 'NONE',  ( 62.41709685856476852, 3.054999999999998828, 5.291415217122922066 ) ) ;
#86791=CARTESIAN_POINT ( 'NONE',  ( 100.7712635252314328, 4.472830434245838482, 4.472830434245842035 ) ) ;
#86799=CARTESIAN_POINT ( 'NONE',  ( 90.25000000000000000, -9.735942053221458872E-16, 7.950000000000000178 ) ) ;
#86806=CARTESIAN_POINT ( 'NONE',  ( 117.5995968585647944, -6.109999999999997655, -1.637169565754160283 ) ) ;
#86813=ORIENTED_EDGE ( 'NONE', *, *, #60548, .F. ) ;
#86833=CARTESIAN_POINT ( 'NONE',  ( 26.54209685856477563, 5.291415217122923842, -3.054999999999996163 ) ) ;
#86856=CARTESIAN_POINT ( 'NONE',  ( 110.7666937171295558, -7.949999999999999289, 2.130196079827424427 ) ) ;
#86878=( BOUNDED_CURVE ( )  B_SPLINE_CURVE ( 2, ( #59331, #103483, #115057, #4122, #120797, #73729, #140415, #54860, #86769, #120051, #96868, #143268, #99034 ),
 .UNSPECIFIED., .F., .T. ) 
 B_SPLINE_CURVE_WITH_KNOTS ( ( 3, 2, 2, 2, 2, 2, 3 ),
 ( 0.5666666666666666519, 0.5694444444444444198, 0.5722222222222221877, 0.5749999999999999556, 0.5777777777777777235, 0.5805555555555556024, 0.5833333333333333703 ),
 .UNSPECIFIED. ) 
 CURVE ( )  GEOMETRIC_REPRESENTATION_ITEM ( )  RATIONAL_B_SPLINE_CURVE ( ( 1.000000000000000000, 0.9659258262890683122, 1.000000000000000000, 0.9659258262890683122, 1.000000000000000000, 0.9659258262890683122, 1.000000000000000000, 0.9659258262890683122, 1.000000000000000000, 0.9659258262890683122, 1.000000000000000000, 0.9659258262890683122, 1.000000000000000000 ) ) 
 REPRESENTATION_ITEM ( '' )  );
#86894=CARTESIAN_POINT ( 'NONE',  ( 91.43793019189810423, -6.110000000000001208, 1.637169565754158951 ) ) ;
#86901=CARTESIAN_POINT ( 'NONE',  ( 49.70833333333332860, -3.974999999999999201, -6.884901960086287964 ) ) ;
#86904=CARTESIAN_POINT ( 'NONE',  ( 96.01626352523143737, -4.472830434245839371, 4.472830434245839371 ) ) ;
#86919=CARTESIAN_POINT ( 'NONE',  ( 0.000000000000000000, 0.000000000000000000, 0.000000000000000000 ) ) ;
#86976=CARTESIAN_POINT ( 'NONE',  ( 95.43293019189809456, 1.637169565754156730, 6.110000000000001208 ) ) ;
#87012=EDGE_CURVE ( 'NONE', #125049, #61826, #15679, .T. ) ;
#87034=CARTESIAN_POINT ( 'NONE',  ( 98.12500000000000000, -7.950000000000000178, -4.867971026610729436E-16 ) ) ;
#87055=CARTESIAN_POINT ( 'NONE',  ( 32.30836038379622721, 7.949999999999997513, 2.130196079827431088 ) ) ;
#87060=CARTESIAN_POINT ( 'NONE',  ( 118.4170968585647756, 3.054999999999998828, 5.291415217122922066 ) ) ;
#87071=CARTESIAN_POINT ( 'NONE',  ( 118.9120968585647802, 5.291415217122921177, -3.054999999999994831 ) ) ;
#87081=CARTESIAN_POINT ( 'NONE',  ( 43.45876352523143993, 0.000000000000000000, -6.110000000000001208 ) ) ;
#87089=CARTESIAN_POINT ( 'NONE',  ( 41.03709685856478728, -3.054999999999998828, -5.291415217122919401 ) ) ;
#87118=CARTESIAN_POINT ( 'NONE',  ( 60.57876352523145158, -7.482591942790325086E-16, 6.109999999999998543 ) ) ;
#87152=CARTESIAN_POINT ( 'NONE',  ( 118.4745968585647802, 1.637169565754164280, -6.109999999999997655 ) ) ;
#87171=VERTEX_POINT ( 'NONE', #63990 ) ;
#87184=CARTESIAN_POINT ( 'NONE',  ( 0.000000000000000000, 9.735942053221458872E-16, -7.950000000000000178 ) ) ;
#87194=CARTESIAN_POINT ( 'NONE',  ( 40.45376352523144448, -6.109999999999999432, -3.741295971395163529E-16 ) ) ;
#87213=CARTESIAN_POINT ( 'NONE',  ( 127.0212635252314328, -4.472830434245839371, -4.472830434245840259 ) ) ;
#87219=ADVANCED_FACE ( 'NONE', ( #57412 ), #116593, .T. ) ;
#87224=CARTESIAN_POINT ( 'NONE',  ( 58.12086038379622721, -6.884901960086286188, 3.974999999999997424 ) ) ;
#87229=CARTESIAN_POINT ( 'NONE',  ( 55.97916666666666430, -7.950000000000001066, 2.130196079827424427 ) ) ;
#87237=CARTESIAN_POINT ( 'NONE',  ( 49.29209685856476852, -5.291415217122921177, 3.054999999999999272 ) ) ;
#87244=CARTESIAN_POINT ( 'NONE',  ( 81.89169371712957002, 2.130196079827421762, 7.950000000000000178 ) ) ;
#87252=CARTESIAN_POINT ( 'NONE',  ( 79.33376352523144703, 6.110000000000001208, 1.122388791418549305E-15 ) ) ;
#87254=CARTESIAN_POINT ( 'NONE',  ( 113.5375270504628986, -9.735942053221456900E-16, 7.949999999999998401 ) ) ;
#87261=CARTESIAN_POINT ( 'NONE',  ( 71.22459685856478018, -1.637169565754160949, 6.109999999999997655 ) ) ;
#87294=CARTESIAN_POINT ( 'NONE',  ( 83.91209685856479439, 5.291415217122921177, -3.054999999999994831 ) ) ;
#87300=DIRECTION ( 'NONE',  ( -1.000000000000000000, -0.000000000000000000, -0.000000000000000000 ) ) ;
#87319=CARTESIAN_POINT ( 'NONE',  ( 37.77126352523143993, 4.472830434245838482, 4.472830434245842035 ) ) ;
#87344=ORIENTED_EDGE ( 'NONE', *, *, #15620, .T. ) ;
#87360=EDGE_CURVE ( 'NONE', #128126, #46491, #31403, .T. ) ;
#87376=CARTESIAN_POINT ( 'NONE',  ( 68.30793019189809456, -6.109999999999999432, 1.637169565754158507 ) ) ;
#87404=CARTESIAN_POINT ( 'NONE',  ( 84.95419371712955581, 6.884901960086283523, 3.975000000000002753 ) ) ;
#87410=CARTESIAN_POINT ( 'NONE',  ( 87.04166666666665719, -3.975000000000002753, 6.884901960086286188 ) ) ;
#87416=ORIENTED_EDGE ( 'NONE', *, *, #44311, .F. ) ;
#87418=CARTESIAN_POINT ( 'NONE',  ( 74.22959685856476142, -6.110000000000000320, -1.637169565754161393 ) ) ;
#87434=CARTESIAN_POINT ( 'NONE',  ( 76.68749999999998579, -5.819803920172573974, 5.819803920172573086 ) ) ;
#87442=CARTESIAN_POINT ( 'NONE',  ( 66.06293019189810423, 1.637169565754157174, 6.110000000000002984 ) ) ;
#87466=( BOUNDED_CURVE ( )  B_SPLINE_CURVE ( 2, ( #7699, #85261, #41783, #118612, #41061, #138965, #28051, #104887, #130231, #5554, #39663, #38924, #50516 ),
 .UNSPECIFIED., .F., .T. ) 
 B_SPLINE_CURVE_WITH_KNOTS ( ( 3, 2, 2, 2, 2, 2, 3 ),
 ( 0.6333333333333333037, 0.6361111111111110716, 0.6388888888888888395, 0.6416666666666667185, 0.6444444444444444864, 0.6472222222222222543, 0.6500000000000000222 ),
 .UNSPECIFIED. ) 
 CURVE ( )  GEOMETRIC_REPRESENTATION_ITEM ( )  RATIONAL_B_SPLINE_CURVE ( ( 1.000000000000000000, 0.9659258262890683122, 1.000000000000000000, 0.9659258262890683122, 1.000000000000000000, 0.9659258262890683122, 1.000000000000000000, 0.9659258262890683122, 1.000000000000000000, 0.9659258262890683122, 1.000000000000000000, 0.9659258262890683122, 1.000000000000000000 ) ) 
 REPRESENTATION_ITEM ( '' )  );
#87470=CARTESIAN_POINT ( 'NONE',  ( 111.7662635252314516, 4.472830434245838482, -4.472830434245837594 ) ) ;
#87491=CARTESIAN_POINT ( 'NONE',  ( 65.91709685856477563, 3.054999999999998828, 5.291415217122922066 ) ) ;
#87496=CARTESIAN_POINT ( 'NONE',  ( 96.10459685856477563, 1.637169565754164946, -6.109999999999999432 ) ) ;
#87511=CARTESIAN_POINT ( 'NONE',  ( 120.8079301918980946, -6.109999999999998543, 1.637169565754158507 ) ) ;
#87525=CARTESIAN_POINT ( 'NONE',  ( 38.04166666666665719, -3.975000000000002753, 6.884901960086286188 ) ) ;
#87537=CARTESIAN_POINT ( 'NONE',  ( 31.50043019189810423, -3.055000000000002380, 5.291415217122920289 ) ) ;
#87559=CARTESIAN_POINT ( 'NONE',  ( 111.7875270504628986, 0.000000000000000000, -7.949999999999998401 ) ) ;
#87583=CARTESIAN_POINT ( 'NONE',  ( 92.72916666666665719, 7.950000000000001954, -2.130196079827421762 ) ) ;
#87591=CARTESIAN_POINT ( 'NONE',  ( 70.41666666666665719, -6.884901960086287076, -3.975000000000000977 ) ) ;
#87599=CARTESIAN_POINT ( 'NONE',  ( 90.12543019189811844, 5.291415217122919401, 3.055000000000002824 ) ) ;
#87603=CARTESIAN_POINT ( 'NONE',  ( 84.22502705046288440, 5.819803920172573974, -5.819803920172573086 ) ) ;
#87607=CARTESIAN_POINT ( 'NONE',  ( 86.68293019189813720, -1.637169565754158951, -6.109999999999998543 ) ) ;
#87661=CARTESIAN_POINT ( 'NONE',  ( 123.6670968585647756, -3.055000000000000160, -5.291415217122921177 ) ) ;
#87690=CARTESIAN_POINT ( 'NONE',  ( 92.37043019189810877, -3.055000000000001936, 5.291415217122918513 ) ) ;
#87691=CARTESIAN_POINT ( 'NONE',  ( 8.118486091812719962, -8.713627631029451592, -3.788380083765350737 ) ) ;
#87696=DIRECTION ( 'NONE',  ( -1.000000000000000000, -0.000000000000000000, -0.000000000000000000 ) ) ;
#87720=EDGE_LOOP ( 'NONE', ( #141736, #81935, #102697, #60280 ) ) ;
#87741=CARTESIAN_POINT ( 'NONE',  ( 110.3750000000000000, 7.950000000000000178, 1.460391307983218535E-15 ) ) ;
#87745=CARTESIAN_POINT ( 'NONE',  ( 96.95833333333334281, 3.974999999999997424, 6.884901960086288852 ) ) ;
#87773=CARTESIAN_POINT ( 'NONE',  ( 122.2087635252314328, -7.482591942790329030E-16, 6.110000000000001208 ) ) ;
#87776=DIRECTION ( 'NONE',  ( -1.000000000000000000, -0.000000000000000000, -0.000000000000000000 ) ) ;
#87781=CARTESIAN_POINT ( 'NONE',  ( 112.0579301918981372, 6.110000000000000320, -1.637169565754156064 ) ) ;
#87784=CARTESIAN_POINT ( 'NONE',  ( 70.66252705046288440, 7.949999999999998401, 1.460391307983218338E-15 ) ) ;
#87788=CARTESIAN_POINT ( 'NONE',  ( 41.12543019189809712, 5.291415217122919401, 3.055000000000002824 ) ) ;
#87793=CARTESIAN_POINT ( 'NONE',  ( 42.78709685856478728, 3.054999999999997495, 5.291415217122919401 ) ) ;
#87801=CARTESIAN_POINT ( 'NONE',  ( 150.3000000000000114, 0.000000000000000000, 4.749999999999997335 ) ) ;
#87825=CARTESIAN_POINT ( 'NONE',  ( 49.20376352523145158, 6.109999999999998543, 1.122388791418548911E-15 ) ) ;
#87827=( BOUNDED_CURVE ( )  B_SPLINE_CURVE ( 2, ( #47716, #135422, #89742, #136816, #125233, #123108, #57867, #23784, #35407, #103457, #102780, #25920, #79649 ),
 .UNSPECIFIED., .F., .T. ) 
 B_SPLINE_CURVE_WITH_KNOTS ( ( 3, 2, 2, 2, 2, 2, 3 ),
 ( 0.2166666666666667296, 0.2194444444444444697, 0.2222222222222222376, 0.2250000000000000056, 0.2277777777777777457, 0.2305555555555555414, 0.2333333333333332815 ),
 .UNSPECIFIED. ) 
 CURVE ( )  GEOMETRIC_REPRESENTATION_ITEM ( )  RATIONAL_B_SPLINE_CURVE ( ( 0.9999999999999993339, 0.9659258262890689783, 1.000000000000000000, 0.9659258262890683122, 1.000000000000000000, 0.9659258262890683122, 1.000000000000000000, 0.9659258262890683122, 1.000000000000000000, 0.9659258262890683122, 1.000000000000000000, 0.9659258262890689783, 0.9999999999999993339 ) ) 
 REPRESENTATION_ITEM ( '' )  );
#87864=CARTESIAN_POINT ( 'NONE',  ( 116.4329301918981088, 1.637169565754156730, 6.110000000000001208 ) ) ;
#87901=CARTESIAN_POINT ( 'NONE',  ( 42.05793019189811588, 6.110000000000001208, -1.637169565754156286 ) ) ;
#87920=CARTESIAN_POINT ( 'NONE',  ( 123.2295968585647756, -6.110000000000000320, -1.637169565754161393 ) ) ;
#87928=CARTESIAN_POINT ( 'NONE',  ( 60.74586038379622721, 3.974999999999996980, 6.884901960086287964 ) ) ;
#87935=CARTESIAN_POINT ( 'NONE',  ( 48.54166666666666430, -3.975000000000002753, 6.884901960086286188 ) ) ;
#87945=CARTESIAN_POINT ( 'NONE',  ( 48.56293019189809712, 1.637169565754157174, 6.110000000000002984 ) ) ;
#87953=CARTESIAN_POINT ( 'NONE',  ( 80.28752705046289861, 0.000000000000000000, -7.949999999999998401 ) ) ;
#87962=CARTESIAN_POINT ( 'NONE',  ( 80.64626352523141861, -4.472830434245840259, 4.472830434245838482 ) ) ;
#87971=CARTESIAN_POINT ( 'NONE',  ( 66.99543019189812298, 5.291415217122916737, 3.055000000000001936 ) ) ;
#88002=CARTESIAN_POINT ( 'NONE',  ( 79.09959685856478018, -6.109999999999997655, -1.637169565754160283 ) ) ;
#88054=ORIENTED_EDGE ( 'NONE', *, *, #57686, .F. ) ;
#88088=CARTESIAN_POINT ( 'NONE',  ( 63.05793019189810877, 6.110000000000001208, -1.637169565754156286 ) ) ;
#88089=CYLINDRICAL_SURFACE ( 'NONE', #27928, 7.950000000000000178 ) ;
#88113=CARTESIAN_POINT ( 'NONE',  ( 85.82919371712955581, -3.975000000000001865, 6.884901960086284411 ) ) ;
#88117=CARTESIAN_POINT ( 'NONE',  ( 70.12500000000000000, -7.950000000000000178, -4.867971026610729436E-16 ) ) ;
#88122=( BOUNDED_CURVE ( )  B_SPLINE_CURVE ( 2, ( #47566, #92419, #2553, #90293, #91724, #14158, #91048, #56995, #101169, #134547, #112765, #25755, #1129 ),
 .UNSPECIFIED., .F., .F. ) 
 B_SPLINE_CURVE_WITH_KNOTS ( ( 3, 2, 2, 2, 2, 2, 3 ),
 ( 0.8666666666666666963, 0.8694444444444444642, 0.8722222222222222321, 0.8750000000000000000, 0.8777777777777777679, 0.8805555555555555358, 0.8833333333333333037 ),
 .UNSPECIFIED. ) 
 CURVE ( )  GEOMETRIC_REPRESENTATION_ITEM ( )  RATIONAL_B_SPLINE_CURVE ( ( 1.000000000000000000, 0.9659258262890683122, 1.000000000000000000, 0.9659258262890683122, 1.000000000000000000, 0.9659258262890683122, 1.000000000000000000, 0.9659258262890683122, 1.000000000000000000, 0.9659258262890683122, 1.000000000000000000, 0.9659258262890683122, 1.000000000000000000 ) ) 
 REPRESENTATION_ITEM ( '' )  );
#88129=CARTESIAN_POINT ( 'NONE',  ( 78.45876352523144703, 0.000000000000000000, -6.110000000000001208 ) ) ;
#88145=ORIENTED_EDGE ( 'NONE', *, *, #68538, .F. ) ;
#88153=CARTESIAN_POINT ( 'NONE',  ( 65.18793019189811844, 6.110000000000002984, -1.637169565754156730 ) ) ;
#88175=CARTESIAN_POINT ( 'NONE',  ( 128.4511022459138019, -4.648522628062369932, -4.648522628062369932 ) ) ;
#88183=CARTESIAN_POINT ( 'NONE',  ( 113.0787635252314516, -7.482591942790325086E-16, 6.109999999999998543 ) ) ;
#88196=CARTESIAN_POINT ( 'NONE',  ( 37.16666666666666430, 6.884901960086285300, 3.975000000000003642 ) ) ;
#88199=CARTESIAN_POINT ( 'NONE',  ( 58.26669371712954870, -7.949999999999998401, 2.130196079827423983 ) ) ;
#88211=CARTESIAN_POINT ( 'NONE',  ( 68.10459685856474721, 1.637169565754164946, -6.109999999999999432 ) ) ;
#88217=CARTESIAN_POINT ( 'NONE',  ( 98.58376352523144703, -6.110000000000001208, -3.741295971395164515E-16 ) ) ;
#88230=CARTESIAN_POINT ( 'NONE',  ( 122.2662635252314374, 4.472830434245838482, -4.472830434245837594 ) ) ;
#88245=AXIS2_PLACEMENT_3D ( 'NONE', #39526, #85142, #72901 ) ;
#88254=UNCERTAINTY_MEASURE_WITH_UNIT (LENGTH_MEASURE( 1.000000000000000082E-05 ), #118250, 'distance_accuracy_value', 'NONE');
#88272=CARTESIAN_POINT ( 'NONE',  ( 42.12499999999999289, -7.950000000000000178, -4.867971026610729436E-16 ) ) ;
#88284=CARTESIAN_POINT ( 'NONE',  ( 113.6833603837962272, -2.130196079827426203, 7.949999999999997513 ) ) ;
#88285=DIRECTION ( 'NONE',  ( -1.000000000000000000, -0.000000000000000000, -0.000000000000000000 ) ) ;
#88329=CARTESIAN_POINT ( 'NONE',  ( 88.95876352523143282, 0.000000000000000000, -6.110000000000001208 ) ) ;
#88332=CARTESIAN_POINT ( 'NONE',  ( 85.39169371712957002, 2.130196079827421762, 7.950000000000000178 ) ) ;
#88337=CARTESIAN_POINT ( 'NONE',  ( 49.99999999999998579, 0.000000000000000000, -7.950000000000000178 ) ) ;
#88340=CARTESIAN_POINT ( 'NONE',  ( 83.18293019189810877, -1.637169565754158951, -6.109999999999998543 ) ) ;
#88377=CARTESIAN_POINT ( 'NONE',  ( 118.3958333333333286, -2.130196079827369804, 7.950000000000031264 ) ) ;
#88427=CARTESIAN_POINT ( 'NONE',  ( 86.82876352523145158, 0.000000000000000000, -6.109999999999999432 ) ) ;
#88428=CARTESIAN_POINT ( 'NONE',  ( 6.094872978304351818, -9.434020220044425642, 1.153095517109193668 ) ) ;
#88475=CARTESIAN_POINT ( 'NONE',  ( 104.1041666666666714, 2.130196079827422206, 7.950000000000001954 ) ) ;
#88489=EDGE_CURVE ( 'NONE', #75827, #2756, #85153, .T. ) ;
#88503=CARTESIAN_POINT ( 'NONE',  ( 121.0420968585647756, 5.291415217122923842, -3.054999999999996163 ) ) ;
#88513=CARTESIAN_POINT ( 'NONE',  ( 110.3079301918980946, -6.109999999999998543, 1.637169565754158063 ) ) ;
#88522=CARTESIAN_POINT ( 'NONE',  ( 39.37543019189809712, -5.291415217122920289, -3.055000000000001492 ) ) ;
#88528=CARTESIAN_POINT ( 'NONE',  ( 26.59959685856477307, -6.109999999999997655, -1.637169565754160283 ) ) ;
#88539=EDGE_CURVE ( 'NONE', #82607, #25494, #33532, .T. ) ;
#88556=DIRECTION ( 'NONE',  ( -1.000000000000000000, -0.000000000000000000, -0.000000000000000000 ) ) ;
#88565=CARTESIAN_POINT ( 'NONE',  ( 46.28709685856477307, 3.054999999999997495, 5.291415217122919401 ) ) ;
#88601=CARTESIAN_POINT ( 'NONE',  ( 113.9537635252314516, -6.109999999999999432, -3.741295971395163529E-16 ) ) ;
#88612=DIRECTION ( 'NONE',  ( 0.000000000000000000, 0.000000000000000000, -1.000000000000000000 ) ) ;
#88638=CARTESIAN_POINT ( 'NONE',  ( 27.76626352523143737, 4.472830434245839371, -4.472830434245839371 ) ) ;
#88644=FACE_OUTER_BOUND ( 'NONE', #39520, .T. ) ;
#88657=CARTESIAN_POINT ( 'NONE',  ( 126.5837635252314612, -6.110000000000001208, -3.741295971395164515E-16 ) ) ;
#88667=CARTESIAN_POINT ( 'NONE',  ( 50.82919371712955581, -3.975000000000001865, 6.884901960086284411 ) ) ;
#88674=CARTESIAN_POINT ( 'NONE',  ( 41.10416666666666430, 2.130196079827422206, 7.950000000000001954 ) ) ;
#88682=CARTESIAN_POINT ( 'NONE',  ( 40.10459685856476142, 1.637169565754164946, -6.109999999999999432 ) ) ;
#88696=CARTESIAN_POINT ( 'NONE',  ( 78.02126352523144703, -4.472830434245838482, -4.472830434245840259 ) ) ;
#88706=CARTESIAN_POINT ( 'NONE',  ( 87.57919371712957002, 3.975000000000002753, -6.884901960086283523 ) ) ;
#88707=CARTESIAN_POINT ( 'NONE',  ( 57.95376352523144448, -6.109999999999998543, -3.741295971395162543E-16 ) ) ;
#88733=CARTESIAN_POINT ( 'NONE',  ( 51.70419371712956291, -6.884901960086285300, -3.975000000000000089 ) ) ;
#88738=CARTESIAN_POINT ( 'NONE',  ( 79.53709685856478018, -3.054999999999998828, -5.291415217122919401 ) ) ;
#88741=EDGE_CURVE ( 'NONE', #108642, #1460, #84351, .T. ) ;
#88815=CARTESIAN_POINT ( 'NONE',  ( 55.76626352523145869, 4.472830434245839371, -4.472830434245839371 ) ) ;
#88818=CARTESIAN_POINT ( 'NONE',  ( 32.16252705046289151, 7.949999999999998401, 1.460391307983218338E-15 ) ) ;
#88841=CARTESIAN_POINT ( 'NONE',  ( 86.12086038379622721, -6.884901960086286188, 3.974999999999997424 ) ) ;
#88848=CARTESIAN_POINT ( 'NONE',  ( 73.91666666666665719, -6.884901960086287076, -3.975000000000000977 ) ) ;
#88855=AXIS2_PLACEMENT_3D ( 'NONE', #36134, #12912, #57188 ) ;
#88860=CARTESIAN_POINT ( 'NONE',  ( 69.12543019189809002, 5.291415217122919401, 3.055000000000002824 ) ) ;
#88878=CARTESIAN_POINT ( 'NONE',  ( 65.04209685856477563, 5.291415217122923842, -3.054999999999996163 ) ) ;
#88905=CARTESIAN_POINT ( 'NONE',  ( 60.50000000000000000, 0.000000000000000000, -7.950000000000000178 ) ) ;
#88913=CARTESIAN_POINT ( 'NONE',  ( 98.78709685856479439, 3.054999999999997495, 5.291415217122919401 ) ) ;
#88939=CARTESIAN_POINT ( 'NONE',  ( 58.18793019189810423, 6.110000000000002984, -1.637169565754156730 ) ) ;
#88943=CARTESIAN_POINT ( 'NONE',  ( 89.83376352523143282, 6.110000000000001208, 1.122388791418549305E-15 ) ) ;
#88960=CARTESIAN_POINT ( 'NONE',  ( 119.4954301918981230, 5.291415217122916737, 3.055000000000001936 ) ) ;
#88993=CYLINDRICAL_SURFACE ( 'NONE', #20940, 7.950000000000000178 ) ;
#89006=CARTESIAN_POINT ( 'NONE',  ( 110.9125270504628986, -7.949999999999998401, -4.867971026610728450E-16 ) ) ;
#89027=CARTESIAN_POINT ( 'NONE',  ( 103.6879301918981042, 6.110000000000002984, -1.637169565754156730 ) ) ;
#89050=CARTESIAN_POINT ( 'NONE',  ( 94.06293019189809002, 1.637169565754157174, 6.110000000000002984 ) ) ;
#89059=CARTESIAN_POINT ( 'NONE',  ( 82.16209685856479439, -5.291415217122919401, 3.054999999999997939 ) ) ;
#89085=DIRECTION ( 'NONE',  ( 0.000000000000000000, 1.000000000000000000, 6.123233995736750012E-17 ) ) ;
#89102=VECTOR ( 'NONE', #84903, 1000.000000000000000 ) ;
#89107=CARTESIAN_POINT ( 'NONE',  ( 119.7295968585647756, -6.110000000000000320, -1.637169565754161393 ) ) ;
#89113=EDGE_CURVE ( 'NONE', #37814, #26730, #99100, .T. ) ;
#89132=ORIENTED_EDGE ( 'NONE', *, *, #88741, .T. ) ;
#89136=CARTESIAN_POINT ( 'NONE',  ( 84.93293019189812298, 1.637169565754156730, 6.110000000000001208 ) ) ;
#89137=CARTESIAN_POINT ( 'NONE',  ( 6.856969496093653582, -9.116755745626452523, 2.682239519146091045 ) ) ;
#89161=( BOUNDED_CURVE ( )  B_SPLINE_CURVE ( 2, ( #142278, #140134, #108158, #29202, #54556, #107478, #119063, #18296, #8141, #73443, #85012, #8823, #42964 ),
 .UNSPECIFIED., .F., .T. ) 
 B_SPLINE_CURVE_WITH_KNOTS ( ( 3, 2, 2, 2, 2, 2, 3 ),
 ( 0.5000000000000000000, 0.5027777777777777679, 0.5055555555555555358, 0.5083333333333333037, 0.5111111111111110716, 0.5138888888888888395, 0.5166666666666667185 ),
 .UNSPECIFIED. ) 
 CURVE ( )  GEOMETRIC_REPRESENTATION_ITEM ( )  RATIONAL_B_SPLINE_CURVE ( ( 1.000000000000000000, 0.9659258262890683122, 1.000000000000000000, 0.9659258262890683122, 1.000000000000000000, 0.9659258262890683122, 1.000000000000000000, 0.9659258262890683122, 1.000000000000000000, 0.9659258262890683122, 1.000000000000000000, 0.9659258262890683122, 1.000000000000000000 ) ) 
 REPRESENTATION_ITEM ( '' )  );
#89182=CARTESIAN_POINT ( 'NONE',  ( 98.56250000000000000, -5.819803920172572198, -5.819803920172573086 ) ) ;
#89200=CARTESIAN_POINT ( 'NONE',  ( 27.00000000000001421, 3.441786896390103934, 7.166352137582786774 ) ) ;
#89203=CARTESIAN_POINT ( 'NONE',  ( 85.68336038379622721, -2.130196079827426203, 7.949999999999996625 ) ) ;
#89211=CARTESIAN_POINT ( 'NONE',  ( 123.2295968585647756, -6.110000000000000320, -1.637169565754161393 ) ) ;
#89218=CARTESIAN_POINT ( 'NONE',  ( 118.4745968585647802, 1.637169565754164058, -6.109999999999996767 ) ) ;
#89226=CARTESIAN_POINT ( 'NONE',  ( 35.87543019189811133, -5.291415217122920289, -3.055000000000001492 ) ) ;
#89227=ORIENTED_EDGE ( 'NONE', *, *, #128931, .F. ) ;
#89232=CARTESIAN_POINT ( 'NONE',  ( 34.18293019189809456, -1.637169565754158951, -6.109999999999998543 ) ) ;
#89259=CARTESIAN_POINT ( 'NONE',  ( 43.37043019189810877, -3.055000000000001492, 5.291415217122917625 ) ) ;
#89294=CARTESIAN_POINT ( 'NONE',  ( 114.3912635252314232, -4.472830434245839371, -4.472830434245839371 ) ) ;
#89307=CARTESIAN_POINT ( 'NONE',  ( 120.0000000000000000, 0.000000000000000000, -7.950000000000000178 ) ) ;
#89332=CARTESIAN_POINT ( 'NONE',  ( 126.0872339960914275, -6.972148538754269431, 2.385612954137347419 ) ) ;
#89333=CARTESIAN_POINT ( 'NONE',  ( 30.53709685856477307, -3.054999999999999272, -5.291415217122919401 ) ) ;
#89350=CARTESIAN_POINT ( 'NONE',  ( 126.0004301918981042, -3.055000000000002380, 5.291415217122920289 ) ) ;
#89360=CARTESIAN_POINT ( 'NONE',  ( 45.43336038379622011, 2.130196079827431532, -7.949999999999997513 ) ) ;
#89366=CARTESIAN_POINT ( 'NONE',  ( 42.56249999999998579, -5.819803920172572198, -5.819803920172573086 ) ) ;
#89376=CARTESIAN_POINT ( 'NONE',  ( 36.31293019189809002, -1.637169565754159617, -6.110000000000001208 ) ) ;
#89382=CARTESIAN_POINT ( 'NONE',  ( 0.000000000000000000, 0.000000000000000000, 7.950000000000000178 ) ) ;
#89399=CARTESIAN_POINT ( 'NONE',  ( 53.72459685856478018, -1.637169565754160949, 6.109999999999997655 ) ) ;
#89417=DIRECTION ( 'NONE',  ( 0.000000000000000000, 0.000000000000000000, 1.000000000000000000 ) ) ;
#89424=CARTESIAN_POINT ( 'NONE',  ( 71.51626352523145158, -4.472830434245838482, 4.472830434245838482 ) ) ;
#89447=CARTESIAN_POINT ( 'NONE',  ( 28.87543019189810067, -5.291415217122920289, -3.055000000000001492 ) ) ;
#89449=CARTESIAN_POINT ( 'NONE',  ( 44.75000000000000000, -9.735942053221458872E-16, 7.950000000000000178 ) ) ;
#89503=CARTESIAN_POINT ( 'NONE',  ( 54.16209685856478018, -5.291415217122919401, 3.054999999999998384 ) ) ;
#89528=CARTESIAN_POINT ( 'NONE',  ( 78.82919371712957002, -3.975000000000001865, 6.884901960086284411 ) ) ;
#89532=CARTESIAN_POINT ( 'NONE',  ( 78.14583333333332860, 2.130196079827431976, -7.949999999999999289 ) ) ;
#89541=CARTESIAN_POINT ( 'NONE',  ( 64.75043019189810423, 3.055000000000002824, -5.291415217122919401 ) ) ;
#89561=CARTESIAN_POINT ( 'NONE',  ( 54.54209685856477563, 5.291415217122923842, -3.054999999999996163 ) ) ;
#89591=CARTESIAN_POINT ( 'NONE',  ( 107.0995968585648086, -6.109999999999997655, -1.637169565754160283 ) ) ;
#89610=CARTESIAN_POINT ( 'NONE',  ( 86.75000000000000000, -9.735942053221458872E-16, 7.950000000000000178 ) ) ;
#89618=CARTESIAN_POINT ( 'NONE',  ( 51.91709685856476852, 3.054999999999998828, 5.291415217122922066 ) ) ;
#89626=CARTESIAN_POINT ( 'NONE',  ( 90.12543019189811844, 5.291415217122919401, 3.055000000000002824 ) ) ;
#89667=CARTESIAN_POINT ( 'NONE',  ( 8.377306452199936970, 8.650827907999497413, -3.927822742214815754 ) ) ;
#89685=CARTESIAN_POINT ( 'NONE',  ( 69.25000000000000000, -9.735942053221458872E-16, 7.950000000000000178 ) ) ;
#89694=CARTESIAN_POINT ( 'NONE',  ( 102.7458603837962272, 3.974999999999996980, 6.884901960086287964 ) ) ;
#89704=FACE_OUTER_BOUND ( 'NONE', #134602, .T. ) ;
#89710=CARTESIAN_POINT ( 'NONE',  ( 92.60459685856478984, 1.637169565754164946, -6.109999999999999432 ) ) ;
#89724=FACE_OUTER_BOUND ( 'NONE', #76309, .T. ) ;
#89734=CARTESIAN_POINT ( 'NONE',  ( 96.68793019189811844, 6.110000000000002984, -1.637169565754156730 ) ) ;
#89742=CARTESIAN_POINT ( 'NONE',  ( 103.9583333333333286, 3.974999999999997424, 6.884901960086288852 ) ) ;
#89745=CARTESIAN_POINT ( 'NONE',  ( 84.64126352523145158, 4.472830434245836706, 4.472830434245840259 ) ) ;
#89792=CARTESIAN_POINT ( 'NONE',  ( 121.4795968585647614, 6.109999999999999432, 1.637169565754164280 ) ) ;
#89810=CARTESIAN_POINT ( 'NONE',  ( 108.2875270504628986, 0.000000000000000000, -7.949999999999998401 ) ) ;
#89822=CARTESIAN_POINT ( 'NONE',  ( 84.49543019189812298, 5.291415217122917625, 3.055000000000002380 ) ) ;
#89840=DIRECTION ( 'NONE',  ( 0.000000000000000000, 0.000000000000000000, 1.000000000000000000 ) ) ;
#89856=CARTESIAN_POINT ( 'NONE',  ( 48.20419371712955581, -6.884901960086285300, -3.975000000000000089 ) ) ;
#89865=CARTESIAN_POINT ( 'NONE',  ( 109.5000000000000000, 0.000000000000000000, -7.950000000000000178 ) ) ;
#89869=CARTESIAN_POINT ( 'NONE',  ( 104.6875000000000000, -5.819803920172573086, 5.819803920172572198 ) ) ;
#89900=CARTESIAN_POINT ( 'NONE',  ( 124.9795968585647756, 6.109999999999999432, 1.637169565754164280 ) ) ;
#89902=CARTESIAN_POINT ( 'NONE',  ( 100.3124999999999858, 5.819803920172571310, 5.819803920172576639 ) ) ;
#89909=CARTESIAN_POINT ( 'NONE',  ( 118.6204301918981230, 3.055000000000001936, -5.291415217122916737 ) ) ;
#89917=CARTESIAN_POINT ( 'NONE',  ( 35.00043019189810423, -3.055000000000002380, 5.291415217122920289 ) ) ;
#89922=CARTESIAN_POINT ( 'NONE',  ( 29.95376352523145158, -6.109999999999998543, -3.741295971395162543E-16 ) ) ;
#89924=CARTESIAN_POINT ( 'NONE',  ( 0.000000000000000000, 9.735942053221458872E-16, -7.950000000000000178 ) ) ;
#89948=CARTESIAN_POINT ( 'NONE',  ( 44.39126352523143737, -4.472830434245838482, -4.472830434245838482 ) ) ;
#89958=ADVANCED_FACE ( 'NONE', ( #139498 ), #62625, .T. ) ;
#89963=EDGE_LOOP ( 'NONE', ( #11724, #763, #66064, #30162 ) ) ;
#89987=CARTESIAN_POINT ( 'NONE',  ( 107.2454301918981088, -5.291415217122919401, -3.055000000000000604 ) ) ;
#90048=CARTESIAN_POINT ( 'NONE',  ( 125.7087635252314470, -7.482591942790329030E-16, 6.110000000000001208 ) ) ;
#90059=CARTESIAN_POINT ( 'NONE',  ( 45.28752705046289151, 0.000000000000000000, -7.949999999999998401 ) ) ;
#90062=VERTEX_POINT ( 'NONE', #109679 ) ;
#90064=CARTESIAN_POINT ( 'NONE',  ( 46.93749999999999289, 5.819803920172573974, -5.819803920172572198 ) ) ;
#90072=CARTESIAN_POINT ( 'NONE',  ( 36.89626352523143993, 4.472830434245840259, -4.472830434245839371 ) ) ;
#90090=CARTESIAN_POINT ( 'NONE',  ( 39.89169371712955581, 2.130196079827421762, 7.950000000000000178 ) ) ;
#90101=CARTESIAN_POINT ( 'NONE',  ( 59.41209685856478728, 5.291415217122921177, -3.054999999999994831 ) ) ;
#90133=CARTESIAN_POINT ( 'NONE',  ( 74.87043019189812298, -3.055000000000001492, 5.291415217122917625 ) ) ;
#90158=CARTESIAN_POINT ( 'NONE',  ( 30.62543019189810423, 5.291415217122919401, 3.055000000000002824 ) ) ;
#90185=VECTOR ( 'NONE', #51434, 1000.000000000000000 ) ;
#90212=CARTESIAN_POINT ( 'NONE',  ( 52.26626352523145158, 4.472830434245839371, -4.472830434245839371 ) ) ;
#90236=CARTESIAN_POINT ( 'NONE',  ( 75.76669371712954160, -7.949999999999999289, 2.130196079827424427 ) ) ;
#90240=CARTESIAN_POINT ( 'NONE',  ( 74.93750000000000000, 5.819803920172573974, -5.819803920172572198 ) ) ;
#90249=CARTESIAN_POINT ( 'NONE',  ( 67.81293019189807580, -1.637169565754159617, -6.110000000000001208 ) ) ;
#90266=CARTESIAN_POINT ( 'NONE',  ( 54.25043019189811133, 3.055000000000002824, -5.291415217122919401 ) ) ;
#90293=CARTESIAN_POINT ( 'NONE',  ( 37.85002705046288440, -5.819803920172573086, -5.819803920172573086 ) ) ;
#90299=ORIENTED_EDGE ( 'NONE', *, *, #68959, .T. ) ;
#90300=CARTESIAN_POINT ( 'NONE',  ( 103.8912635252314516, -4.472830434245838482, -4.472830434245838482 ) ) ;
#90313=ORIENTED_EDGE ( 'NONE', *, *, #4816, .T. ) ;
#90318=CARTESIAN_POINT ( 'NONE',  ( 68.37499999999998579, 7.950000000000000178, 1.460391307983218535E-15 ) ) ;
#90332=CARTESIAN_POINT ( 'NONE',  ( 50.45876352523143282, 0.000000000000000000, -6.110000000000001208 ) ) ;
#90337=CARTESIAN_POINT ( 'NONE',  ( 88.22959685856474721, -6.110000000000000320, -1.637169565754161393 ) ) ;
#90357=CIRCLE ( 'NONE', #62644, 4.749999999999997335 ) ;
#90364=DIRECTION ( 'NONE',  ( -1.000000000000000000, -0.000000000000000000, -0.000000000000000000 ) ) ;
#90409=CARTESIAN_POINT ( 'NONE',  ( 99.53752705046289861, -9.735942053221456900E-16, 7.949999999999998401 ) ) ;
#90427=CARTESIAN_POINT ( 'NONE',  ( 97.70876352523144703, -7.482591942790329030E-16, 6.110000000000001208 ) ) ;
#90428=VECTOR ( 'NONE', #5878, 1000.000000000000000 ) ;
#90447=CARTESIAN_POINT ( 'NONE',  ( 101.4333603837962414, 2.130196079827431532, -7.949999999999996625 ) ) ;
#90448=CARTESIAN_POINT ( 'NONE',  ( 0.000000000000000000, 0.000000000000000000, 0.000000000000000000 ) ) ;
#90456=CARTESIAN_POINT ( 'NONE',  ( 84.43793019189811844, -6.110000000000001208, 1.637169565754158951 ) ) ;
#90470=CARTESIAN_POINT ( 'NONE',  ( 83.91209685856479439, 5.291415217122921177, -3.054999999999994831 ) ) ;
#90516=CARTESIAN_POINT ( 'NONE',  ( 116.1625270504628986, 7.949999999999998401, 1.460391307983218338E-15 ) ) ;
#90526=CARTESIAN_POINT ( 'NONE',  ( 121.3337635252314328, 6.110000000000001208, 1.122388791418549305E-15 ) ) ;
#90562=CARTESIAN_POINT ( 'NONE',  ( 80.12043019189810877, 3.055000000000002380, -5.291415217122917625 ) ) ;
#90564=CARTESIAN_POINT ( 'NONE',  ( 98.51669371712957002, 7.950000000000000178, -2.130196079827421318 ) ) ;
#90576=CARTESIAN_POINT ( 'NONE',  ( 80.28752705046289861, 0.000000000000000000, -7.949999999999998401 ) ) ;
#90577=ADVANCED_FACE ( 'NONE', ( #42529 ), #86732, .T. ) ;
#90610=CARTESIAN_POINT ( 'NONE',  ( 95.79166666666665719, 3.975000000000003642, -6.884901960086285300 ) ) ;
#90622=CARTESIAN_POINT ( 'NONE',  ( 14.55557268365555679, 9.434219313260308937, -1.151903651517597549 ) ) ;
#90645=CARTESIAN_POINT ( 'NONE',  ( 108.5004301918981184, -3.055000000000002380, 5.291415217122920289 ) ) ;
#90650=CARTESIAN_POINT ( 'NONE',  ( 99.87499999999998579, 7.950000000000000178, 1.460391307983218535E-15 ) ) ;
#90658=CARTESIAN_POINT ( 'NONE',  ( 109.5787635252314516, -7.482591942790325086E-16, 6.109999999999998543 ) ) ;
#90673=CARTESIAN_POINT ( 'NONE',  ( 32.72459685856478728, -1.637169565754160949, 6.109999999999997655 ) ) ;
#90703=CARTESIAN_POINT ( 'NONE',  ( 48.76626352523144448, 4.472830434245838482, -4.472830434245837594 ) ) ;
#90742=CARTESIAN_POINT ( 'NONE',  ( 111.1829301918981230, -1.637169565754159173, -6.109999999999999432 ) ) ;
#90754=CARTESIAN_POINT ( 'NONE',  ( 120.4374999999999858, 5.819803920172574863, -5.819803920172573086 ) ) ;
#90789=CARTESIAN_POINT ( 'NONE',  ( 121.8958333333333144, -2.130196079827427091, 7.949999999999999289 ) ) ;
#90801=CARTESIAN_POINT ( 'NONE',  ( 124.1045968585647756, 1.637169565754164946, -6.109999999999999432 ) ) ;
#90804=CARTESIAN_POINT ( 'NONE',  ( 104.7875270504628986, 0.000000000000000000, -7.949999999999998401 ) ) ;
#90810=CARTESIAN_POINT ( 'NONE',  ( 51.41252705046289861, -7.949999999999998401, -4.867971026610728450E-16 ) ) ;
#90816=CARTESIAN_POINT ( 'NONE',  ( 48.68749999999998579, -5.819803920172573086, 5.819803920172572198 ) ) ;
#90830=CARTESIAN_POINT ( 'NONE',  ( 42.43793019189809712, -6.110000000000001208, 1.637169565754158951 ) ) ;
#90837=MECHANICAL_DESIGN_GEOMETRIC_PRESENTATION_REPRESENTATION('',(#137067),#44486);
#90852=CARTESIAN_POINT ( 'NONE',  ( 31.28752705046289151, 0.000000000000000000, -7.949999999999998401 ) ) ;
#90853=CARTESIAN_POINT ( 'NONE',  ( 58.68293019189811588, -1.637169565754158951, -6.109999999999998543 ) ) ;
#90874=CYLINDRICAL_SURFACE ( 'NONE', #96584, 4.749999999999997335 ) ;
#90876=ORIENTED_EDGE ( 'NONE', *, *, #107812, .T. ) ;
#90879=( BOUNDED_SURFACE ( )  B_SPLINE_SURFACE ( 1, 2, ( 
 ( #111055, #98766, #32104, #56032, #120493, #143004, #132875, #43693, #132150, #121241, #21931, #11024, #33565, #121940, #45163, #126255, #92902, #26931, #3711, #35716, #38534, #46605, #79938, #16021, #92173, #48697, #101633, #125555, #26232, #24786, #58912, #71180, #124109, #60307, #102382, #90789, #114642, #15310, #113216, #81347, #103753, #69035, #48004, #13886, #14635, #3031, #4397, #104485, #103077, #47323, #58189, #91495, #27637, #36392, #49444, #82757, #135708, #115326, #136402, #5146, #137136, #37839, #71902, #82073, #70496, #93630, #137861, #69768, #80622, #126944, #116075, #37092, #124822, #25491, #59593, #113943, #16771, #2284, #135021, #130552, #51565, #83473, #141407, #127694, #84210, #94327, #128405, #105206, #7297, #31237, #105892, #96436, #42122, #107347, #41371, #6557, #116796, #52946, #75453, #28380, #72637, #50838, #119624, #63174, #140680, #61051, #86333, #117485, #19625, #17480, #29771, #50130, #5865, #139301, #140006, #138562, #30521, #85583, #62441, #106600, #8015, #39258, #61733, #52255, #74754, #129814, #118935, #95759, #18159, #29083, #95026, #39993, #73317, #63871, #108031, #40682, #84887, #129096, #74019, #8695, #118198, #18907, #97148, #1416, #45700, #111643, #21042, #133407, #134117, #65310, #43524, #120326, #97912, #89869, #76902, #77606, #55126, #88475, #11573, #121075, #34096, #66022, #78305, #9426, #99303, #121777, #122492, #23167, #108743, #55854, #22455, #100763, #10859, #131980, #100059, #34804, #56598, #109495, #143547, #66711, #21775, #44262, #79048, #110887, #132718, #67447, #32665, #12313, #20319, #33408, #710, #64562, #45006, #53709, #142150, #89182, #110188, #42834, #87034, #131249, #31937, #76162, #10170, #54433, #98609, #142840, #87745, #2114, #115164, #58010, #46427, #92722, #136958, #70326, #90610, #113776, #102205, #47159, #4225, #124650, #58744, #69592, #59435, #24620, #37667, #15836, #4965, #91340, #134852, #13718, #113045, #81169, #25327, #60133, #104299, #23927, #14466, #136232, #112358, #38365, #35548, #92016, #123958, #36920, #57291, #48520, #81906, #125376, #102913, #3554, #126097, #49267, #26762, #68875, #80459, #71012, #47851, #13016, #93456, #68186, #137691, #123253, #2859, #135549, #36233, #103592, #26063, #114474, #15152, #101463, #79778, #106421, #54097, #50657, #87410, #65696, #17988, #73839, #98283, #128928, #71718, #10524, #7109, #139114, #142508, #131626, #18715, #29601, #117317, #82579, #39070, #118013, #43195, #109859, #105034, #76544, #17311, #5699, #32315, #120722, #64948, #49965, #73153, #61572, #6382, #109139, #84040, #62265, #28914, #9825, #127506, #21432, #54786, #98964, #94850, #94148, #116629, #72459, #40515, #128236, #143203, #126772, #27456, #51389, #95583, #115882, #16583, #138384, #139844, #83297, #84717, #60873, #28202, #105722, #39818, #89532, #133763, #101838, #35904, #13374, #133073, #1072, #46805, #112020, #33060, #68528, #132366, #113412, #124304, #33756, #56245, #11958, #123627, #100425, #46062, #55499, #67830, #90240, #24971, #69228, #135216, #44654, #57650, #14096, #88848, #67082, #359, #121441, #58392, #45357, #101114, #78667, #12672, #35184, #34443, #2490, #122876, #90988, #77271, #23562, #1761, #80121, #102575, #22119, #79430, #134484, #43904, #56942, #24281, #112713, #88117, #66374, #77961, #110545, #11219, #99683, #122144, #22808, #111266, #116281, #27843, #4594, #48902, #5354, #116986, #91672, #93816, #16976, #72108, #138042, #137337, #59781, #114820, #114137, #72836, #125752, #38729, #6052, #26427, #69973, #14822, #81547, #48177, #37300, #82950, #16217, #61246, #127146, #105392, #93106, #80821, #83688, #135896, #125013, #50324, #38032, #94511, #3221, #27122, #71365, #59094, #103946, #138764, #25695, #39460, #3901, #36573, #60507, #104686, #103253, #126430, #49637, #92364, #82255, #136595, #115522, #70675, #127896, #28578, #17657, #15501, #61930, #47512, #32129, #40872, #53915, #43021, #106812, #75647, #52440, #9636, #97352, #42318, #76358, #141615, #130016, #86528, #108946, #74214, #73507, #20508, #53148, #96628, #140186, #29972, #30726, #117671, #87229, #74952, #131453, #120527, #140866, #128590, #21251, #29265, #129282, #139505, #118406, #6753, #41565, #106081, #7501, #130754, #51036, #8881, #31425, #51760, #18356, #98108, #95233, #62632, #95950, #85077, #40189, #108219, #119819, #84397, #19107, #63372, #64765, #107539, #119129, #8198, #142338, #85788, #19811, #64052, #121971, #123461, #68371, #1605, #12508, #100250, #65512, #21959, #100947, #35014, #90816, #87935, #57479, #172, #132178, #79255, #24119, #56789, #32873, #56061, #44467, #132907, #90064, #66906, #905, #11778, #45890, #110378, #112547, #101662, #135053, #33589, #77095, #99499, #55325, #23381, #111087, #2319, #46638, #109690, #45189, #78498, #54613, #124136, #121272, #34277, #66204, #122696, #143034, #134314, #13206, #67652, #89366, #133601, #35747, #79965, #10358, #11051, #22642, #98795, #111846, #43719, #88674, #77790, #94355, #105238, #14665, #37122, #136428, #104516, #81378, #26957, #36421, #125585, #80651, #69798, #58944, #5174, #37868, #49473, #16044, #93663, #70526, #102412, #5890, #113243, #3060, #82791, #15338, #115356, #24820, #48729, #92931, #91521, #26262, #137887, #47355, #126974, #25522, #13921, #82102, #126280, #124847, #4420, #71209, #135736, #114668, #113973, #59625, #103103, #60335, #27665, #103781, #3740, #48030, #92200, #138593, #137166, #116101, #50159, #38560, #71932, #16800, #61079, #39285, #83508, #58221, #69063, #129846, #64592, #118229, #95786, #63894, #9456, #20346, #29108, #107374, #30548, #40709, #18938, #53736, #74782, #8043, #97173, #140033, #130582, #108766, #63203, #118961, #141439, #19653, #116826, #97937, #52278, #84913, #42149, #31265, #108057, #8724, #96464, #127724, #84237, #52978, #86360, #142175, #6588, #119649, #62464, #50865, #75478, #42864, #28404, #95061, #140708, #106635, #51590 ),
 ( #17506, #72668, #139331, #41401, #128435, #85608, #61761, #105925, #40021, #73347, #29805, #74044, #117515, #18189, #7327, #129127, #44291, #89900, #11598, #76191, #111672, #31964, #13041, #23954, #76927, #99332, #55154, #23194, #17026, #89211, #79078, #21071, #101492, #134145, #112387, #34835, #87773, #56625, #57317, #132004, #110211, #43551, #65339, #2144, #88503, #734, #121801, #55884, #78332, #132740, #100791, #33433, #1442, #120351, #22479, #45030, #66741, #77633, #67479, #32696, #45727, #123281, #87060, #10885, #109520, #121101, #21800, #133431, #110915, #68211, #131275, #10195, #100083, #34119, #54459, #98635, #142864, #122525, #66048, #12338, #123982, #115185, #104325, #4253, #92037, #136261, #4992, #38390, #15866, #135577, #3580, #49294, #114501, #35575, #71037, #134879, #115907, #126798, #36256, #58771, #14490, #126119, #102938, #48550, #82605, #24644, #60898, #93481, #71749, #137716, #47184, #60159, #16615, #91366, #69619, #2888, #68899, #105062, #47873, #103614, #81196, #15179, #37693, #36947, #27484, #125404, #46454, #79806, #26092, #92746, #90645, #113077, #13747, #81933, #136987, #58037, #70351, #59456, #26791, #102237, #80485, #124679, #25357, #113804, #62293, #40540, #75312, #96292, #29625, #118786, #117340, #8553, #130405, #84742, #140535, #19480, #52111, #138414, #119480, #73868, #106452, #63727, #52799, #85431, #41226, #128955, #5723, #105746, #129659, #107886, #31093, #28228, #141249, #84064, #72487, #96998, #41962, #30357, #116650, #139865, #128261, #73179, #74601, #7133, #94878, #83325, #139140, #20170, #28937, #86177, #64413, #6406, #49990, #95609, #94172, #39100, #127531, #17337, #61595, #118041, #50688, #39844, #18012, #51415, #18746, #63021, #107197, #7872, #32515, #132570, #120182, #89734, #77468, #45560, #34655, #99153, #131109, #133957, #31793, #131824, #142003, #76750, #9272, #54987, #78889, #10029, #567, #123096, #11422, #89050, #54292, #20893, #100627, #23776, #76008, #65159, #98471, #108589, #110738, #44861, #53548, #97757, #21633, #67286, #109348, #121632, #42694, #86894, #43386, #44107, #142695, #78164, #133267, #110045, #10719, #55703, #87599, #120931, #99899, #122340, #33950, #23016, #143400, #65887, #88329, #33265, #22302, #66571, #111485, #12166, #56452, #1275, #36094, #123818, #112915, #102045, #4089, #81022, #92567, #59291, #136807, #113619, #1961, #4810, #12867, #46272, #125947, #58599, #15014, #68042, #91870, #136092, #134700, #25181, #37519, #90456, #26623, #68725, #57151, #125224, #25911, #79640, #47708, #70179, #35396, #14312, #24476, #124507, #13575, #114342, #70865, #69435, #36772, #103448, #102770, #3414, #137538, #48372, #81754, #115018, #80322, #15695, #49113, #59978, #104146, #93305, #38223, #101325, #82442, #126625, #112220, #57858, #2714, #47011, #91200, #135415, #27315, #127355, #62843, #140374, #52645, #49833, #19314, #105582, #94003, #41066, #85264, #117867, #138244, #17854, #6243, #94704, #51958, #28779, #106282, #117173, #107024, #72319, #129487, #63571, #96832, #138968, #38927, #61440, #17178, #128783, #73024, #107732, #8392, #71567, #62121, #40382, #16427, #85997, #83149, #139701, #28054, #84586, #104891, #96138, #30180, #29462, #6958, #51245, #74428, #141076, #118615, #116485, #128098, #41787, #95438, #60722, #115725, #5559, #50521, #39667, #83893, #73697, #18563, #7703, #98314, #132399, #122173, #64254, #1103, #133103, #11988, #77992, #130955, #99718, #100452, #31626, #9855, #86728, #108417, #56275, #43225, #43932, #21461, #54814, #121469, #87442, #390, #32341, #44685, #119319, #65725, #88153, #88878, #33784, #75157, #22145, #33090, #67111, #120755, #142538, #66404, #45384, #22842, #75850, #141827, #109888, #77301, #9096, #76578, #97575, #131657, #120014, #110575, #111299, #10553, #20726, #53363, #64984, #130235, #109172, #30923, #20006, #54124, #42525, #98998, #143234, #11256, #55526, #61780, #82816, #113441, #27689, #94371, #57685, #56971, #5908, #38581, #80150, #123653, #13403, #14129, #101144, #72690, #58421, #28428, #17523, #124335, #112046, #116847, #12700, #112742, #122912, #101864, #133792, #35931, #105945, #134516, #126997, #6605, #137907, #71955, #35217, #1791, #83533, #89561, #46092, #90266, #79459, #34477, #93681, #116126, #78694, #23591, #2524, #50183, #24309, #104540, #67861, #68555, #46832, #25004, #91021, #61104, #16828, #135242, #69259, #105258, #5205, #49496, #138618, #39310, #127744, #42168, #41422, #107395, #18963, #18211, #120371, #29824, #86382, #53757, #73368, #62484, #63229, #106662, #95806, #84934, #130608, #63911, #75496, #31286, #119667, #96484, #128455, #131295, #139355, #29126, #108790, #85631, #141463, #50890, #74809, #118986, #117534, #8061, #20366, #7351, #9480, #51614, #40044, #108076, #8744, #64611, #19672, #97959, #52297, #142194, #31979, #129869, #42886, #87081, #97198, #84257, #21094, #52999, #140726, #76206, #65358, #109539, #95085, #30571, #140052, #40730, #129147, #74066, #118253, #87788, #111689, #10907, #132024, #34136, #78349, #100099, #32718, #33449, #110225, #55174, #133449, #88522, #77650, #132760, #45047, #121121, #122543, #12356, #100807, #99348, #76947, #66065, #17, #11618, #121819, #56642, #1459, #10214, #22494, #55901, #142884, #54474, #21818, #753, #44310, #89226, #66761, #23218, #67498, #45744, #110934, #89917, #98655, #43569, #109284, #85376, #96938, #142633, #64357, #128887, #20832, #84684, #65829, #76689, #129592, #8495, #107830, #75947, #52746, #141945, #131764, #73807, #10655, #43326, #21571, #87537, #140477, #9962, #109990, #41166, #19418, #96234, #117977, #54922, #141185, #53486, #31032, #108529, #131045, #41901, #54232, #86114, #98416, #29569, #75258, #97691, #32448, #120860, #18682, #31729, #42635, #139807, #130342, #119418, #120121, #40486, #62957, #30297, #20112, #86833, #9204, #65093, #107134, #7811, #52059, #74540, #118724, #63671, #16453, #126656 ) ),
 .UNSPECIFIED., .F., .F., .F. ) 
 B_SPLINE_SURFACE_WITH_KNOTS ( ( 2, 2 ),
 ( 3, 2, 2, 2, 2, 2, 2, 2, 2, 2, 2, 2, 2, 2, 2, 2, 2, 2, 2, 2, 2, 2, 2, 2, 2, 2, 2, 2, 2, 2, 2, 2, 2, 2, 2, 2, 2, 2, 2, 2, 2, 2, 2, 2, 2, 2, 2, 2, 2, 2, 2, 2, 2, 2, 2, 2, 2, 2, 2, 2, 2, 2, 2, 2, 2, 2, 2, 2, 2, 2, 2, 2, 2, 2, 2, 2, 2, 2, 2, 2, 2, 2, 2, 2, 2, 2, 2, 2, 2, 2, 2, 2, 2, 2, 2, 2, 2, 2, 2, 2, 2, 2, 2, 2, 2, 2, 2, 2, 2, 2, 2, 2, 2, 2, 2, 2, 2, 2, 2, 2, 2, 2, 2, 2, 2, 2, 2, 2, 2, 2, 2, 2, 2, 2, 2, 2, 2, 2, 2, 2, 2, 2, 2, 2, 2, 2, 2, 2, 2, 2, 2, 2, 2, 2, 2, 2, 2, 2, 2, 2, 2, 2, 2, 2, 2, 2, 2, 2, 2, 2, 2, 2, 2, 2, 2, 2, 2, 2, 2, 2, 2, 2, 2, 2, 2, 2, 2, 2, 2, 2, 2, 2, 2, 2, 2, 2, 2, 2, 2, 2, 2, 2, 2, 2, 2, 2, 2, 2, 2, 2, 2, 2, 2, 2, 2, 2, 2, 2, 2, 2, 2, 2, 2, 2, 2, 2, 2, 2, 2, 2, 2, 2, 2, 2, 2, 2, 2, 2, 2, 2, 2, 2, 2, 2, 2, 2, 2, 2, 2, 2, 2, 2, 2, 2, 2, 2, 2, 2, 2, 2, 2, 2, 2, 2, 2, 2, 2, 2, 2, 2, 2, 2, 2, 2, 2, 2, 2, 2, 2, 2, 2, 2, 2, 2, 2, 2, 2, 2, 2, 2, 2, 2, 2, 2, 2, 2, 2, 2, 2, 2, 2, 2, 2, 2, 2, 2, 2, 2, 2, 2, 2, 2, 2, 2, 2, 2, 2, 2, 2, 2, 2, 2, 2, 2, 2, 2, 2, 2, 2, 2, 2, 2, 2, 2, 2, 2, 2, 2, 2, 2, 2, 2, 2, 2, 2, 2, 2, 2, 2, 2, 2, 3 ),
 ( 0.000000000000000000, 1.000000000000000000 ),
 ( 0.000000000000000000, 0.002777777777777777884, 0.005555555555555555768, 0.008333333333333333218, 0.01111111111111111154, 0.01388888888888888812, 0.01666666666666666644, 0.01944444444444444475, 0.02222222222222222307, 0.02500000000000000139, 0.02777777777777777624, 0.03055555555555555455, 0.03333333333333333287, 0.03611111111111110772, 0.03888888888888888951, 0.04166666666666666435, 0.04444444444444444614, 0.04722222222222222099, 0.05000000000000000278, 0.05277777777777777762, 0.05555555555555555247, 0.05833333333333333426, 0.06111111111111110911, 0.06388888888888888395, 0.06666666666666666574, 0.06944444444444444753, 0.07222222222222221544, 0.07499999999999999722, 0.07777777777777777901, 0.08055555555555556080, 0.08333333333333332871, 0.08611111111111111049, 0.08888888888888889228, 0.09166666666666666019, 0.09444444444444444198, 0.09722222222222222376, 0.1000000000000000056, 0.1027777777777777735, 0.1055555555555555552, 0.1083333333333333370, 0.1111111111111111049, 0.1138888888888888867, 0.1166666666666666685, 0.1194444444444444503, 0.1222222222222222182, 0.1250000000000000000, 0.1277777777777777679, 0.1305555555555555636, 0.1333333333333333315, 0.1361111111111110994, 0.1388888888888888951, 0.1416666666666666630, 0.1444444444444444309, 0.1472222222222222265, 0.1499999999999999944, 0.1527777777777777901, 0.1555555555555555580, 0.1583333333333333259, 0.1611111111111111216, 0.1638888888888888895, 0.1666666666666666574, 0.1694444444444444531, 0.1722222222222222210, 0.1749999999999999889, 0.1777777777777777846, 0.1805555555555555525, 0.1833333333333333204, 0.1861111111111111160, 0.1888888888888888840, 0.1916666666666666796, 0.1944444444444444475, 0.1972222222222222154, 0.2000000000000000111, 0.2027777777777777790, 0.2055555555555555469, 0.2083333333333333426, 0.2111111111111111105, 0.2138888888888888784, 0.2166666666666666741, 0.2194444444444444420, 0.2222222222222222099, 0.2250000000000000056, 0.2277777777777777735, 0.2305555555555555691, 0.2333333333333333370, 0.2361111111111111049, 0.2388888888888889006, 0.2416666666666666685, 0.2444444444444444364, 0.2472222222222222321, 0.2500000000000000000, 0.2527777777777777679, 0.2555555555555555358, 0.2583333333333333592, 0.2611111111111111271, 0.2638888888888888951, 0.2666666666666666630, 0.2694444444444444309, 0.2722222222222221988, 0.2750000000000000222, 0.2777777777777777901, 0.2805555555555555580, 0.2833333333333333259, 0.2861111111111110938, 0.2888888888888888618, 0.2916666666666666852, 0.2944444444444444531, 0.2972222222222222210, 0.2999999999999999889, 0.3027777777777777568, 0.3055555555555555802, 0.3083333333333333481, 0.3111111111111111160, 0.3138888888888888840, 0.3166666666666666519, 0.3194444444444444198, 0.3222222222222222432, 0.3250000000000000111, 0.3277777777777777790, 0.3305555555555555469, 0.3333333333333333148, 0.3361111111111111382, 0.3388888888888889062, 0.3416666666666666741, 0.3444444444444444420, 0.3472222222222222099, 0.3499999999999999778, 0.3527777777777778012, 0.3555555555555555691, 0.3583333333333333370, 0.3611111111111111049, 0.3638888888888888729, 0.3666666666666666408, 0.3694444444444444642, 0.3722222222222222321, 0.3750000000000000000, 0.3777777777777777679, 0.3805555555555555358, 0.3833333333333333592, 0.3861111111111111271, 0.3888888888888888951, 0.3916666666666666630, 0.3944444444444444309, 0.3972222222222221988, 0.4000000000000000222, 0.4027777777777777901, 0.4055555555555555580, 0.4083333333333333259, 0.4111111111111110938, 0.4138888888888888618, 0.4166666666666666852, 0.4194444444444444531, 0.4222222222222222210, 0.4249999999999999889, 0.4277777777777777568, 0.4305555555555555802, 0.4333333333333333481, 0.4361111111111111160, 0.4388888888888888840, 0.4416666666666666519, 0.4444444444444444198, 0.4472222222222222432, 0.4500000000000000111, 0.4527777777777777790, 0.4555555555555555469, 0.4583333333333333148, 0.4611111111111111382, 0.4638888888888889062, 0.4666666666666666741, 0.4694444444444444420, 0.4722222222222222099, 0.4749999999999999778, 0.4777777777777778012, 0.4805555555555555691, 0.4833333333333333370, 0.4861111111111111049, 0.4888888888888888729, 0.4916666666666666408, 0.4944444444444444642, 0.4972222222222222321, 0.5000000000000000000, 0.5027777777777777679, 0.5055555555555555358, 0.5083333333333333037, 0.5111111111111110716, 0.5138888888888888395, 0.5166666666666667185, 0.5194444444444444864, 0.5222222222222222543, 0.5250000000000000222, 0.5277777777777777901, 0.5305555555555555580, 0.5333333333333333259, 0.5361111111111110938, 0.5388888888888888618, 0.5416666666666666297, 0.5444444444444443976, 0.5472222222222222765, 0.5500000000000000444, 0.5527777777777778123, 0.5555555555555555802, 0.5583333333333333481, 0.5611111111111111160, 0.5638888888888888840, 0.5666666666666666519, 0.5694444444444444198, 0.5722222222222221877, 0.5749999999999999556, 0.5777777777777777235, 0.5805555555555556024, 0.5833333333333333703, 0.5861111111111111382, 0.5888888888888889062, 0.5916666666666666741, 0.5944444444444444420, 0.5972222222222222099, 0.5999999999999999778, 0.6027777777777777457, 0.6055555555555555136, 0.6083333333333332815, 0.6111111111111111605, 0.6138888888888889284, 0.6166666666666666963, 0.6194444444444444642, 0.6222222222222222321, 0.6250000000000000000, 0.6277777777777777679, 0.6305555555555555358, 0.6333333333333333037, 0.6361111111111110716, 0.6388888888888888395, 0.6416666666666667185, 0.6444444444444444864, 0.6472222222222222543, 0.6500000000000000222, 0.6527777777777777901, 0.6555555555555555580, 0.6583333333333333259, 0.6611111111111110938, 0.6638888888888888618, 0.6666666666666666297, 0.6694444444444443976, 0.6722222222222222765, 0.6750000000000000444, 0.6777777777777778123, 0.6805555555555555802, 0.6833333333333333481, 0.6861111111111111160, 0.6888888888888888840, 0.6916666666666666519, 0.6944444444444444198, 0.6972222222222221877, 0.6999999999999999556, 0.7027777777777777235, 0.7055555555555556024, 0.7083333333333333703, 0.7111111111111111382, 0.7138888888888889062, 0.7166666666666666741, 0.7194444444444444420, 0.7222222222222222099, 0.7249999999999999778, 0.7277777777777777457, 0.7305555555555555136, 0.7333333333333332815, 0.7361111111111111605, 0.7388888888888889284, 0.7416666666666666963, 0.7444444444444444642, 0.7472222222222222321, 0.7500000000000000000, 0.7527777777777777679, 0.7555555555555555358, 0.7583333333333333037, 0.7611111111111110716, 0.7638888888888888395, 0.7666666666666667185, 0.7694444444444444864, 0.7722222222222222543, 0.7750000000000000222, 0.7777777777777777901, 0.7805555555555555580, 0.7833333333333333259, 0.7861111111111110938, 0.7888888888888888618, 0.7916666666666666297, 0.7944444444444443976, 0.7972222222222222765, 0.8000000000000000444, 0.8027777777777778123, 0.8055555555555555802, 0.8083333333333333481, 0.8111111111111111160, 0.8138888888888888840, 0.8166666666666666519, 0.8194444444444444198, 0.8222222222222221877, 0.8249999999999999556, 0.8277777777777777235, 0.8305555555555556024, 0.8333333333333333703, 0.8361111111111111382, 0.8388888888888889062, 0.8416666666666666741, 0.8444444444444444420, 0.8472222222222222099, 0.8499999999999999778, 0.8527777777777777457, 0.8555555555555555136, 0.8583333333333332815, 0.8611111111111111605, 0.8638888888888889284, 0.8666666666666666963, 0.8694444444444444642, 0.8722222222222222321, 0.8750000000000000000, 0.8777777777777777679, 0.8805555555555555358, 0.8833333333333333037, 0.8861111111111110716, 0.8888888888888888395, 0.8916666666666667185, 0.8944444444444444864, 0.8972222222222222543, 0.9000000000000000222, 0.9027777777777777901, 0.9055555555555555580, 0.9083333333333333259, 0.9111111111111110938, 0.9138888888888888618, 0.9166666666666666297, 0.9194444444444443976, 0.9222222222222222765, 0.9250000000000000444, 0.9277777777777778123, 0.9305555555555555802, 0.9333333333333333481, 0.9361111111111111160, 0.9388888888888888840, 0.9416666666666666519, 0.9444444444444444198, 0.9472222222222221877, 0.9499999999999999556, 0.9527777777777777235, 0.9555555555555556024, 0.9583333333333333703, 0.9611111111111111382, 0.9638888888888889062, 0.9666666666666666741, 0.9694444444444444420, 0.9722222222222222099, 0.9749999999999999778 ),
 .UNSPECIFIED. ) 
 GEOMETRIC_REPRESENTATION_ITEM ( )  RATIONAL_B_SPLINE_SURFACE ( (
 ( 1.000000000000000000, 0.9659258262890683122, 1.000000000000000000, 0.9659258262890683122, 1.000000000000000000, 0.9659258262890683122, 1.000000000000000000, 0.9659258262890683122, 1.000000000000000000, 0.9659258262890683122, 1.000000000000000000, 0.9659258262890683122, 1.000000000000000000, 0.9659258262890683122, 1.000000000000000000, 0.9659258262890683122, 1.000000000000000000, 0.9659258262890683122, 1.000000000000000000, 0.9659258262890683122, 1.000000000000000000, 0.9659258262890683122, 1.000000000000000000, 0.9659258262890683122, 1.000000000000000000, 0.9659258262890683122, 1.000000000000000000, 0.9659258262890683122, 1.000000000000000000, 0.9659258262890683122, 1.000000000000000000, 0.9659258262890683122, 1.000000000000000000, 0.9659258262890683122, 1.000000000000000000, 0.9659258262890683122, 1.000000000000000000, 0.9659258262890683122, 1.000000000000000000, 0.9659258262890683122, 1.000000000000000000, 0.9659258262890683122, 1.000000000000000000, 0.9659258262890683122, 1.000000000000000000, 0.9659258262890683122, 1.000000000000000000, 0.9659258262890683122, 1.000000000000000000, 0.9659258262890683122, 1.000000000000000000, 0.9659258262890683122, 1.000000000000000000, 0.9659258262890683122, 1.000000000000000000, 0.9659258262890683122, 1.000000000000000000, 0.9659258262890683122, 1.000000000000000000, 0.9659258262890683122, 1.000000000000000000, 0.9659258262890683122, 1.000000000000000000, 0.9659258262890683122, 1.000000000000000000, 0.9659258262890683122, 1.000000000000000000, 0.9659258262890683122, 1.000000000000000000, 0.9659258262890683122, 1.000000000000000000, 0.9659258262890683122, 1.000000000000000000, 0.9659258262890683122, 1.000000000000000000, 0.9659258262890683122, 1.000000000000000000, 0.9659258262890683122, 1.000000000000000000, 0.9659258262890683122, 1.000000000000000000, 0.9659258262890683122, 1.000000000000000000, 0.9659258262890683122, 1.000000000000000000, 0.9659258262890683122, 1.000000000000000000, 0.9659258262890683122, 1.000000000000000000, 0.9659258262890683122, 1.000000000000000000, 0.9659258262890683122, 1.000000000000000000, 0.9659258262890683122, 1.000000000000000000, 0.9659258262890683122, 1.000000000000000000, 0.9659258262890683122, 1.000000000000000000, 0.9659258262890683122, 1.000000000000000000, 0.9659258262890683122, 1.000000000000000000, 0.9659258262890683122, 1.000000000000000000, 0.9659258262890683122, 1.000000000000000000, 0.9659258262890683122, 1.000000000000000000, 0.9659258262890683122, 1.000000000000000000, 0.9659258262890683122, 1.000000000000000000, 0.9659258262890683122, 1.000000000000000000, 0.9659258262890683122, 1.000000000000000000, 0.9659258262890683122, 1.000000000000000000, 0.9659258262890683122, 1.000000000000000000, 0.9659258262890683122, 1.000000000000000000, 0.9659258262890683122, 1.000000000000000000, 0.9659258262890683122, 1.000000000000000000, 0.9659258262890683122, 1.000000000000000000, 0.9659258262890683122, 1.000000000000000000, 0.9659258262890683122, 1.000000000000000000, 0.9659258262890683122, 1.000000000000000000, 0.9659258262890683122, 1.000000000000000000, 0.9659258262890683122, 1.000000000000000000, 0.9659258262890683122, 1.000000000000000000, 0.9659258262890683122, 1.000000000000000000, 0.9659258262890683122, 1.000000000000000000, 0.9659258262890683122, 1.000000000000000000, 0.9659258262890683122, 1.000000000000000000, 0.9659258262890683122, 1.000000000000000000, 0.9659258262890683122, 1.000000000000000000, 0.9659258262890683122, 1.000000000000000000, 0.9659258262890683122, 1.000000000000000000, 0.9659258262890683122, 1.000000000000000000, 0.9659258262890683122, 1.000000000000000000, 0.9659258262890683122, 1.000000000000000000, 0.9659258262890683122, 1.000000000000000000, 0.9659258262890683122, 1.000000000000000000, 0.9659258262890683122, 1.000000000000000000, 0.9659258262890683122, 1.000000000000000000, 0.9659258262890683122, 1.000000000000000000, 0.9659258262890683122, 1.000000000000000000, 0.9659258262890683122, 1.000000000000000000, 0.9659258262890683122, 1.000000000000000000, 0.9659258262890683122, 1.000000000000000000, 0.9659258262890683122, 1.000000000000000000, 0.9659258262890683122, 1.000000000000000000, 0.9659258262890683122, 1.000000000000000000, 0.9659258262890683122, 1.000000000000000000, 0.9659258262890683122, 1.000000000000000000, 0.9659258262890683122, 1.000000000000000000, 0.9659258262890683122, 1.000000000000000000, 0.9659258262890683122, 1.000000000000000000, 0.9659258262890683122, 1.000000000000000000, 0.9659258262890683122, 1.000000000000000000, 0.9659258262890683122, 1.000000000000000000, 0.9659258262890683122, 1.000000000000000000, 0.9659258262890683122, 1.000000000000000000, 0.9659258262890683122, 1.000000000000000000, 0.9659258262890683122, 1.000000000000000000, 0.9659258262890683122, 1.000000000000000000, 0.9659258262890683122, 1.000000000000000000, 0.9659258262890683122, 1.000000000000000000, 0.9659258262890683122, 1.000000000000000000, 0.9659258262890683122, 1.000000000000000000, 0.9659258262890683122, 1.000000000000000000, 0.9659258262890683122, 1.000000000000000000, 0.9659258262890683122, 1.000000000000000000, 0.9659258262890683122, 1.000000000000000000, 0.9659258262890683122, 1.000000000000000000, 0.9659258262890683122, 1.000000000000000000, 0.9659258262890683122, 1.000000000000000000, 0.9659258262890683122, 1.000000000000000000, 0.9659258262890683122, 1.000000000000000000, 0.9659258262890683122, 1.000000000000000000, 0.9659258262890683122, 1.000000000000000000, 0.9659258262890683122, 1.000000000000000000, 0.9659258262890683122, 1.000000000000000000, 0.9659258262890683122, 1.000000000000000000, 0.9659258262890683122, 1.000000000000000000, 0.9659258262890683122, 1.000000000000000000, 0.9659258262890683122, 1.000000000000000000, 0.9659258262890683122, 1.000000000000000000, 0.9659258262890683122, 1.000000000000000000, 0.9659258262890683122, 1.000000000000000000, 0.9659258262890683122, 1.000000000000000000, 0.9659258262890683122, 1.000000000000000000, 0.9659258262890683122, 1.000000000000000000, 0.9659258262890683122, 1.000000000000000000, 0.9659258262890683122, 1.000000000000000000, 0.9659258262890683122, 1.000000000000000000, 0.9659258262890683122, 1.000000000000000000, 0.9659258262890683122, 1.000000000000000000, 0.9659258262890683122, 1.000000000000000000, 0.9659258262890683122, 1.000000000000000000, 0.9659258262890683122, 1.000000000000000000, 0.9659258262890683122, 1.000000000000000000, 0.9659258262890683122, 1.000000000000000000, 0.9659258262890683122, 1.000000000000000000, 0.9659258262890683122, 1.000000000000000000, 0.9659258262890683122, 1.000000000000000000, 0.9659258262890683122, 1.000000000000000000, 0.9659258262890683122, 1.000000000000000000, 0.9659258262890683122, 1.000000000000000000, 0.9659258262890683122, 1.000000000000000000, 0.9659258262890683122, 1.000000000000000000, 0.9659258262890683122, 1.000000000000000000, 0.9659258262890683122, 1.000000000000000000, 0.9659258262890683122, 1.000000000000000000, 0.9659258262890683122, 1.000000000000000000, 0.9659258262890683122, 1.000000000000000000, 0.9659258262890683122, 1.000000000000000000, 0.9659258262890683122, 1.000000000000000000, 0.9659258262890683122, 1.000000000000000000, 0.9659258262890683122, 1.000000000000000000, 0.9659258262890683122, 1.000000000000000000, 0.9659258262890683122, 1.000000000000000000, 0.9659258262890683122, 1.000000000000000000, 0.9659258262890683122, 1.000000000000000000, 0.9659258262890683122, 1.000000000000000000, 0.9659258262890683122, 1.000000000000000000, 0.9659258262890683122, 1.000000000000000000, 0.9659258262890683122, 1.000000000000000000, 0.9659258262890683122, 1.000000000000000000, 0.9659258262890683122, 1.000000000000000000, 0.9659258262890683122, 1.000000000000000000, 0.9659258262890683122, 1.000000000000000000, 0.9659258262890683122, 1.000000000000000000, 0.9659258262890683122, 1.000000000000000000, 0.9659258262890683122, 1.000000000000000000, 0.9659258262890683122, 1.000000000000000000, 0.9659258262890683122, 1.000000000000000000, 0.9659258262890683122, 1.000000000000000000, 0.9659258262890683122, 1.000000000000000000, 0.9659258262890683122, 1.000000000000000000, 0.9659258262890683122, 1.000000000000000000, 0.9659258262890683122, 1.000000000000000000, 0.9659258262890683122, 1.000000000000000000, 0.9659258262890683122, 1.000000000000000000, 0.9659258262890683122, 1.000000000000000000, 0.9659258262890683122, 1.000000000000000000, 0.9659258262890683122, 1.000000000000000000, 0.9659258262890683122, 1.000000000000000000, 0.9659258262890683122, 1.000000000000000000, 0.9659258262890683122, 1.000000000000000000, 0.9659258262890683122, 1.000000000000000000, 0.9659258262890683122, 1.000000000000000000, 0.9659258262890683122, 1.000000000000000000, 0.9659258262890683122, 1.000000000000000000, 0.9659258262890683122, 1.000000000000000000, 0.9659258262890683122, 1.000000000000000000, 0.9659258262890683122, 1.000000000000000000, 0.9659258262890683122, 1.000000000000000000, 0.9659258262890683122, 1.000000000000000000, 0.9659258262890683122, 1.000000000000000000, 0.9659258262890683122, 1.000000000000000000, 0.9659258262890683122, 1.000000000000000000, 0.9659258262890683122, 1.000000000000000000, 0.9659258262890683122, 1.000000000000000000, 0.9659258262890683122, 1.000000000000000000, 0.9659258262890683122, 1.000000000000000000, 0.9659258262890683122, 1.000000000000000000, 0.9659258262890683122, 1.000000000000000000, 0.9659258262890683122, 1.000000000000000000, 0.9659258262890683122, 1.000000000000000000, 0.9659258262890683122, 1.000000000000000000, 0.9659258262890683122, 1.000000000000000000, 0.9659258262890683122, 1.000000000000000000, 0.9659258262890683122, 1.000000000000000000, 0.9659258262890683122, 1.000000000000000000, 0.9659258262890683122, 1.000000000000000000, 0.9659258262890683122, 1.000000000000000000, 0.9659258262890683122, 1.000000000000000000, 0.9659258262890683122, 1.000000000000000000, 0.9659258262890683122, 1.000000000000000000, 0.9659258262890683122, 1.000000000000000000, 0.9659258262890683122, 1.000000000000000000, 0.9659258262890683122, 1.000000000000000000, 0.9659258262890683122, 1.000000000000000000, 0.9659258262890683122, 1.000000000000000000, 0.9659258262890683122, 1.000000000000000000, 0.9659258262890683122, 1.000000000000000000, 0.9659258262890683122, 1.000000000000000000, 0.9659258262890683122, 1.000000000000000000, 0.9659258262890683122, 1.000000000000000000, 0.9659258262890683122, 1.000000000000000000, 0.9659258262890683122, 1.000000000000000000, 0.9659258262890683122, 1.000000000000000000, 0.9659258262890683122, 1.000000000000000000, 0.9659258262890683122, 1.000000000000000000, 0.9659258262890683122, 1.000000000000000000, 0.9659258262890683122, 1.000000000000000000, 0.9659258262890683122, 1.000000000000000000, 0.9659258262890683122, 1.000000000000000000, 0.9659258262890683122, 1.000000000000000000, 0.9659258262890683122, 1.000000000000000000, 0.9659258262890683122, 1.000000000000000000, 0.9659258262890683122, 1.000000000000000000, 0.9659258262890683122, 1.000000000000000000, 0.9659258262890683122, 1.000000000000000000, 0.9659258262890683122, 1.000000000000000000, 0.9659258262890683122, 1.000000000000000000, 0.9659258262890683122, 1.000000000000000000, 0.9659258262890683122, 1.000000000000000000, 0.9659258262890683122, 1.000000000000000000, 0.9659258262890683122, 1.000000000000000000, 0.9659258262890683122, 1.000000000000000000, 0.9659258262890683122, 1.000000000000000000, 0.9659258262890683122, 1.000000000000000000, 0.9659258262890683122, 1.000000000000000000, 0.9659258262890683122, 1.000000000000000000, 0.9659258262890683122, 1.000000000000000000, 0.9659258262890683122, 1.000000000000000000, 0.9659258262890683122, 1.000000000000000000, 0.9659258262890683122, 1.000000000000000000, 0.9659258262890683122, 1.000000000000000000, 0.9659258262890683122, 1.000000000000000000, 0.9659258262890683122, 1.000000000000000000, 0.9659258262890683122, 1.000000000000000000, 0.9659258262890683122, 1.000000000000000000, 0.9659258262890683122, 1.000000000000000000, 0.9659258262890683122, 1.000000000000000000, 0.9659258262890683122, 1.000000000000000000, 0.9659258262890683122, 1.000000000000000000, 0.9659258262890683122, 1.000000000000000000, 0.9659258262890683122, 1.000000000000000000, 0.9659258262890683122, 1.000000000000000000, 0.9659258262890683122, 1.000000000000000000, 0.9659258262890683122, 1.000000000000000000, 0.9659258262890683122, 1.000000000000000000, 0.9659258262890683122, 1.000000000000000000, 0.9659258262890683122, 1.000000000000000000, 0.9659258262890683122, 1.000000000000000000, 0.9659258262890683122, 1.000000000000000000, 0.9659258262890683122, 1.000000000000000000, 0.9659258262890683122, 1.000000000000000000, 0.9659258262890683122, 1.000000000000000000, 0.9659258262890683122, 1.000000000000000000, 0.9659258262890683122, 1.000000000000000000, 0.9659258262890683122, 1.000000000000000000, 0.9659258262890683122, 1.000000000000000000, 0.9659258262890683122, 1.000000000000000000, 0.9659258262890683122, 1.000000000000000000, 0.9659258262890683122, 1.000000000000000000, 0.9659258262890683122, 1.000000000000000000, 0.9659258262890683122, 1.000000000000000000, 0.9659258262890683122, 1.000000000000000000, 0.9659258262890683122, 1.000000000000000000, 0.9659258262890683122, 1.000000000000000000, 0.9659258262890683122, 1.000000000000000000, 0.9659258262890683122, 1.000000000000000000, 0.9659258262890683122, 1.000000000000000000, 0.9659258262890683122, 1.000000000000000000, 0.9659258262890683122, 1.000000000000000000, 0.9659258262890683122, 1.000000000000000000, 0.9659258262890683122, 1.000000000000000000, 0.9659258262890683122, 1.000000000000000000, 0.9659258262890683122, 1.000000000000000000, 0.9659258262890683122, 1.000000000000000000, 0.9659258262890683122, 1.000000000000000000, 0.9659258262890683122, 1.000000000000000000, 0.9659258262890683122, 1.000000000000000000, 0.9659258262890683122, 1.000000000000000000, 0.9659258262890683122, 1.000000000000000000, 0.9659258262890683122, 1.000000000000000000, 0.9659258262890683122, 1.000000000000000000, 0.9659258262890683122, 1.000000000000000000, 0.9659258262890683122, 1.000000000000000000, 0.9659258262890683122, 1.000000000000000000, 0.9659258262890683122, 1.000000000000000000, 0.9659258262890683122, 1.000000000000000000, 0.9659258262890683122, 1.000000000000000000, 0.9659258262890683122, 1.000000000000000000, 0.9659258262890683122, 1.000000000000000000, 0.9659258262890683122, 1.000000000000000000, 0.9659258262890683122, 1.000000000000000000, 0.9659258262890683122, 1.000000000000000000, 0.9659258262890683122, 1.000000000000000000, 0.9659258262890683122, 1.000000000000000000, 0.9659258262890683122, 1.000000000000000000, 0.9659258262890683122, 1.000000000000000000, 0.9659258262890683122, 1.000000000000000000, 0.9659258262890683122, 1.000000000000000000, 0.9659258262890683122, 1.000000000000000000, 0.9659258262890683122, 1.000000000000000000, 0.9659258262890683122, 1.000000000000000000, 0.9659258262890683122, 1.000000000000000000, 0.9659258262890683122, 1.000000000000000000, 0.9659258262890683122, 1.000000000000000000, 0.9659258262890683122, 1.000000000000000000, 0.9659258262890683122, 1.000000000000000000, 0.9659258262890683122, 1.000000000000000000, 0.9659258262890683122, 1.000000000000000000, 0.9659258262890683122, 1.000000000000000000, 0.9659258262890683122, 1.000000000000000000, 0.9659258262890683122, 1.000000000000000000, 0.9659258262890683122, 1.000000000000000000, 0.9659258262890683122, 1.000000000000000000, 0.9659258262890683122, 1.000000000000000000, 0.9659258262890683122, 1.000000000000000000, 0.9659258262890683122, 1.000000000000000000, 0.9659258262890683122, 1.000000000000000000, 0.9659258262890683122, 1.000000000000000000, 0.9659258262890683122, 1.000000000000000000, 0.9659258262890683122, 1.000000000000000000, 0.9659258262890683122, 1.000000000000000000),
 ( 1.000000000000000000, 0.9659258262890683122, 1.000000000000000000, 0.9659258262890683122, 1.000000000000000000, 0.9659258262890683122, 1.000000000000000000, 0.9659258262890683122, 1.000000000000000000, 0.9659258262890683122, 1.000000000000000000, 0.9659258262890683122, 1.000000000000000000, 0.9659258262890683122, 1.000000000000000000, 0.9659258262890683122, 1.000000000000000000, 0.9659258262890683122, 1.000000000000000000, 0.9659258262890683122, 1.000000000000000000, 0.9659258262890683122, 1.000000000000000000, 0.9659258262890683122, 1.000000000000000000, 0.9659258262890683122, 1.000000000000000000, 0.9659258262890683122, 1.000000000000000000, 0.9659258262890683122, 1.000000000000000000, 0.9659258262890683122, 1.000000000000000000, 0.9659258262890683122, 1.000000000000000000, 0.9659258262890683122, 1.000000000000000000, 0.9659258262890683122, 1.000000000000000000, 0.9659258262890683122, 1.000000000000000000, 0.9659258262890683122, 1.000000000000000000, 0.9659258262890683122, 1.000000000000000000, 0.9659258262890683122, 1.000000000000000000, 0.9659258262890683122, 1.000000000000000000, 0.9659258262890683122, 1.000000000000000000, 0.9659258262890683122, 1.000000000000000000, 0.9659258262890683122, 1.000000000000000000, 0.9659258262890683122, 1.000000000000000000, 0.9659258262890683122, 1.000000000000000000, 0.9659258262890683122, 1.000000000000000000, 0.9659258262890683122, 1.000000000000000000, 0.9659258262890683122, 1.000000000000000000, 0.9659258262890683122, 1.000000000000000000, 0.9659258262890683122, 1.000000000000000000, 0.9659258262890683122, 1.000000000000000000, 0.9659258262890683122, 1.000000000000000000, 0.9659258262890683122, 1.000000000000000000, 0.9659258262890683122, 1.000000000000000000, 0.9659258262890683122, 1.000000000000000000, 0.9659258262890683122, 1.000000000000000000, 0.9659258262890683122, 1.000000000000000000, 0.9659258262890683122, 1.000000000000000000, 0.9659258262890683122, 1.000000000000000000, 0.9659258262890683122, 1.000000000000000000, 0.9659258262890683122, 1.000000000000000000, 0.9659258262890683122, 1.000000000000000000, 0.9659258262890683122, 1.000000000000000000, 0.9659258262890683122, 1.000000000000000000, 0.9659258262890683122, 1.000000000000000000, 0.9659258262890683122, 1.000000000000000000, 0.9659258262890683122, 1.000000000000000000, 0.9659258262890683122, 1.000000000000000000, 0.9659258262890683122, 1.000000000000000000, 0.9659258262890683122, 1.000000000000000000, 0.9659258262890683122, 1.000000000000000000, 0.9659258262890683122, 1.000000000000000000, 0.9659258262890683122, 1.000000000000000000, 0.9659258262890683122, 1.000000000000000000, 0.9659258262890683122, 1.000000000000000000, 0.9659258262890683122, 1.000000000000000000, 0.9659258262890683122, 1.000000000000000000, 0.9659258262890683122, 1.000000000000000000, 0.9659258262890683122, 1.000000000000000000, 0.9659258262890683122, 1.000000000000000000, 0.9659258262890683122, 1.000000000000000000, 0.9659258262890683122, 1.000000000000000000, 0.9659258262890683122, 1.000000000000000000, 0.9659258262890683122, 1.000000000000000000, 0.9659258262890683122, 1.000000000000000000, 0.9659258262890683122, 1.000000000000000000, 0.9659258262890683122, 1.000000000000000000, 0.9659258262890683122, 1.000000000000000000, 0.9659258262890683122, 1.000000000000000000, 0.9659258262890683122, 1.000000000000000000, 0.9659258262890683122, 1.000000000000000000, 0.9659258262890683122, 1.000000000000000000, 0.9659258262890683122, 1.000000000000000000, 0.9659258262890683122, 1.000000000000000000, 0.9659258262890683122, 1.000000000000000000, 0.9659258262890683122, 1.000000000000000000, 0.9659258262890683122, 1.000000000000000000, 0.9659258262890683122, 1.000000000000000000, 0.9659258262890683122, 1.000000000000000000, 0.9659258262890683122, 1.000000000000000000, 0.9659258262890683122, 1.000000000000000000, 0.9659258262890683122, 1.000000000000000000, 0.9659258262890683122, 1.000000000000000000, 0.9659258262890683122, 1.000000000000000000, 0.9659258262890683122, 1.000000000000000000, 0.9659258262890683122, 1.000000000000000000, 0.9659258262890683122, 1.000000000000000000, 0.9659258262890683122, 1.000000000000000000, 0.9659258262890683122, 1.000000000000000000, 0.9659258262890683122, 1.000000000000000000, 0.9659258262890683122, 1.000000000000000000, 0.9659258262890683122, 1.000000000000000000, 0.9659258262890683122, 1.000000000000000000, 0.9659258262890683122, 1.000000000000000000, 0.9659258262890683122, 1.000000000000000000, 0.9659258262890683122, 1.000000000000000000, 0.9659258262890683122, 1.000000000000000000, 0.9659258262890683122, 1.000000000000000000, 0.9659258262890683122, 1.000000000000000000, 0.9659258262890683122, 1.000000000000000000, 0.9659258262890683122, 1.000000000000000000, 0.9659258262890683122, 1.000000000000000000, 0.9659258262890683122, 1.000000000000000000, 0.9659258262890683122, 1.000000000000000000, 0.9659258262890683122, 1.000000000000000000, 0.9659258262890683122, 1.000000000000000000, 0.9659258262890683122, 1.000000000000000000, 0.9659258262890683122, 1.000000000000000000, 0.9659258262890683122, 1.000000000000000000, 0.9659258262890683122, 1.000000000000000000, 0.9659258262890683122, 1.000000000000000000, 0.9659258262890683122, 1.000000000000000000, 0.9659258262890683122, 1.000000000000000000, 0.9659258262890683122, 1.000000000000000000, 0.9659258262890683122, 1.000000000000000000, 0.9659258262890683122, 1.000000000000000000, 0.9659258262890683122, 1.000000000000000000, 0.9659258262890683122, 1.000000000000000000, 0.9659258262890683122, 1.000000000000000000, 0.9659258262890683122, 1.000000000000000000, 0.9659258262890683122, 1.000000000000000000, 0.9659258262890683122, 1.000000000000000000, 0.9659258262890683122, 1.000000000000000000, 0.9659258262890683122, 1.000000000000000000, 0.9659258262890683122, 1.000000000000000000, 0.9659258262890683122, 1.000000000000000000, 0.9659258262890683122, 1.000000000000000000, 0.9659258262890683122, 1.000000000000000000, 0.9659258262890683122, 1.000000000000000000, 0.9659258262890683122, 1.000000000000000000, 0.9659258262890683122, 1.000000000000000000, 0.9659258262890683122, 1.000000000000000000, 0.9659258262890683122, 1.000000000000000000, 0.9659258262890683122, 1.000000000000000000, 0.9659258262890683122, 1.000000000000000000, 0.9659258262890683122, 1.000000000000000000, 0.9659258262890683122, 1.000000000000000000, 0.9659258262890683122, 1.000000000000000000, 0.9659258262890683122, 1.000000000000000000, 0.9659258262890683122, 1.000000000000000000, 0.9659258262890683122, 1.000000000000000000, 0.9659258262890683122, 1.000000000000000000, 0.9659258262890683122, 1.000000000000000000, 0.9659258262890683122, 1.000000000000000000, 0.9659258262890683122, 1.000000000000000000, 0.9659258262890683122, 1.000000000000000000, 0.9659258262890683122, 1.000000000000000000, 0.9659258262890683122, 1.000000000000000000, 0.9659258262890683122, 1.000000000000000000, 0.9659258262890683122, 1.000000000000000000, 0.9659258262890683122, 1.000000000000000000, 0.9659258262890683122, 1.000000000000000000, 0.9659258262890683122, 1.000000000000000000, 0.9659258262890683122, 1.000000000000000000, 0.9659258262890683122, 1.000000000000000000, 0.9659258262890683122, 1.000000000000000000, 0.9659258262890683122, 1.000000000000000000, 0.9659258262890683122, 1.000000000000000000, 0.9659258262890683122, 1.000000000000000000, 0.9659258262890683122, 1.000000000000000000, 0.9659258262890683122, 1.000000000000000000, 0.9659258262890683122, 1.000000000000000000, 0.9659258262890683122, 1.000000000000000000, 0.9659258262890683122, 1.000000000000000000, 0.9659258262890683122, 1.000000000000000000, 0.9659258262890683122, 1.000000000000000000, 0.9659258262890683122, 1.000000000000000000, 0.9659258262890683122, 1.000000000000000000, 0.9659258262890683122, 1.000000000000000000, 0.9659258262890683122, 1.000000000000000000, 0.9659258262890683122, 1.000000000000000000, 0.9659258262890683122, 1.000000000000000000, 0.9659258262890683122, 1.000000000000000000, 0.9659258262890683122, 1.000000000000000000, 0.9659258262890683122, 1.000000000000000000, 0.9659258262890683122, 1.000000000000000000, 0.9659258262890683122, 1.000000000000000000, 0.9659258262890683122, 1.000000000000000000, 0.9659258262890683122, 1.000000000000000000, 0.9659258262890683122, 1.000000000000000000, 0.9659258262890683122, 1.000000000000000000, 0.9659258262890683122, 1.000000000000000000, 0.9659258262890683122, 1.000000000000000000, 0.9659258262890683122, 1.000000000000000000, 0.9659258262890683122, 1.000000000000000000, 0.9659258262890683122, 1.000000000000000000, 0.9659258262890683122, 1.000000000000000000, 0.9659258262890683122, 1.000000000000000000, 0.9659258262890683122, 1.000000000000000000, 0.9659258262890683122, 1.000000000000000000, 0.9659258262890683122, 1.000000000000000000, 0.9659258262890683122, 1.000000000000000000, 0.9659258262890683122, 1.000000000000000000, 0.9659258262890683122, 1.000000000000000000, 0.9659258262890683122, 1.000000000000000000, 0.9659258262890683122, 1.000000000000000000, 0.9659258262890683122, 1.000000000000000000, 0.9659258262890683122, 1.000000000000000000, 0.9659258262890683122, 1.000000000000000000, 0.9659258262890683122, 1.000000000000000000, 0.9659258262890683122, 1.000000000000000000, 0.9659258262890683122, 1.000000000000000000, 0.9659258262890683122, 1.000000000000000000, 0.9659258262890683122, 1.000000000000000000, 0.9659258262890683122, 1.000000000000000000, 0.9659258262890683122, 1.000000000000000000, 0.9659258262890683122, 1.000000000000000000, 0.9659258262890683122, 1.000000000000000000, 0.9659258262890683122, 1.000000000000000000, 0.9659258262890683122, 1.000000000000000000, 0.9659258262890683122, 1.000000000000000000, 0.9659258262890683122, 1.000000000000000000, 0.9659258262890683122, 1.000000000000000000, 0.9659258262890683122, 1.000000000000000000, 0.9659258262890683122, 1.000000000000000000, 0.9659258262890683122, 1.000000000000000000, 0.9659258262890683122, 1.000000000000000000, 0.9659258262890683122, 1.000000000000000000, 0.9659258262890683122, 1.000000000000000000, 0.9659258262890683122, 1.000000000000000000, 0.9659258262890683122, 1.000000000000000000, 0.9659258262890683122, 1.000000000000000000, 0.9659258262890683122, 1.000000000000000000, 0.9659258262890683122, 1.000000000000000000, 0.9659258262890683122, 1.000000000000000000, 0.9659258262890683122, 1.000000000000000000, 0.9659258262890683122, 1.000000000000000000, 0.9659258262890683122, 1.000000000000000000, 0.9659258262890683122, 1.000000000000000000, 0.9659258262890683122, 1.000000000000000000, 0.9659258262890683122, 1.000000000000000000, 0.9659258262890683122, 1.000000000000000000, 0.9659258262890683122, 1.000000000000000000, 0.9659258262890683122, 1.000000000000000000, 0.9659258262890683122, 1.000000000000000000, 0.9659258262890683122, 1.000000000000000000, 0.9659258262890683122, 1.000000000000000000, 0.9659258262890683122, 1.000000000000000000, 0.9659258262890683122, 1.000000000000000000, 0.9659258262890683122, 1.000000000000000000, 0.9659258262890683122, 1.000000000000000000, 0.9659258262890683122, 1.000000000000000000, 0.9659258262890683122, 1.000000000000000000, 0.9659258262890683122, 1.000000000000000000, 0.9659258262890683122, 1.000000000000000000, 0.9659258262890683122, 1.000000000000000000, 0.9659258262890683122, 1.000000000000000000, 0.9659258262890683122, 1.000000000000000000, 0.9659258262890683122, 1.000000000000000000, 0.9659258262890683122, 1.000000000000000000, 0.9659258262890683122, 1.000000000000000000, 0.9659258262890683122, 1.000000000000000000, 0.9659258262890683122, 1.000000000000000000, 0.9659258262890683122, 1.000000000000000000, 0.9659258262890683122, 1.000000000000000000, 0.9659258262890683122, 1.000000000000000000, 0.9659258262890683122, 1.000000000000000000, 0.9659258262890683122, 1.000000000000000000, 0.9659258262890683122, 1.000000000000000000, 0.9659258262890683122, 1.000000000000000000, 0.9659258262890683122, 1.000000000000000000, 0.9659258262890683122, 1.000000000000000000, 0.9659258262890683122, 1.000000000000000000, 0.9659258262890683122, 1.000000000000000000, 0.9659258262890683122, 1.000000000000000000, 0.9659258262890683122, 1.000000000000000000, 0.9659258262890683122, 1.000000000000000000, 0.9659258262890683122, 1.000000000000000000, 0.9659258262890683122, 1.000000000000000000, 0.9659258262890683122, 1.000000000000000000, 0.9659258262890683122, 1.000000000000000000, 0.9659258262890683122, 1.000000000000000000, 0.9659258262890683122, 1.000000000000000000, 0.9659258262890683122, 1.000000000000000000, 0.9659258262890683122, 1.000000000000000000, 0.9659258262890683122, 1.000000000000000000, 0.9659258262890683122, 1.000000000000000000, 0.9659258262890683122, 1.000000000000000000, 0.9659258262890683122, 1.000000000000000000, 0.9659258262890683122, 1.000000000000000000, 0.9659258262890683122, 1.000000000000000000, 0.9659258262890683122, 1.000000000000000000, 0.9659258262890683122, 1.000000000000000000, 0.9659258262890683122, 1.000000000000000000, 0.9659258262890683122, 1.000000000000000000, 0.9659258262890683122, 1.000000000000000000, 0.9659258262890683122, 1.000000000000000000, 0.9659258262890683122, 1.000000000000000000, 0.9659258262890683122, 1.000000000000000000, 0.9659258262890683122, 1.000000000000000000, 0.9659258262890683122, 1.000000000000000000, 0.9659258262890683122, 1.000000000000000000, 0.9659258262890683122, 1.000000000000000000, 0.9659258262890683122, 1.000000000000000000, 0.9659258262890683122, 1.000000000000000000, 0.9659258262890683122, 1.000000000000000000, 0.9659258262890683122, 1.000000000000000000, 0.9659258262890683122, 1.000000000000000000, 0.9659258262890683122, 1.000000000000000000, 0.9659258262890683122, 1.000000000000000000, 0.9659258262890683122, 1.000000000000000000, 0.9659258262890683122, 1.000000000000000000, 0.9659258262890683122, 1.000000000000000000, 0.9659258262890683122, 1.000000000000000000, 0.9659258262890683122, 1.000000000000000000, 0.9659258262890683122, 1.000000000000000000, 0.9659258262890683122, 1.000000000000000000, 0.9659258262890683122, 1.000000000000000000, 0.9659258262890683122, 1.000000000000000000, 0.9659258262890683122, 1.000000000000000000, 0.9659258262890683122, 1.000000000000000000, 0.9659258262890683122, 1.000000000000000000, 0.9659258262890683122, 1.000000000000000000, 0.9659258262890683122, 1.000000000000000000, 0.9659258262890683122, 1.000000000000000000, 0.9659258262890683122, 1.000000000000000000, 0.9659258262890683122, 1.000000000000000000, 0.9659258262890683122, 1.000000000000000000, 0.9659258262890683122, 1.000000000000000000, 0.9659258262890683122, 1.000000000000000000, 0.9659258262890683122, 1.000000000000000000, 0.9659258262890683122, 1.000000000000000000, 0.9659258262890683122, 1.000000000000000000, 0.9659258262890683122, 1.000000000000000000, 0.9659258262890683122, 1.000000000000000000, 0.9659258262890683122, 1.000000000000000000, 0.9659258262890683122, 1.000000000000000000, 0.9659258262890683122, 1.000000000000000000, 0.9659258262890683122, 1.000000000000000000, 0.9659258262890683122, 1.000000000000000000, 0.9659258262890683122, 1.000000000000000000, 0.9659258262890683122, 1.000000000000000000, 0.9659258262890683122, 1.000000000000000000, 0.9659258262890683122, 1.000000000000000000, 0.9659258262890683122, 1.000000000000000000, 0.9659258262890683122, 1.000000000000000000, 0.9659258262890683122, 1.000000000000000000, 0.9659258262890683122, 1.000000000000000000, 0.9659258262890683122, 1.000000000000000000, 0.9659258262890683122, 1.000000000000000000, 0.9659258262890683122, 1.000000000000000000, 0.9659258262890683122, 1.000000000000000000, 0.9659258262890683122, 1.000000000000000000, 0.9659258262890683122, 1.000000000000000000, 0.9659258262890683122, 1.000000000000000000, 0.9659258262890683122, 1.000000000000000000, 0.9659258262890683122, 1.000000000000000000) ) ) 
 REPRESENTATION_ITEM ( '' )  SURFACE ( )  );
#90883=CARTESIAN_POINT ( 'NONE',  ( 72.53709685856478018, -3.054999999999998828, -5.291415217122919401 ) ) ;
#90891=CARTESIAN_POINT ( 'NONE',  ( 122.6250000000000000, -7.950000000000000178, -4.867971026610729436E-16 ) ) ;
#90895=DIRECTION ( 'NONE',  ( -1.000000000000000000, -0.000000000000000000, -0.000000000000000000 ) ) ;
#90906=CARTESIAN_POINT ( 'NONE',  ( 27.27126352523142927, 4.472830434245838482, 4.472830434245842035 ) ) ;
#90956=CARTESIAN_POINT ( 'NONE',  ( 53.14126352523144448, 4.472830434245837594, 4.472830434245841147 ) ) ;
#90972=DIRECTION ( 'NONE',  ( 0.000000000000000000, 0.000000000000000000, 1.000000000000000000 ) ) ;
#90983=CARTESIAN_POINT ( 'NONE',  ( 76.20419371712955581, -6.884901960086285300, -3.975000000000000089 ) ) ;
#90988=CARTESIAN_POINT ( 'NONE',  ( 72.02083333333334281, 7.949999999999999289, 2.130196079827431532 ) ) ;
#91000=CARTESIAN_POINT ( 'NONE',  ( 67.22959685856476142, -6.110000000000000320, -1.637169565754161393 ) ) ;
#91008=CARTESIAN_POINT ( 'NONE',  ( 43.29166666666665719, 3.975000000000003642, -6.884901960086285300 ) ) ;
#91021=CARTESIAN_POINT ( 'NONE',  ( 52.06293019189809712, 1.637169565754157174, 6.110000000000002984 ) ) ;
#91048=CARTESIAN_POINT ( 'NONE',  ( 37.41252705046288440, -7.949999999999998401, -4.867971026610728450E-16 ) ) ;
#91056=CARTESIAN_POINT ( 'NONE',  ( 99.07876352523145158, -7.482591942790325086E-16, 6.109999999999998543 ) ) ;
#91067=EDGE_CURVE ( 'NONE', #140445, #2581, #56434, .T. ) ;
#91079=CARTESIAN_POINT ( 'NONE',  ( 54.54209685856477563, 5.291415217122923842, -3.054999999999996163 ) ) ;
#91084=CARTESIAN_POINT ( 'NONE',  ( 94.06293019189810423, 1.637169565754157174, 6.110000000000002984 ) ) ;
#91096=FACE_OUTER_BOUND ( 'NONE', #24826, .T. ) ;
#91153=CARTESIAN_POINT ( 'NONE',  ( 107.2666937171295558, -7.949999999999999289, 2.130196079827424427 ) ) ;
#91173=CARTESIAN_POINT ( 'NONE',  ( 96.83376352523144703, 6.110000000000001208, 1.122388791418549305E-15 ) ) ;
#91200=CARTESIAN_POINT ( 'NONE',  ( 78.75043019189810423, 3.055000000000002824, -5.291415217122919401 ) ) ;
#91210=VERTEX_POINT ( 'NONE', #90852 ) ;
#91214=CARTESIAN_POINT ( 'NONE',  ( 76.62043019189812298, 3.055000000000001936, -5.291415217122916737 ) ) ;
#91235=ORIENTED_EDGE ( 'NONE', *, *, #49164, .T. ) ;
#91260=CARTESIAN_POINT ( 'NONE',  ( 117.8337635252314470, 6.110000000000001208, 1.122388791418549305E-15 ) ) ;
#91336=VECTOR ( 'NONE', #24709, 1000.000000000000000 ) ;
#91340=CARTESIAN_POINT ( 'NONE',  ( 93.89583333333331439, -2.130196079827427091, 7.949999999999999289 ) ) ;
#91346=CARTESIAN_POINT ( 'NONE',  ( 12.53018939210443428, 8.713309148047983399, 3.789081179538163369 ) ) ;
#91359=CARTESIAN_POINT ( 'NONE',  ( 26.99999999999998579, 5.473733291157039993, 4.253954074006194297 ) ) ;
#91362=CARTESIAN_POINT ( 'NONE',  ( 86.55836038379621300, -7.949999999999996625, -2.130196079827426203 ) ) ;
#91366=CARTESIAN_POINT ( 'NONE',  ( 110.9795968585647756, 6.109999999999999432, 1.637169565754164280 ) ) ;
#91370=CARTESIAN_POINT ( 'NONE',  ( 100.4583333333333286, 3.974999999999997424, 6.884901960086288852 ) ) ;
#91375=CARTESIAN_POINT ( 'NONE',  ( 103.4537635252314516, -6.109999999999998543, -3.741295971395162543E-16 ) ) ;
#91380=CARTESIAN_POINT ( 'NONE',  ( 98.41666666666667140, -6.884901960086287076, -3.975000000000000977 ) ) ;
#91390=CARTESIAN_POINT ( 'NONE',  ( 29.37043019189811233, -3.055000000000001492, 5.291415217122917625 ) ) ;
#91395=ORIENTED_EDGE ( 'NONE', *, *, #111056, .F. ) ;
#91412=CARTESIAN_POINT ( 'NONE',  ( 41.91209685856478728, 5.291415217122921177, -3.054999999999994831 ) ) ;
#91446=CARTESIAN_POINT ( 'NONE',  ( 109.5787635252314516, -7.482591942790327058E-16, 6.109999999999999432 ) ) ;
#91495=CARTESIAN_POINT ( 'NONE',  ( 119.5624999999999716, -5.819803920172572198, -5.819803920172573086 ) ) ;
#91497=VERTEX_POINT ( 'NONE', #125245 ) ;
#91508=CARTESIAN_POINT ( 'NONE',  ( 108.2087635252314470, -7.482591942790329030E-16, 6.110000000000001208 ) ) ;
#91516=CARTESIAN_POINT ( 'NONE',  ( 49.66252705046289861, 7.949999999999998401, 1.460391307983218338E-15 ) ) ;
#91521=CARTESIAN_POINT ( 'NONE',  ( 36.58333333333332860, 6.884901960086290629, -3.974999999999994316 ) ) ;
#91530=CARTESIAN_POINT ( 'NONE',  ( 38.50043019189809712, -3.055000000000002380, 5.291415217122920289 ) ) ;
#91543=CARTESIAN_POINT ( 'NONE',  ( 38.57919371712956291, 3.975000000000002753, -6.884901960086283523 ) ) ;
#91549=CARTESIAN_POINT ( 'NONE',  ( 55.76626352523145869, 4.472830434245839371, -4.472830434245838482 ) ) ;
#91551=CARTESIAN_POINT ( 'NONE',  ( 124.6666666666666572, 6.884901960086285300, 3.975000000000003642 ) ) ;
#91561=VERTEX_POINT ( 'NONE', #68750 ) ;
#91575=CARTESIAN_POINT ( 'NONE',  ( 66.55793019189812298, 6.110000000000000320, -1.637169565754156064 ) ) ;
#91622=CARTESIAN_POINT ( 'NONE',  ( 27.68749999999998579, -5.819803920172573974, 5.819803920172573086 ) ) ;
#91647=CARTESIAN_POINT ( 'NONE',  ( 56.20376352523144448, 6.109999999999999432, 1.122388791418549108E-15 ) ) ;
#91649=CARTESIAN_POINT ( 'NONE',  ( 31.28752705046289151, 0.000000000000000000, -7.949999999999998401 ) ) ;
#91667=CARTESIAN_POINT ( 'NONE',  ( 117.6666666666666714, 6.884901960086285300, 3.975000000000003642 ) ) ;
#91668=CARTESIAN_POINT ( 'NONE',  ( 76.05836038379621300, -7.949999999999997513, -2.130196079827425759 ) ) ;
#91672=CARTESIAN_POINT ( 'NONE',  ( 67.93750000000000000, 5.819803920172573974, -5.819803920172572198 ) ) ;
#91683=CARTESIAN_POINT ( 'NONE',  ( 63.87543019189810423, -5.291415217122920289, -3.055000000000001492 ) ) ;
#91689=CARTESIAN_POINT ( 'NONE',  ( 43.72916666666666430, 7.950000000000001954, -2.130196079827421762 ) ) ;
#91724=CARTESIAN_POINT ( 'NONE',  ( 37.70419371712956291, -6.884901960086285300, -3.975000000000000089 ) ) ;
#91732=CARTESIAN_POINT ( 'NONE',  ( 97.76626352523145158, 4.472830434245838482, -4.472830434245837594 ) ) ;
#91744=CARTESIAN_POINT ( 'NONE',  ( 69.25000000000000000, -9.735942053221458872E-16, 7.950000000000000178 ) ) ;
#91754=CARTESIAN_POINT ( 'NONE',  ( 54.39626352523143993, 4.472830434245840259, -4.472830434245838482 ) ) ;
#91774=CARTESIAN_POINT ( 'NONE',  ( 128.3912635252314374, -4.472830434245839371, -4.472830434245839371 ) ) ;
#91820=CARTESIAN_POINT ( 'NONE',  ( 0.000000000000000000, 9.735942053221458872E-16, -7.950000000000000178 ) ) ;
#91829=CARTESIAN_POINT ( 'NONE',  ( 104.9333603837962130, 2.130196079827431532, -7.949999999999997513 ) ) ;
#91830=CARTESIAN_POINT ( 'NONE',  ( 71.87500000000000000, 7.950000000000000178, 1.460391307983218535E-15 ) ) ;
#91845=CARTESIAN_POINT ( 'NONE',  ( 93.18793019189809002, 6.110000000000002984, -1.637169565754156730 ) ) ;
#91857=CARTESIAN_POINT ( 'NONE',  ( 0.000000000000000000, 0.000000000000000000, 7.950000000000000178 ) ) ;
#91870=CARTESIAN_POINT ( 'NONE',  ( 85.16709685856477563, -3.055000000000000160, -5.291415217122921177 ) ) ;
#91882=CARTESIAN_POINT ( 'NONE',  ( 74.57876352523145158, -7.482591942790325086E-16, 6.109999999999998543 ) ) ;
#91915=( BOUNDED_SURFACE ( )  B_SPLINE_SURFACE ( 1, 2, ( 
 ( #127822, #7423, #3320, #91774, #95159, #29193, #36000, #73434, #18287, #51684, #36674, #134597, #103349, #35295, #48272, #79538, #24382, #68631, #112814, #2609, #13471, #46916, #101945, #135317, #80226, #124410, #135998, #14921, #42244, #85003, #132103, #66136, #85703, #131375, #109609, #40802, #108865, #110301, #10978, #75574, #10287, #32058, #97269, #8816, #63979, #141540, #140125, #119743, #19745, #118333, #108149, #86455, #95877, #74140, #129948, #98036, #130682, #30649, #76290, #9559, #20443, #53832, #119055, #21175, #129211, #74880, #53074, #42955, #31355, #142269, #64695, #87152, #65431, #29898, #21886, #120447, #54546, #19036, #32797, #107468, #63300, #98724, #8131, #142953, #43645, #87864, #52371, #77020, #121193, #96558, #140796, #41494, #121893, #55982, #47275, #67572, #36348, #57398, #13128, #89294, #78423, #124065, #88601, #133519, #122621, #2241, #34206, #101578, #45811, #46553, #24740, #99426, #124771, #45117, #13839, #113895, #135659, #66835, #69712, #79892, #55246, #90742, #68986, #23292, #25442, #134969, #80576, #22566, #111764, #35667, #111014, #100180, #91446, #12430, #91, #113165, #58136, #56713, #102333, #100874, #44394, #1529, #830, #2981, #68298, #123375, #132832, #33516, #89987, #77717, #11694, #134236, #34929, #79171, #24039, #112475, #105846, #84161, #93577, #37046, #126205, #138512, #39199, #39942, #26185, #60256, #116015, #128360, #137083, #115274, #83425, #127638, #59545, #50085, #105157, #16720, #104432, #28331, #126887, #60998, #71849, #72592, #14583, #29032, #5810, #70447, #82708, #114592, #116747, #94276, #17428, #61685, #73269, #15964, #5093, #3664, #50786, #58865, #4346, #6505, #94974, #103025, #27584, #47961, #92125, #137810, #139247, #136355, #49394, #71129, #26882, #38485, #81294, #125498, #82026, #15260, #103700, #48650, #92847, #37785, #107293, #119575, #107979, #52203, #97860, #130506, #141352, #75400, #42785, #86976, #106555, #20271, #131199, #20993, #31886, #97093, #117433, #73967, #85525, #64512, #18108, #31185, #10124, #43478, #19573, #7239, #41316, #129762, #131925, #120277, #87690, #98560, #62392, #108688, #76107, #65256, #63118, #9374, #109439, #51514, #95706, #53649, #139958, #96392, #54385, #52889, #63817, #142099, #142787, #32618, #140630, #118885, #8652, #40636, #84839, #129046, #29718, #118144, #42068, #86282, #18851, #7964, #30463, #74704, #143491, #21724, #668, #44211, #88427, #134064, #10815, #78261, #76850, #122444, #100720, #1365, #44959, #22403, #23109, #34753, #132667, #89136, #79729, #134799, #89822, #100004, #121025, #133354, #78990, #111583, #12262, #101414, #65978, #123198, #67394, #56549, #45648, #34046, #110135, #66667, #35496, #23871, #55078, #33359, #99248, #68136, #46376, #77557, #2065, #112314, #12963, #121727, #110831, #57240, #90562, #11521, #123912, #55802, #95377, #62779, #94649, #117121, #38867, #93951, #5494, #83087, #81687, #61382, #104827, #59919, #49772, #127290, #37449, #15630, #27254, #39601, #29404, #138184, #18504, #83833, #138908, #71502, #62069, #115665, #106961, #27988, #126564, #17795, #50465, #105527, #106228, #128727, #16360, #6900, #40323, #70805, #128041, #17114, #72258, #28721, #73639, #7641, #116428, #104087, #6189, #51178, #139644, #51901, #49044, #72965, #84532, #96081, #60663, #117815, #125889, #26562, #82387, #114950, #4741, #93241, #137474, #38167, #109102, #142475, #54064, #54756, #140319, #11185, #98252, #8336, #64915, #52585, #98936, #32282, #76513, #87376, #110515, #97507, #86669, #129429, #33024, #55466, #130171, #120681, #10498, #85206, #9791, #30866, #143171, #22091, #43164, #21402, #141767, #53296, #108354, #42469, #41006, #20663, #64196, #19254, #9031, #130895, #30117, #118553, #75094, #131591, #31567, #119261, #65666, #109830, #43873, #88088, #19952, #132331, #74365, #75790, #119953, #77241, #121408, #66348, #63510, #107676, #96763, #141015, #41721, #85933, #58365, #14796, #36550, #111237, #114112, #124275, #99651, #101807, #113379, #78638, #69944, #57616, #80785, #22773, #122850, #135188, #67051, #100396, #77933, #2465, #122119, #23530, #102545, #35154, #1734, #35877, #124986, #25666, #67801, #101085, #46028, #322, #91647, #69196, #3196, #88815, #79398, #123599, #11925, #14069, #56213, #44623, #1039, #133043, #56912, #45327, #89503, #80093, #133737, #24254, #33726, #134454, #46774, #90956, #12644, #34413, #68501, #24941, #111992, #90212, #112680, #13348, #47484, #135870, #59068, #126403, #105363, #38700, #127114, #61900, #103225, #6021, #49607, #82927, #93789, #27095, #117642, #114793, #106055, #16944, #29234, #81516, #128561, #71337, #50299, #73476, #61219, #82231, #38005, #6722, #28547, #125723, #16189, #3875, #26403, #48153, #92333, #95205, #51007, #136562, #37273, #27814, #15474, #70649, #94485, #59755, #5326, #103916, #104654, #115491, #60480, #4565, #17627, #138015, #127869, #72806, #48872, #138734, #116960, #139475, #40160, #72081, #93077, #137306, #116254, #39428, #83660, #84372, #54582, #87901, #64022, #51727, #85752, #30692, #32839, #21218, #132145, #143000, #62599, #9601, #87194, #76326, #107510, #31391, #131421, #106785, #120488, #8171, #75613, #32100, #7468, #140161, #64727, #40838, #140836, #65473, #97314, #108191, #53879, #43687, #77060, #41526, #19782, #8851, #18324, #10327, #109653, #98762, #95922, #141585, #42285, #85047, #129251, #74182, #29939, #118376, #19077, #119099, #63339, #52410, #98074, #96596, #86494, #129987, #53113, #20481, #108911, #74921, #130725, #119788, #142309, #42993, #122660, #49248, #4948, #114460, #133565, #121234, #45158, #26048, #100914, #47834, #126082, #21927, #70310, #111806, #3535, #12472, #89333, #38350, #33559, #26748, #81150, #93441, #136, #137676, #34247, #15136, #66173, #125360, #867, #100218, #70998, #92706, #44438, #78469, #110343, #88638, #11020, #55294, #15820, #115147, #99464, #132869, #92000, #77759, #121936 ),
 ( #11741, #23344, #59418, #67617, #103575, #56755, #4212, #48504, #22608, #66877, #111051, #81890, #56027, #60117, #136218, #36903, #136939, #37652, #104283, #52765, #39799, #28899, #71700, #118745, #96956, #72445, #117998, #96252, #27440, #95566, #116613, #140497, #107850, #139830, #18700, #84025, #139096, #50644, #128221, #126756, #106405, #6367, #105013, #94832, #73134, #82566, #60857, #17293, #84703, #117303, #61558, #62979, #40503, #7095, #128909, #105707, #7833, #115867, #17973, #62251, #29589, #51372, #73826, #107154, #52078, #41184, #16566, #8516, #85394, #129618, #141208, #19440, #94133, #5685, #30319, #49950, #74557, #63690, #138370, #39056, #83278, #127488, #28186, #20855, #77432, #108549, #42654, #33906, #54254, #22973, #44064, #143357, #75970, #66532, #120142, #111441, #9988, #131064, #22264, #54948, #110009, #110699, #133230, #65115, #11377, #44821, #75275, #88284, #21593, #98434, #132532, #78126, #12122, #120882, #64378, #142655, #55658, #99859, #67240, #53508, #87559, #33219, #56407, #109305, #43348, #522, #89006, #86856, #121596, #122299, #100588, #131785, #41924, #10674, #86136, #99113, #130364, #31055, #119440, #20137, #97713, #9226, #141967, #31753, #32474, #76713, #65853, #25137, #68684, #23727, #13535, #91153, #1231, #123051, #134656, #3373, #135374, #79595, #125184, #14274, #69392, #102727, #24436, #70139, #34608, #35350, #112871, #91829, #123778, #47668, #36056, #136054, #114300, #45515, #70828, #57815, #103406, #59947, #81712, #12828, #15658, #25867, #89694, #36737, #14974, #102004, #114975, #80976, #125912, #67998, #2667, #59252, #112182, #1922, #136761, #46966, #26584, #4053, #48338, #80278, #92528, #124469, #133920, #113576, #90409, #37478, #58559, #78843, #57101, #101284, #46228, #128747, #106988, #137499, #106251, #83859, #116451, #51206, #51925, #30143, #39632, #126588, #72285, #84554, #29426, #129457, #115688, #6211, #62093, #74394, #83113, #61404, #73666, #117841, #5518, #139667, #95404, #6924, #50488, #18527, #72987, #40346, #17820, #62809, #104109, #118582, #7670, #16389, #28745, #60690, #96105, #140343, #41030, #85234, #19279, #105548, #94674, #93266, #4772, #49073, #93972, #38192, #82406, #27278, #117142, #138206, #71533, #104852, #49796, #38892, #138930, #17138, #128063, #127315, #28017, #120716, #75118, #131622, #119288, #22114, #98958, #143199, #10520, #33751, #20695, #9821, #52611, #99678, #77955, #53323, #43900, #77266, #8359, #76540, #97541, #121436, #88841, #21428, #88113, #64942, #119980, #31593, #109135, #107701, #87404, #130921, #85964, #75816, #54091, #63537, #41749, #141794, #65691, #98278, #42492, #132362, #109854, #32311, #54781, #86696, #33054, #96795, #142503, #43189, #66369, #110540, #11214, #55495, #354, #44650, #141045, #133069, #122139, #130199, #30890, #19974, #64221, #108382, #9063, #37296, #24965, #36569, #1756, #136589, #124299, #3896, #89528, #46057, #58388, #133757, #23558, #14818, #35179, #48172, #69224, #113408, #56936, #47507, #101109, #92360, #134480, #112015, #3215, #35899, #90983, #91668, #114134, #90236, #135891, #25692, #56240, #14091, #2486, #79425, #102571, #59088, #81543, #101833, #45352, #123622, #80817, #125010, #22803, #34439, #68523, #69969, #67077, #24275, #112707, #103248, #111262, #67826, #11954, #100420, #1066, #13369, #78663, #135211, #122871, #80115, #12667, #57646, #46801, #51755, #140181, #18351, #117665, #95946, #70670, #6046, #82250, #4589, #72831, #48897, #72104, #125747, #27838, #49633, #82944, #59776, #84393, #116277, #51030, #95229, #114814, #127892, #139501, #29260, #40184, #105387, #26422, #126425, #93810, #28572, #15496, #138759, #62627, #40866, #16971, #103942, #138037, #38723, #93102, #128584, #137333, #106807, #38026, #116981, #73502, #7497, #71360, #39455, #27116, #115518, #16212, #17652, #60503, #104681, #5349, #61242, #50319, #61924, #127142, #94506, #83684, #106076, #6749, #110372, #77089, #54607, #87928, #74209, #20504, #64759, #8192, #98789, #140862, #55320, #52434, #118402, #42313, #96622, #41559, #21246, #63367, #108941, #85072, #119814, #87224, #131447, #141610, #119125, #9631, #120520, #85782, #86523, #11045, #99493, #76352, #97346, #129277, #8876, #32124, #53909, #98103, #132173, #29966, #65504, #75642, #142334, #43015, #53143, #165, #130012, #32867, #109683, #19101, #107535, #30721, #130749, #10353, #74946, #143028, #108214, #64047, #121265, #43714, #19806, #31420, #21953, #66198, #56783, #44462, #111840, #90810, #24113, #112540, #47348, #88667, #135047, #35007, #68366, #79250, #12502, #103099, #100244, #91516, #2314, #14659, #66900, #113968, #100941, #35741, #58937, #46632, #67647, #23375, #135729, #13915, #111082, #1599, #132901, #11772, #33584, #77783, #80645, #36415, #121965, #22637, #13200, #898, #56056, #79959, #45184, #134309, #89360, #90059, #45884, #123455, #133594, #34272, #78493, #124130, #122690, #24813, #57474, #101656, #69058, #113238, #58215, #102407, #3053, #124842, #25517, #69791, #50153, #137882, #5884, #72662, #48024, #73340, #137160, #105919, #62459, #84231, #15332, #18184, #28399, #3734, #94350, #17500, #126275, #117509, #105230, #128428, #70520, #26951, #39280, #114662, #4415, #139326, #16038, #29102, #138586, #83503, #37861, #116819, #82095, #92195, #115351, #92925, #127717, #16796, #71927, #61754, #95056, #71204, #6583, #50858, #37117, #40015, #126969, #60330, #136424, #81372, #125579, #82783, #26256, #104511, #59619, #103775, #48724, #5169, #49467, #93655, #38555, #27660, #116096, #61073, #118225, #8720, #64588, #76922, #85603, #63890, #87055, #31958, #8035, #142170, #53731, #108761, #52973, #131270, #75474, #9451, #20342, #21065, #106628, #121096, #97933, #18932, #31259, #63199, #65334, #42856, #76187, #120347, #21794, #108052, #97168, #95779, #142860, #7323, #96459, #109515, #10190, #51585, #119643, #140702, #54453, #132000, #98628, #43547 ) ),
 .UNSPECIFIED., .F., .F., .T. ) 
 B_SPLINE_SURFACE_WITH_KNOTS ( ( 2, 2 ),
 ( 3, 2, 2, 2, 2, 2, 2, 2, 2, 2, 2, 2, 2, 2, 2, 2, 2, 2, 2, 2, 2, 2, 2, 2, 2, 2, 2, 2, 2, 2, 2, 2, 2, 2, 2, 2, 2, 2, 2, 2, 2, 2, 2, 2, 2, 2, 2, 2, 2, 2, 2, 2, 2, 2, 2, 2, 2, 2, 2, 2, 2, 2, 2, 2, 2, 2, 2, 2, 2, 2, 2, 2, 2, 2, 2, 2, 2, 2, 2, 2, 2, 2, 2, 2, 2, 2, 2, 2, 2, 2, 2, 2, 2, 2, 2, 2, 2, 2, 2, 2, 2, 2, 2, 2, 2, 2, 2, 2, 2, 2, 2, 2, 2, 2, 2, 2, 2, 2, 2, 2, 2, 2, 2, 2, 2, 2, 2, 2, 2, 2, 2, 2, 2, 2, 2, 2, 2, 2, 2, 2, 2, 2, 2, 2, 2, 2, 2, 2, 2, 2, 2, 2, 2, 2, 2, 2, 2, 2, 2, 2, 2, 2, 2, 2, 2, 2, 2, 2, 2, 2, 2, 2, 2, 2, 2, 2, 2, 2, 2, 2, 2, 2, 2, 2, 2, 2, 2, 2, 2, 2, 2, 2, 2, 2, 2, 2, 2, 2, 2, 2, 2, 2, 2, 2, 2, 2, 2, 2, 2, 2, 2, 2, 2, 2, 2, 2, 2, 2, 2, 2, 2, 2, 2, 2, 2, 2, 2, 2, 2, 2, 2, 2, 2, 2, 2, 2, 2, 2, 2, 2, 2, 2, 2, 2, 2, 2, 2, 2, 2, 2, 2, 2, 2, 2, 2, 2, 2, 2, 2, 2, 2, 2, 2, 2, 2, 2, 2, 2, 2, 2, 2, 2, 2, 2, 2, 2, 2, 2, 2, 2, 2, 2, 2, 2, 2, 2, 2, 2, 2, 2, 2, 2, 2, 2, 2, 2, 2, 2, 2, 2, 2, 2, 2, 2, 2, 2, 2, 2, 2, 2, 2, 2, 2, 2, 2, 2, 2, 2, 2, 2, 2, 2, 2, 2, 2, 2, 2, 2, 2, 2, 2, 2, 2, 2, 2, 2, 2, 2, 2, 2, 2, 2, 2, 2, 2, 2, 2, 2, 2, 2, 2, 3 ),
 ( 0.000000000000000000, 1.000000000000000000 ),
 ( 0.000000000000000000, 0.002777777777777777884, 0.005555555555555555768, 0.008333333333333333218, 0.01111111111111111154, 0.01388888888888888812, 0.01666666666666666644, 0.01944444444444444475, 0.02222222222222222307, 0.02500000000000000139, 0.02777777777777777624, 0.03055555555555555455, 0.03333333333333333287, 0.03611111111111110772, 0.03888888888888888951, 0.04166666666666666435, 0.04444444444444444614, 0.04722222222222222099, 0.05000000000000000278, 0.05277777777777777762, 0.05555555555555555247, 0.05833333333333333426, 0.06111111111111110911, 0.06388888888888888395, 0.06666666666666666574, 0.06944444444444444753, 0.07222222222222221544, 0.07499999999999999722, 0.07777777777777777901, 0.08055555555555556080, 0.08333333333333332871, 0.08611111111111111049, 0.08888888888888889228, 0.09166666666666666019, 0.09444444444444444198, 0.09722222222222222376, 0.1000000000000000056, 0.1027777777777777735, 0.1055555555555555552, 0.1083333333333333370, 0.1111111111111111049, 0.1138888888888888867, 0.1166666666666666685, 0.1194444444444444503, 0.1222222222222222182, 0.1250000000000000000, 0.1277777777777777679, 0.1305555555555555636, 0.1333333333333333315, 0.1361111111111110994, 0.1388888888888888951, 0.1416666666666666630, 0.1444444444444444309, 0.1472222222222222265, 0.1499999999999999944, 0.1527777777777777901, 0.1555555555555555580, 0.1583333333333333259, 0.1611111111111111216, 0.1638888888888888895, 0.1666666666666666574, 0.1694444444444444531, 0.1722222222222222210, 0.1749999999999999889, 0.1777777777777777846, 0.1805555555555555525, 0.1833333333333333204, 0.1861111111111111160, 0.1888888888888888840, 0.1916666666666666796, 0.1944444444444444475, 0.1972222222222222154, 0.2000000000000000111, 0.2027777777777777790, 0.2055555555555555469, 0.2083333333333333426, 0.2111111111111111105, 0.2138888888888888784, 0.2166666666666666741, 0.2194444444444444420, 0.2222222222222222099, 0.2250000000000000056, 0.2277777777777777735, 0.2305555555555555691, 0.2333333333333333370, 0.2361111111111111049, 0.2388888888888889006, 0.2416666666666666685, 0.2444444444444444364, 0.2472222222222222321, 0.2500000000000000000, 0.2527777777777777679, 0.2555555555555555358, 0.2583333333333333592, 0.2611111111111111271, 0.2638888888888888951, 0.2666666666666666630, 0.2694444444444444309, 0.2722222222222221988, 0.2750000000000000222, 0.2777777777777777901, 0.2805555555555555580, 0.2833333333333333259, 0.2861111111111110938, 0.2888888888888888618, 0.2916666666666666852, 0.2944444444444444531, 0.2972222222222222210, 0.2999999999999999889, 0.3027777777777777568, 0.3055555555555555802, 0.3083333333333333481, 0.3111111111111111160, 0.3138888888888888840, 0.3166666666666666519, 0.3194444444444444198, 0.3222222222222222432, 0.3250000000000000111, 0.3277777777777777790, 0.3305555555555555469, 0.3333333333333333148, 0.3361111111111111382, 0.3388888888888889062, 0.3416666666666666741, 0.3444444444444444420, 0.3472222222222222099, 0.3499999999999999778, 0.3527777777777778012, 0.3555555555555555691, 0.3583333333333333370, 0.3611111111111111049, 0.3638888888888888729, 0.3666666666666666408, 0.3694444444444444642, 0.3722222222222222321, 0.3750000000000000000, 0.3777777777777777679, 0.3805555555555555358, 0.3833333333333333592, 0.3861111111111111271, 0.3888888888888888951, 0.3916666666666666630, 0.3944444444444444309, 0.3972222222222221988, 0.4000000000000000222, 0.4027777777777777901, 0.4055555555555555580, 0.4083333333333333259, 0.4111111111111110938, 0.4138888888888888618, 0.4166666666666666852, 0.4194444444444444531, 0.4222222222222222210, 0.4249999999999999889, 0.4277777777777777568, 0.4305555555555555802, 0.4333333333333333481, 0.4361111111111111160, 0.4388888888888888840, 0.4416666666666666519, 0.4444444444444444198, 0.4472222222222222432, 0.4500000000000000111, 0.4527777777777777790, 0.4555555555555555469, 0.4583333333333333148, 0.4611111111111111382, 0.4638888888888889062, 0.4666666666666666741, 0.4694444444444444420, 0.4722222222222222099, 0.4749999999999999778, 0.4777777777777778012, 0.4805555555555555691, 0.4833333333333333370, 0.4861111111111111049, 0.4888888888888888729, 0.4916666666666666408, 0.4944444444444444642, 0.4972222222222222321, 0.5000000000000000000, 0.5027777777777777679, 0.5055555555555555358, 0.5083333333333333037, 0.5111111111111110716, 0.5138888888888888395, 0.5166666666666667185, 0.5194444444444444864, 0.5222222222222222543, 0.5250000000000000222, 0.5277777777777777901, 0.5305555555555555580, 0.5333333333333333259, 0.5361111111111110938, 0.5388888888888888618, 0.5416666666666666297, 0.5444444444444443976, 0.5472222222222222765, 0.5500000000000000444, 0.5527777777777778123, 0.5555555555555555802, 0.5583333333333333481, 0.5611111111111111160, 0.5638888888888888840, 0.5666666666666666519, 0.5694444444444444198, 0.5722222222222221877, 0.5749999999999999556, 0.5777777777777777235, 0.5805555555555556024, 0.5833333333333333703, 0.5861111111111111382, 0.5888888888888889062, 0.5916666666666666741, 0.5944444444444444420, 0.5972222222222222099, 0.5999999999999999778, 0.6027777777777777457, 0.6055555555555555136, 0.6083333333333332815, 0.6111111111111111605, 0.6138888888888889284, 0.6166666666666666963, 0.6194444444444444642, 0.6222222222222222321, 0.6250000000000000000, 0.6277777777777777679, 0.6305555555555555358, 0.6333333333333333037, 0.6361111111111110716, 0.6388888888888888395, 0.6416666666666667185, 0.6444444444444444864, 0.6472222222222222543, 0.6500000000000000222, 0.6527777777777777901, 0.6555555555555555580, 0.6583333333333333259, 0.6611111111111110938, 0.6638888888888888618, 0.6666666666666666297, 0.6694444444444443976, 0.6722222222222222765, 0.6750000000000000444, 0.6777777777777778123, 0.6805555555555555802, 0.6833333333333333481, 0.6861111111111111160, 0.6888888888888888840, 0.6916666666666666519, 0.6944444444444444198, 0.6972222222222221877, 0.6999999999999999556, 0.7027777777777777235, 0.7055555555555556024, 0.7083333333333333703, 0.7111111111111111382, 0.7138888888888889062, 0.7166666666666666741, 0.7194444444444444420, 0.7222222222222222099, 0.7249999999999999778, 0.7277777777777777457, 0.7305555555555555136, 0.7333333333333332815, 0.7361111111111111605, 0.7388888888888889284, 0.7416666666666666963, 0.7444444444444444642, 0.7472222222222222321, 0.7500000000000000000, 0.7527777777777777679, 0.7555555555555555358, 0.7583333333333333037, 0.7611111111111110716, 0.7638888888888888395, 0.7666666666666667185, 0.7694444444444444864, 0.7722222222222222543, 0.7750000000000000222, 0.7777777777777777901, 0.7805555555555555580, 0.7833333333333333259, 0.7861111111111110938, 0.7888888888888888618, 0.7916666666666666297, 0.7944444444444443976, 0.7972222222222222765, 0.8000000000000000444, 0.8027777777777778123, 0.8055555555555555802, 0.8083333333333333481, 0.8111111111111111160, 0.8138888888888888840, 0.8166666666666666519, 0.8194444444444444198, 0.8222222222222221877, 0.8249999999999999556, 0.8277777777777777235, 0.8305555555555556024, 0.8333333333333333703, 0.8361111111111111382, 0.8388888888888889062, 0.8416666666666666741, 0.8444444444444444420, 0.8472222222222222099, 0.8499999999999999778, 0.8527777777777777457, 0.8555555555555555136, 0.8583333333333332815, 0.8611111111111111605, 0.8638888888888889284, 0.8666666666666666963, 0.8694444444444444642, 0.8722222222222222321, 0.8750000000000000000, 0.8777777777777777679, 0.8805555555555555358, 0.8833333333333333037, 0.8861111111111110716, 0.8888888888888888395, 0.8916666666666667185, 0.8944444444444444864, 0.8972222222222222543, 0.9000000000000000222, 0.9027777777777777901, 0.9055555555555555580, 0.9083333333333333259, 0.9111111111111110938, 0.9138888888888888618, 0.9166666666666666297, 0.9194444444444443976, 0.9222222222222222765, 0.9250000000000000444, 0.9277777777777778123, 0.9305555555555555802, 0.9333333333333333481, 0.9361111111111111160, 0.9388888888888888840, 0.9416666666666666519, 0.9444444444444444198, 0.9472222222222221877, 0.9499999999999999556, 0.9527777777777777235, 0.9555555555555556024, 0.9583333333333333703, 0.9611111111111111382, 0.9638888888888889062, 0.9666666666666666741, 0.9694444444444444420, 0.9722222222222222099, 0.9749999999999999778 ),
 .UNSPECIFIED. ) 
 GEOMETRIC_REPRESENTATION_ITEM ( )  RATIONAL_B_SPLINE_SURFACE ( (
 ( 1.000000000000000000, 0.9659258262890683122, 1.000000000000000000, 0.9659258262890683122, 1.000000000000000000, 0.9659258262890683122, 1.000000000000000000, 0.9659258262890683122, 1.000000000000000000, 0.9659258262890683122, 1.000000000000000000, 0.9659258262890683122, 1.000000000000000000, 0.9659258262890683122, 1.000000000000000000, 0.9659258262890683122, 1.000000000000000000, 0.9659258262890683122, 1.000000000000000000, 0.9659258262890683122, 1.000000000000000000, 0.9659258262890683122, 1.000000000000000000, 0.9659258262890683122, 1.000000000000000000, 0.9659258262890683122, 1.000000000000000000, 0.9659258262890683122, 1.000000000000000000, 0.9659258262890683122, 1.000000000000000000, 0.9659258262890683122, 1.000000000000000000, 0.9659258262890683122, 1.000000000000000000, 0.9659258262890683122, 1.000000000000000000, 0.9659258262890683122, 1.000000000000000000, 0.9659258262890683122, 1.000000000000000000, 0.9659258262890683122, 1.000000000000000000, 0.9659258262890683122, 1.000000000000000000, 0.9659258262890683122, 1.000000000000000000, 0.9659258262890683122, 1.000000000000000000, 0.9659258262890683122, 1.000000000000000000, 0.9659258262890683122, 1.000000000000000000, 0.9659258262890683122, 1.000000000000000000, 0.9659258262890683122, 1.000000000000000000, 0.9659258262890683122, 1.000000000000000000, 0.9659258262890683122, 1.000000000000000000, 0.9659258262890683122, 1.000000000000000000, 0.9659258262890683122, 1.000000000000000000, 0.9659258262890683122, 1.000000000000000000, 0.9659258262890683122, 1.000000000000000000, 0.9659258262890683122, 1.000000000000000000, 0.9659258262890683122, 1.000000000000000000, 0.9659258262890683122, 1.000000000000000000, 0.9659258262890683122, 1.000000000000000000, 0.9659258262890683122, 1.000000000000000000, 0.9659258262890683122, 1.000000000000000000, 0.9659258262890683122, 1.000000000000000000, 0.9659258262890683122, 1.000000000000000000, 0.9659258262890683122, 1.000000000000000000, 0.9659258262890683122, 1.000000000000000000, 0.9659258262890683122, 1.000000000000000000, 0.9659258262890683122, 1.000000000000000000, 0.9659258262890683122, 1.000000000000000000, 0.9659258262890683122, 1.000000000000000000, 0.9659258262890683122, 1.000000000000000000, 0.9659258262890683122, 1.000000000000000000, 0.9659258262890683122, 1.000000000000000000, 0.9659258262890683122, 1.000000000000000000, 0.9659258262890683122, 1.000000000000000000, 0.9659258262890683122, 1.000000000000000000, 0.9659258262890683122, 1.000000000000000000, 0.9659258262890683122, 1.000000000000000000, 0.9659258262890683122, 1.000000000000000000, 0.9659258262890683122, 1.000000000000000000, 0.9659258262890683122, 1.000000000000000000, 0.9659258262890683122, 1.000000000000000000, 0.9659258262890683122, 1.000000000000000000, 0.9659258262890683122, 1.000000000000000000, 0.9659258262890683122, 1.000000000000000000, 0.9659258262890683122, 1.000000000000000000, 0.9659258262890683122, 1.000000000000000000, 0.9659258262890683122, 1.000000000000000000, 0.9659258262890683122, 1.000000000000000000, 0.9659258262890683122, 1.000000000000000000, 0.9659258262890683122, 1.000000000000000000, 0.9659258262890683122, 1.000000000000000000, 0.9659258262890683122, 1.000000000000000000, 0.9659258262890683122, 1.000000000000000000, 0.9659258262890683122, 1.000000000000000000, 0.9659258262890683122, 1.000000000000000000, 0.9659258262890683122, 1.000000000000000000, 0.9659258262890683122, 1.000000000000000000, 0.9659258262890683122, 1.000000000000000000, 0.9659258262890683122, 1.000000000000000000, 0.9659258262890683122, 1.000000000000000000, 0.9659258262890683122, 1.000000000000000000, 0.9659258262890683122, 1.000000000000000000, 0.9659258262890683122, 1.000000000000000000, 0.9659258262890683122, 1.000000000000000000, 0.9659258262890683122, 1.000000000000000000, 0.9659258262890683122, 1.000000000000000000, 0.9659258262890683122, 1.000000000000000000, 0.9659258262890683122, 1.000000000000000000, 0.9659258262890683122, 1.000000000000000000, 0.9659258262890683122, 1.000000000000000000, 0.9659258262890683122, 1.000000000000000000, 0.9659258262890683122, 1.000000000000000000, 0.9659258262890683122, 1.000000000000000000, 0.9659258262890683122, 1.000000000000000000, 0.9659258262890683122, 1.000000000000000000, 0.9659258262890683122, 1.000000000000000000, 0.9659258262890683122, 1.000000000000000000, 0.9659258262890683122, 1.000000000000000000, 0.9659258262890683122, 1.000000000000000000, 0.9659258262890683122, 1.000000000000000000, 0.9659258262890683122, 1.000000000000000000, 0.9659258262890683122, 1.000000000000000000, 0.9659258262890683122, 1.000000000000000000, 0.9659258262890683122, 1.000000000000000000, 0.9659258262890683122, 1.000000000000000000, 0.9659258262890683122, 1.000000000000000000, 0.9659258262890683122, 1.000000000000000000, 0.9659258262890683122, 1.000000000000000000, 0.9659258262890683122, 1.000000000000000000, 0.9659258262890683122, 1.000000000000000000, 0.9659258262890683122, 1.000000000000000000, 0.9659258262890683122, 1.000000000000000000, 0.9659258262890683122, 1.000000000000000000, 0.9659258262890683122, 1.000000000000000000, 0.9659258262890683122, 1.000000000000000000, 0.9659258262890683122, 1.000000000000000000, 0.9659258262890683122, 1.000000000000000000, 0.9659258262890683122, 1.000000000000000000, 0.9659258262890683122, 1.000000000000000000, 0.9659258262890683122, 1.000000000000000000, 0.9659258262890683122, 1.000000000000000000, 0.9659258262890683122, 1.000000000000000000, 0.9659258262890683122, 1.000000000000000000, 0.9659258262890683122, 1.000000000000000000, 0.9659258262890683122, 1.000000000000000000, 0.9659258262890683122, 1.000000000000000000, 0.9659258262890683122, 1.000000000000000000, 0.9659258262890683122, 1.000000000000000000, 0.9659258262890683122, 1.000000000000000000, 0.9659258262890683122, 1.000000000000000000, 0.9659258262890683122, 1.000000000000000000, 0.9659258262890683122, 1.000000000000000000, 0.9659258262890683122, 1.000000000000000000, 0.9659258262890683122, 1.000000000000000000, 0.9659258262890683122, 1.000000000000000000, 0.9659258262890683122, 1.000000000000000000, 0.9659258262890683122, 1.000000000000000000, 0.9659258262890683122, 1.000000000000000000, 0.9659258262890683122, 1.000000000000000000, 0.9659258262890683122, 1.000000000000000000, 0.9659258262890683122, 1.000000000000000000, 0.9659258262890683122, 1.000000000000000000, 0.9659258262890683122, 1.000000000000000000, 0.9659258262890683122, 1.000000000000000000, 0.9659258262890683122, 1.000000000000000000, 0.9659258262890683122, 1.000000000000000000, 0.9659258262890683122, 1.000000000000000000, 0.9659258262890683122, 1.000000000000000000, 0.9659258262890683122, 1.000000000000000000, 0.9659258262890683122, 1.000000000000000000, 0.9659258262890683122, 1.000000000000000000, 0.9659258262890683122, 1.000000000000000000, 0.9659258262890683122, 1.000000000000000000, 0.9659258262890683122, 1.000000000000000000, 0.9659258262890683122, 1.000000000000000000, 0.9659258262890683122, 1.000000000000000000, 0.9659258262890683122, 1.000000000000000000, 0.9659258262890683122, 1.000000000000000000, 0.9659258262890683122, 1.000000000000000000, 0.9659258262890683122, 1.000000000000000000, 0.9659258262890683122, 1.000000000000000000, 0.9659258262890683122, 1.000000000000000000, 0.9659258262890683122, 1.000000000000000000, 0.9659258262890683122, 1.000000000000000000, 0.9659258262890683122, 1.000000000000000000, 0.9659258262890683122, 1.000000000000000000, 0.9659258262890683122, 1.000000000000000000, 0.9659258262890683122, 1.000000000000000000, 0.9659258262890683122, 1.000000000000000000, 0.9659258262890683122, 1.000000000000000000, 0.9659258262890683122, 1.000000000000000000, 0.9659258262890683122, 1.000000000000000000, 0.9659258262890683122, 1.000000000000000000, 0.9659258262890683122, 1.000000000000000000, 0.9659258262890683122, 1.000000000000000000, 0.9659258262890683122, 1.000000000000000000, 0.9659258262890683122, 1.000000000000000000, 0.9659258262890683122, 1.000000000000000000, 0.9659258262890683122, 1.000000000000000000, 0.9659258262890683122, 1.000000000000000000, 0.9659258262890683122, 1.000000000000000000, 0.9659258262890683122, 1.000000000000000000, 0.9659258262890683122, 1.000000000000000000, 0.9659258262890683122, 1.000000000000000000, 0.9659258262890683122, 1.000000000000000000, 0.9659258262890683122, 1.000000000000000000, 0.9659258262890683122, 1.000000000000000000, 0.9659258262890683122, 1.000000000000000000, 0.9659258262890683122, 1.000000000000000000, 0.9659258262890683122, 1.000000000000000000, 0.9659258262890683122, 1.000000000000000000, 0.9659258262890683122, 1.000000000000000000, 0.9659258262890683122, 1.000000000000000000, 0.9659258262890683122, 1.000000000000000000, 0.9659258262890683122, 1.000000000000000000, 0.9659258262890683122, 1.000000000000000000, 0.9659258262890683122, 1.000000000000000000, 0.9659258262890683122, 1.000000000000000000, 0.9659258262890683122, 1.000000000000000000, 0.9659258262890683122, 1.000000000000000000, 0.9659258262890683122, 1.000000000000000000, 0.9659258262890683122, 1.000000000000000000, 0.9659258262890683122, 1.000000000000000000, 0.9659258262890683122, 1.000000000000000000, 0.9659258262890683122, 1.000000000000000000, 0.9659258262890683122, 1.000000000000000000, 0.9659258262890683122, 1.000000000000000000, 0.9659258262890683122, 1.000000000000000000, 0.9659258262890683122, 1.000000000000000000, 0.9659258262890683122, 1.000000000000000000, 0.9659258262890683122, 1.000000000000000000, 0.9659258262890683122, 1.000000000000000000, 0.9659258262890683122, 1.000000000000000000, 0.9659258262890683122, 1.000000000000000000, 0.9659258262890683122, 1.000000000000000000, 0.9659258262890683122, 1.000000000000000000, 0.9659258262890683122, 1.000000000000000000, 0.9659258262890683122, 1.000000000000000000, 0.9659258262890683122, 1.000000000000000000, 0.9659258262890683122, 1.000000000000000000, 0.9659258262890683122, 1.000000000000000000, 0.9659258262890683122, 1.000000000000000000, 0.9659258262890683122, 1.000000000000000000, 0.9659258262890683122, 1.000000000000000000, 0.9659258262890683122, 1.000000000000000000, 0.9659258262890683122, 1.000000000000000000, 0.9659258262890683122, 1.000000000000000000, 0.9659258262890683122, 1.000000000000000000, 0.9659258262890683122, 1.000000000000000000, 0.9659258262890683122, 1.000000000000000000, 0.9659258262890683122, 1.000000000000000000, 0.9659258262890683122, 1.000000000000000000, 0.9659258262890683122, 1.000000000000000000, 0.9659258262890683122, 1.000000000000000000, 0.9659258262890683122, 1.000000000000000000, 0.9659258262890683122, 1.000000000000000000, 0.9659258262890683122, 1.000000000000000000, 0.9659258262890683122, 1.000000000000000000, 0.9659258262890683122, 1.000000000000000000, 0.9659258262890683122, 1.000000000000000000, 0.9659258262890683122, 1.000000000000000000, 0.9659258262890683122, 1.000000000000000000, 0.9659258262890683122, 1.000000000000000000, 0.9659258262890683122, 1.000000000000000000, 0.9659258262890683122, 1.000000000000000000, 0.9659258262890683122, 1.000000000000000000, 0.9659258262890683122, 1.000000000000000000, 0.9659258262890683122, 1.000000000000000000, 0.9659258262890683122, 1.000000000000000000, 0.9659258262890683122, 1.000000000000000000, 0.9659258262890683122, 1.000000000000000000, 0.9659258262890683122, 1.000000000000000000, 0.9659258262890683122, 1.000000000000000000, 0.9659258262890683122, 1.000000000000000000, 0.9659258262890683122, 1.000000000000000000, 0.9659258262890683122, 1.000000000000000000, 0.9659258262890683122, 1.000000000000000000, 0.9659258262890683122, 1.000000000000000000, 0.9659258262890683122, 1.000000000000000000, 0.9659258262890683122, 1.000000000000000000, 0.9659258262890683122, 1.000000000000000000, 0.9659258262890683122, 1.000000000000000000, 0.9659258262890683122, 1.000000000000000000, 0.9659258262890683122, 1.000000000000000000, 0.9659258262890683122, 1.000000000000000000, 0.9659258262890683122, 1.000000000000000000, 0.9659258262890683122, 1.000000000000000000, 0.9659258262890683122, 1.000000000000000000, 0.9659258262890683122, 1.000000000000000000, 0.9659258262890683122, 1.000000000000000000, 0.9659258262890683122, 1.000000000000000000, 0.9659258262890683122, 1.000000000000000000, 0.9659258262890683122, 1.000000000000000000, 0.9659258262890683122, 1.000000000000000000, 0.9659258262890683122, 1.000000000000000000, 0.9659258262890683122, 1.000000000000000000, 0.9659258262890683122, 1.000000000000000000, 0.9659258262890683122, 1.000000000000000000, 0.9659258262890683122, 1.000000000000000000, 0.9659258262890683122, 1.000000000000000000, 0.9659258262890683122, 1.000000000000000000, 0.9659258262890683122, 1.000000000000000000, 0.9659258262890683122, 1.000000000000000000, 0.9659258262890683122, 1.000000000000000000, 0.9659258262890683122, 1.000000000000000000, 0.9659258262890683122, 1.000000000000000000, 0.9659258262890683122, 1.000000000000000000, 0.9659258262890683122, 1.000000000000000000, 0.9659258262890683122, 1.000000000000000000, 0.9659258262890683122, 1.000000000000000000, 0.9659258262890683122, 1.000000000000000000, 0.9659258262890683122, 1.000000000000000000, 0.9659258262890683122, 1.000000000000000000, 0.9659258262890683122, 1.000000000000000000, 0.9659258262890683122, 1.000000000000000000, 0.9659258262890683122, 1.000000000000000000, 0.9659258262890683122, 1.000000000000000000, 0.9659258262890683122, 1.000000000000000000, 0.9659258262890683122, 1.000000000000000000, 0.9659258262890683122, 1.000000000000000000, 0.9659258262890683122, 1.000000000000000000, 0.9659258262890683122, 1.000000000000000000, 0.9659258262890683122, 1.000000000000000000, 0.9659258262890683122, 1.000000000000000000, 0.9659258262890683122, 1.000000000000000000, 0.9659258262890683122, 1.000000000000000000, 0.9659258262890683122, 1.000000000000000000, 0.9659258262890683122, 1.000000000000000000, 0.9659258262890683122, 1.000000000000000000, 0.9659258262890683122, 1.000000000000000000, 0.9659258262890683122, 1.000000000000000000, 0.9659258262890683122, 1.000000000000000000, 0.9659258262890683122, 1.000000000000000000, 0.9659258262890683122, 1.000000000000000000, 0.9659258262890683122, 1.000000000000000000, 0.9659258262890683122, 1.000000000000000000, 0.9659258262890683122, 1.000000000000000000, 0.9659258262890683122, 1.000000000000000000, 0.9659258262890683122, 1.000000000000000000, 0.9659258262890683122, 1.000000000000000000, 0.9659258262890683122, 1.000000000000000000, 0.9659258262890683122, 1.000000000000000000, 0.9659258262890683122, 1.000000000000000000, 0.9659258262890683122, 1.000000000000000000, 0.9659258262890683122, 1.000000000000000000, 0.9659258262890683122, 1.000000000000000000, 0.9659258262890683122, 1.000000000000000000, 0.9659258262890683122, 1.000000000000000000, 0.9659258262890683122, 1.000000000000000000, 0.9659258262890683122, 1.000000000000000000, 0.9659258262890683122, 1.000000000000000000, 0.9659258262890683122, 1.000000000000000000, 0.9659258262890683122, 1.000000000000000000, 0.9659258262890683122, 1.000000000000000000, 0.9659258262890683122, 1.000000000000000000, 0.9659258262890683122, 1.000000000000000000, 0.9659258262890683122, 1.000000000000000000, 0.9659258262890683122, 1.000000000000000000, 0.9659258262890683122, 1.000000000000000000, 0.9659258262890683122, 1.000000000000000000, 0.9659258262890683122, 1.000000000000000000, 0.9659258262890683122, 1.000000000000000000, 0.9659258262890683122, 1.000000000000000000, 0.9659258262890683122, 1.000000000000000000, 0.9659258262890683122, 1.000000000000000000, 0.9659258262890683122, 1.000000000000000000, 0.9659258262890683122, 1.000000000000000000, 0.9659258262890683122, 1.000000000000000000, 0.9659258262890683122, 1.000000000000000000, 0.9659258262890683122, 1.000000000000000000, 0.9659258262890683122, 1.000000000000000000, 0.9659258262890683122, 1.000000000000000000),
 ( 1.000000000000000000, 0.9659258262890683122, 1.000000000000000000, 0.9659258262890683122, 1.000000000000000000, 0.9659258262890683122, 1.000000000000000000, 0.9659258262890683122, 1.000000000000000000, 0.9659258262890683122, 1.000000000000000000, 0.9659258262890683122, 1.000000000000000000, 0.9659258262890683122, 1.000000000000000000, 0.9659258262890683122, 1.000000000000000000, 0.9659258262890683122, 1.000000000000000000, 0.9659258262890683122, 1.000000000000000000, 0.9659258262890683122, 1.000000000000000000, 0.9659258262890683122, 1.000000000000000000, 0.9659258262890683122, 1.000000000000000000, 0.9659258262890683122, 1.000000000000000000, 0.9659258262890683122, 1.000000000000000000, 0.9659258262890683122, 1.000000000000000000, 0.9659258262890683122, 1.000000000000000000, 0.9659258262890683122, 1.000000000000000000, 0.9659258262890683122, 1.000000000000000000, 0.9659258262890683122, 1.000000000000000000, 0.9659258262890683122, 1.000000000000000000, 0.9659258262890683122, 1.000000000000000000, 0.9659258262890683122, 1.000000000000000000, 0.9659258262890683122, 1.000000000000000000, 0.9659258262890683122, 1.000000000000000000, 0.9659258262890683122, 1.000000000000000000, 0.9659258262890683122, 1.000000000000000000, 0.9659258262890683122, 1.000000000000000000, 0.9659258262890683122, 1.000000000000000000, 0.9659258262890683122, 1.000000000000000000, 0.9659258262890683122, 1.000000000000000000, 0.9659258262890683122, 1.000000000000000000, 0.9659258262890683122, 1.000000000000000000, 0.9659258262890683122, 1.000000000000000000, 0.9659258262890683122, 1.000000000000000000, 0.9659258262890683122, 1.000000000000000000, 0.9659258262890683122, 1.000000000000000000, 0.9659258262890683122, 1.000000000000000000, 0.9659258262890683122, 1.000000000000000000, 0.9659258262890683122, 1.000000000000000000, 0.9659258262890683122, 1.000000000000000000, 0.9659258262890683122, 1.000000000000000000, 0.9659258262890683122, 1.000000000000000000, 0.9659258262890683122, 1.000000000000000000, 0.9659258262890683122, 1.000000000000000000, 0.9659258262890683122, 1.000000000000000000, 0.9659258262890683122, 1.000000000000000000, 0.9659258262890683122, 1.000000000000000000, 0.9659258262890683122, 1.000000000000000000, 0.9659258262890683122, 1.000000000000000000, 0.9659258262890683122, 1.000000000000000000, 0.9659258262890683122, 1.000000000000000000, 0.9659258262890683122, 1.000000000000000000, 0.9659258262890683122, 1.000000000000000000, 0.9659258262890683122, 1.000000000000000000, 0.9659258262890683122, 1.000000000000000000, 0.9659258262890683122, 1.000000000000000000, 0.9659258262890683122, 1.000000000000000000, 0.9659258262890683122, 1.000000000000000000, 0.9659258262890683122, 1.000000000000000000, 0.9659258262890683122, 1.000000000000000000, 0.9659258262890683122, 1.000000000000000000, 0.9659258262890683122, 1.000000000000000000, 0.9659258262890683122, 1.000000000000000000, 0.9659258262890683122, 1.000000000000000000, 0.9659258262890683122, 1.000000000000000000, 0.9659258262890683122, 1.000000000000000000, 0.9659258262890683122, 1.000000000000000000, 0.9659258262890683122, 1.000000000000000000, 0.9659258262890683122, 1.000000000000000000, 0.9659258262890683122, 1.000000000000000000, 0.9659258262890683122, 1.000000000000000000, 0.9659258262890683122, 1.000000000000000000, 0.9659258262890683122, 1.000000000000000000, 0.9659258262890683122, 1.000000000000000000, 0.9659258262890683122, 1.000000000000000000, 0.9659258262890683122, 1.000000000000000000, 0.9659258262890683122, 1.000000000000000000, 0.9659258262890683122, 1.000000000000000000, 0.9659258262890683122, 1.000000000000000000, 0.9659258262890683122, 1.000000000000000000, 0.9659258262890683122, 1.000000000000000000, 0.9659258262890683122, 1.000000000000000000, 0.9659258262890683122, 1.000000000000000000, 0.9659258262890683122, 1.000000000000000000, 0.9659258262890683122, 1.000000000000000000, 0.9659258262890683122, 1.000000000000000000, 0.9659258262890683122, 1.000000000000000000, 0.9659258262890683122, 1.000000000000000000, 0.9659258262890683122, 1.000000000000000000, 0.9659258262890683122, 1.000000000000000000, 0.9659258262890683122, 1.000000000000000000, 0.9659258262890683122, 1.000000000000000000, 0.9659258262890683122, 1.000000000000000000, 0.9659258262890683122, 1.000000000000000000, 0.9659258262890683122, 1.000000000000000000, 0.9659258262890683122, 1.000000000000000000, 0.9659258262890683122, 1.000000000000000000, 0.9659258262890683122, 1.000000000000000000, 0.9659258262890683122, 1.000000000000000000, 0.9659258262890683122, 1.000000000000000000, 0.9659258262890683122, 1.000000000000000000, 0.9659258262890683122, 1.000000000000000000, 0.9659258262890683122, 1.000000000000000000, 0.9659258262890683122, 1.000000000000000000, 0.9659258262890683122, 1.000000000000000000, 0.9659258262890683122, 1.000000000000000000, 0.9659258262890683122, 1.000000000000000000, 0.9659258262890683122, 1.000000000000000000, 0.9659258262890683122, 1.000000000000000000, 0.9659258262890683122, 1.000000000000000000, 0.9659258262890683122, 1.000000000000000000, 0.9659258262890683122, 1.000000000000000000, 0.9659258262890683122, 1.000000000000000000, 0.9659258262890683122, 1.000000000000000000, 0.9659258262890683122, 1.000000000000000000, 0.9659258262890683122, 1.000000000000000000, 0.9659258262890683122, 1.000000000000000000, 0.9659258262890683122, 1.000000000000000000, 0.9659258262890683122, 1.000000000000000000, 0.9659258262890683122, 1.000000000000000000, 0.9659258262890683122, 1.000000000000000000, 0.9659258262890683122, 1.000000000000000000, 0.9659258262890683122, 1.000000000000000000, 0.9659258262890683122, 1.000000000000000000, 0.9659258262890683122, 1.000000000000000000, 0.9659258262890683122, 1.000000000000000000, 0.9659258262890683122, 1.000000000000000000, 0.9659258262890683122, 1.000000000000000000, 0.9659258262890683122, 1.000000000000000000, 0.9659258262890683122, 1.000000000000000000, 0.9659258262890683122, 1.000000000000000000, 0.9659258262890683122, 1.000000000000000000, 0.9659258262890683122, 1.000000000000000000, 0.9659258262890683122, 1.000000000000000000, 0.9659258262890683122, 1.000000000000000000, 0.9659258262890683122, 1.000000000000000000, 0.9659258262890683122, 1.000000000000000000, 0.9659258262890683122, 1.000000000000000000, 0.9659258262890683122, 1.000000000000000000, 0.9659258262890683122, 1.000000000000000000, 0.9659258262890683122, 1.000000000000000000, 0.9659258262890683122, 1.000000000000000000, 0.9659258262890683122, 1.000000000000000000, 0.9659258262890683122, 1.000000000000000000, 0.9659258262890683122, 1.000000000000000000, 0.9659258262890683122, 1.000000000000000000, 0.9659258262890683122, 1.000000000000000000, 0.9659258262890683122, 1.000000000000000000, 0.9659258262890683122, 1.000000000000000000, 0.9659258262890683122, 1.000000000000000000, 0.9659258262890683122, 1.000000000000000000, 0.9659258262890683122, 1.000000000000000000, 0.9659258262890683122, 1.000000000000000000, 0.9659258262890683122, 1.000000000000000000, 0.9659258262890683122, 1.000000000000000000, 0.9659258262890683122, 1.000000000000000000, 0.9659258262890683122, 1.000000000000000000, 0.9659258262890683122, 1.000000000000000000, 0.9659258262890683122, 1.000000000000000000, 0.9659258262890683122, 1.000000000000000000, 0.9659258262890683122, 1.000000000000000000, 0.9659258262890683122, 1.000000000000000000, 0.9659258262890683122, 1.000000000000000000, 0.9659258262890683122, 1.000000000000000000, 0.9659258262890683122, 1.000000000000000000, 0.9659258262890683122, 1.000000000000000000, 0.9659258262890683122, 1.000000000000000000, 0.9659258262890683122, 1.000000000000000000, 0.9659258262890683122, 1.000000000000000000, 0.9659258262890683122, 1.000000000000000000, 0.9659258262890683122, 1.000000000000000000, 0.9659258262890683122, 1.000000000000000000, 0.9659258262890683122, 1.000000000000000000, 0.9659258262890683122, 1.000000000000000000, 0.9659258262890683122, 1.000000000000000000, 0.9659258262890683122, 1.000000000000000000, 0.9659258262890683122, 1.000000000000000000, 0.9659258262890683122, 1.000000000000000000, 0.9659258262890683122, 1.000000000000000000, 0.9659258262890683122, 1.000000000000000000, 0.9659258262890683122, 1.000000000000000000, 0.9659258262890683122, 1.000000000000000000, 0.9659258262890683122, 1.000000000000000000, 0.9659258262890683122, 1.000000000000000000, 0.9659258262890683122, 1.000000000000000000, 0.9659258262890683122, 1.000000000000000000, 0.9659258262890683122, 1.000000000000000000, 0.9659258262890683122, 1.000000000000000000, 0.9659258262890683122, 1.000000000000000000, 0.9659258262890683122, 1.000000000000000000, 0.9659258262890683122, 1.000000000000000000, 0.9659258262890683122, 1.000000000000000000, 0.9659258262890683122, 1.000000000000000000, 0.9659258262890683122, 1.000000000000000000, 0.9659258262890683122, 1.000000000000000000, 0.9659258262890683122, 1.000000000000000000, 0.9659258262890683122, 1.000000000000000000, 0.9659258262890683122, 1.000000000000000000, 0.9659258262890683122, 1.000000000000000000, 0.9659258262890683122, 1.000000000000000000, 0.9659258262890683122, 1.000000000000000000, 0.9659258262890683122, 1.000000000000000000, 0.9659258262890683122, 1.000000000000000000, 0.9659258262890683122, 1.000000000000000000, 0.9659258262890683122, 1.000000000000000000, 0.9659258262890683122, 1.000000000000000000, 0.9659258262890683122, 1.000000000000000000, 0.9659258262890683122, 1.000000000000000000, 0.9659258262890683122, 1.000000000000000000, 0.9659258262890683122, 1.000000000000000000, 0.9659258262890683122, 1.000000000000000000, 0.9659258262890683122, 1.000000000000000000, 0.9659258262890683122, 1.000000000000000000, 0.9659258262890683122, 1.000000000000000000, 0.9659258262890683122, 1.000000000000000000, 0.9659258262890683122, 1.000000000000000000, 0.9659258262890683122, 1.000000000000000000, 0.9659258262890683122, 1.000000000000000000, 0.9659258262890683122, 1.000000000000000000, 0.9659258262890683122, 1.000000000000000000, 0.9659258262890683122, 1.000000000000000000, 0.9659258262890683122, 1.000000000000000000, 0.9659258262890683122, 1.000000000000000000, 0.9659258262890683122, 1.000000000000000000, 0.9659258262890683122, 1.000000000000000000, 0.9659258262890683122, 1.000000000000000000, 0.9659258262890683122, 1.000000000000000000, 0.9659258262890683122, 1.000000000000000000, 0.9659258262890683122, 1.000000000000000000, 0.9659258262890683122, 1.000000000000000000, 0.9659258262890683122, 1.000000000000000000, 0.9659258262890683122, 1.000000000000000000, 0.9659258262890683122, 1.000000000000000000, 0.9659258262890683122, 1.000000000000000000, 0.9659258262890683122, 1.000000000000000000, 0.9659258262890683122, 1.000000000000000000, 0.9659258262890683122, 1.000000000000000000, 0.9659258262890683122, 1.000000000000000000, 0.9659258262890683122, 1.000000000000000000, 0.9659258262890683122, 1.000000000000000000, 0.9659258262890683122, 1.000000000000000000, 0.9659258262890683122, 1.000000000000000000, 0.9659258262890683122, 1.000000000000000000, 0.9659258262890683122, 1.000000000000000000, 0.9659258262890683122, 1.000000000000000000, 0.9659258262890683122, 1.000000000000000000, 0.9659258262890683122, 1.000000000000000000, 0.9659258262890683122, 1.000000000000000000, 0.9659258262890683122, 1.000000000000000000, 0.9659258262890683122, 1.000000000000000000, 0.9659258262890683122, 1.000000000000000000, 0.9659258262890683122, 1.000000000000000000, 0.9659258262890683122, 1.000000000000000000, 0.9659258262890683122, 1.000000000000000000, 0.9659258262890683122, 1.000000000000000000, 0.9659258262890683122, 1.000000000000000000, 0.9659258262890683122, 1.000000000000000000, 0.9659258262890683122, 1.000000000000000000, 0.9659258262890683122, 1.000000000000000000, 0.9659258262890683122, 1.000000000000000000, 0.9659258262890683122, 1.000000000000000000, 0.9659258262890683122, 1.000000000000000000, 0.9659258262890683122, 1.000000000000000000, 0.9659258262890683122, 1.000000000000000000, 0.9659258262890683122, 1.000000000000000000, 0.9659258262890683122, 1.000000000000000000, 0.9659258262890683122, 1.000000000000000000, 0.9659258262890683122, 1.000000000000000000, 0.9659258262890683122, 1.000000000000000000, 0.9659258262890683122, 1.000000000000000000, 0.9659258262890683122, 1.000000000000000000, 0.9659258262890683122, 1.000000000000000000, 0.9659258262890683122, 1.000000000000000000, 0.9659258262890683122, 1.000000000000000000, 0.9659258262890683122, 1.000000000000000000, 0.9659258262890683122, 1.000000000000000000, 0.9659258262890683122, 1.000000000000000000, 0.9659258262890683122, 1.000000000000000000, 0.9659258262890683122, 1.000000000000000000, 0.9659258262890683122, 1.000000000000000000, 0.9659258262890683122, 1.000000000000000000, 0.9659258262890683122, 1.000000000000000000, 0.9659258262890683122, 1.000000000000000000, 0.9659258262890683122, 1.000000000000000000, 0.9659258262890683122, 1.000000000000000000, 0.9659258262890683122, 1.000000000000000000, 0.9659258262890683122, 1.000000000000000000, 0.9659258262890683122, 1.000000000000000000, 0.9659258262890683122, 1.000000000000000000, 0.9659258262890683122, 1.000000000000000000, 0.9659258262890683122, 1.000000000000000000, 0.9659258262890683122, 1.000000000000000000, 0.9659258262890683122, 1.000000000000000000, 0.9659258262890683122, 1.000000000000000000, 0.9659258262890683122, 1.000000000000000000, 0.9659258262890683122, 1.000000000000000000, 0.9659258262890683122, 1.000000000000000000, 0.9659258262890683122, 1.000000000000000000, 0.9659258262890683122, 1.000000000000000000, 0.9659258262890683122, 1.000000000000000000, 0.9659258262890683122, 1.000000000000000000, 0.9659258262890683122, 1.000000000000000000, 0.9659258262890683122, 1.000000000000000000, 0.9659258262890683122, 1.000000000000000000, 0.9659258262890683122, 1.000000000000000000, 0.9659258262890683122, 1.000000000000000000, 0.9659258262890683122, 1.000000000000000000, 0.9659258262890683122, 1.000000000000000000, 0.9659258262890683122, 1.000000000000000000, 0.9659258262890683122, 1.000000000000000000, 0.9659258262890683122, 1.000000000000000000, 0.9659258262890683122, 1.000000000000000000, 0.9659258262890683122, 1.000000000000000000, 0.9659258262890683122, 1.000000000000000000, 0.9659258262890683122, 1.000000000000000000, 0.9659258262890683122, 1.000000000000000000, 0.9659258262890683122, 1.000000000000000000, 0.9659258262890683122, 1.000000000000000000, 0.9659258262890683122, 1.000000000000000000, 0.9659258262890683122, 1.000000000000000000, 0.9659258262890683122, 1.000000000000000000, 0.9659258262890683122, 1.000000000000000000, 0.9659258262890683122, 1.000000000000000000, 0.9659258262890683122, 1.000000000000000000, 0.9659258262890683122, 1.000000000000000000, 0.9659258262890683122, 1.000000000000000000, 0.9659258262890683122, 1.000000000000000000, 0.9659258262890683122, 1.000000000000000000, 0.9659258262890683122, 1.000000000000000000, 0.9659258262890683122, 1.000000000000000000, 0.9659258262890683122, 1.000000000000000000, 0.9659258262890683122, 1.000000000000000000, 0.9659258262890683122, 1.000000000000000000, 0.9659258262890683122, 1.000000000000000000, 0.9659258262890683122, 1.000000000000000000, 0.9659258262890683122, 1.000000000000000000, 0.9659258262890683122, 1.000000000000000000, 0.9659258262890683122, 1.000000000000000000, 0.9659258262890683122, 1.000000000000000000, 0.9659258262890683122, 1.000000000000000000, 0.9659258262890683122, 1.000000000000000000, 0.9659258262890683122, 1.000000000000000000, 0.9659258262890683122, 1.000000000000000000, 0.9659258262890683122, 1.000000000000000000, 0.9659258262890683122, 1.000000000000000000, 0.9659258262890683122, 1.000000000000000000, 0.9659258262890683122, 1.000000000000000000, 0.9659258262890683122, 1.000000000000000000, 0.9659258262890683122, 1.000000000000000000, 0.9659258262890683122, 1.000000000000000000) ) ) 
 REPRESENTATION_ITEM ( '' )  SURFACE ( )  );
#91933=CARTESIAN_POINT ( 'NONE',  ( 122.2087635252314328, -7.482591942790329030E-16, 6.110000000000001208 ) ) ;
#91952=CARTESIAN_POINT ( 'NONE',  ( 113.4374999999999858, 5.819803920172574863, -5.819803920172573086 ) ) ;
#92000=CARTESIAN_POINT ( 'NONE',  ( 26.74543019189810877, -5.291415217122919401, -3.055000000000000604 ) ) ;
#92003=CARTESIAN_POINT ( 'NONE',  ( 48.35002705046287730, -5.819803920172573086, -5.819803920172573086 ) ) ;
#92016=CARTESIAN_POINT ( 'NONE',  ( 91.85416666666668561, -2.130196079827425315, -7.950000000000001066 ) ) ;
#92027=CARTESIAN_POINT ( 'NONE',  ( 126.8792446338207753, 3.521890969138218086, 5.552962617327368733 ) ) ;
#92037=CARTESIAN_POINT ( 'NONE',  ( 115.2087635252314470, -7.482591942790329030E-16, 6.110000000000001208 ) ) ;
#92044=DIRECTION ( 'NONE',  ( -1.000000000000000000, -0.000000000000000000, -0.000000000000000000 ) ) ;
#92045=CARTESIAN_POINT ( 'NONE',  ( 104.6204301918981230, 3.055000000000001936, -5.291415217122916737 ) ) ;
#92088=VERTEX_POINT ( 'NONE', #39515 ) ;
#92089=( BOUNDED_CURVE ( )  B_SPLINE_CURVE ( 2, ( #32443, #44033, #33876, #45485, #13504, #131757, #57073, #101252, #143329, #110670, #100558, #24409, #79563 ),
 .UNSPECIFIED., .F., .T. ) 
 B_SPLINE_CURVE_WITH_KNOTS ( ( 3, 2, 2, 2, 2, 2, 3 ),
 ( 0.6500000000000000222, 0.6527777777777777901, 0.6555555555555555580, 0.6583333333333333259, 0.6611111111111110938, 0.6638888888888888618, 0.6666666666666666297 ),
 .UNSPECIFIED. ) 
 CURVE ( )  GEOMETRIC_REPRESENTATION_ITEM ( )  RATIONAL_B_SPLINE_CURVE ( ( 1.000000000000000000, 0.9659258262890683122, 1.000000000000000000, 0.9659258262890683122, 1.000000000000000000, 0.9659258262890683122, 1.000000000000000000, 0.9659258262890683122, 1.000000000000000000, 0.9659258262890683122, 1.000000000000000000, 0.9659258262890683122, 1.000000000000000000 ) ) 
 REPRESENTATION_ITEM ( '' )  );
#92091=CARTESIAN_POINT ( 'NONE',  ( 38.55793019189811588, 6.110000000000000320, -1.637169565754156064 ) ) ;
#92103=CARTESIAN_POINT ( 'NONE',  ( 41.78752705046289151, 0.000000000000000000, -7.949999999999998401 ) ) ;
#92125=CARTESIAN_POINT ( 'NONE',  ( 99.07876352523145158, -7.482591942790327058E-16, 6.109999999999999432 ) ) ;
#92155=CARTESIAN_POINT ( 'NONE',  ( 111.3958333333333144, -2.130196079827427091, 7.949999999999998401 ) ) ;
#92173=CARTESIAN_POINT ( 'NONE',  ( 123.5000000000000000, 0.000000000000000000, -7.950000000000000178 ) ) ;
#92185=CARTESIAN_POINT ( 'NONE',  ( 113.4587635252314470, 0.000000000000000000, -6.110000000000001208 ) ) ;
#92195=CARTESIAN_POINT ( 'NONE',  ( 37.70419371712956291, -6.884901960086285300, -3.975000000000000089 ) ) ;
#92200=CARTESIAN_POINT ( 'NONE',  ( 33.37499999999998579, 7.950000000000000178, 1.460391307983218535E-15 ) ) ;
#92212=CARTESIAN_POINT ( 'NONE',  ( 28.00043019189810067, -3.055000000000002380, 5.291415217122920289 ) ) ;
#92225=CARTESIAN_POINT ( 'NONE',  ( 39.01669371712955581, 7.950000000000000178, -2.130196079827421318 ) ) ;
#92231=CARTESIAN_POINT ( 'NONE',  ( 45.12043019189810877, 3.055000000000001936, -5.291415217122916737 ) ) ;
#92262=CARTESIAN_POINT ( 'NONE',  ( 65.82876352523145158, 0.000000000000000000, -6.109999999999998543 ) ) ;
#92272=CARTESIAN_POINT ( 'NONE',  ( 101.4791666666666430, -7.950000000000000178, 2.130196079827424427 ) ) ;
#92324=CARTESIAN_POINT ( 'NONE',  ( 64.82919371712955581, -3.975000000000001865, 6.884901960086284411 ) ) ;
#92333=CARTESIAN_POINT ( 'NONE',  ( 46.87043019189811588, -3.055000000000001936, 5.291415217122918513 ) ) ;
#92357=VECTOR ( 'NONE', #131413, 1000.000000000000000 ) ;
#92359=CARTESIAN_POINT ( 'NONE',  ( 117.0833333333333286, 6.884901960086290629, -3.974999999999994316 ) ) ;
#92360=CARTESIAN_POINT ( 'NONE',  ( 76.93336038379621300, 2.130196079827431532, -7.949999999999997513 ) ) ;
#92364=CARTESIAN_POINT ( 'NONE',  ( 61.08333333333332149, 6.884901960086290629, -3.974999999999994316 ) ) ;
#92372=CARTESIAN_POINT ( 'NONE',  ( 59.50043019189810423, -3.055000000000002380, 5.291415217122920289 ) ) ;
#92404=CARTESIAN_POINT ( 'NONE',  ( 73.14169371712955581, -2.130196079827424871, -7.949999999999998401 ) ) ;
#92419=CARTESIAN_POINT ( 'NONE',  ( 38.14169371712954870, -2.130196079827424871, -7.949999999999998401 ) ) ;
#92426=CARTESIAN_POINT ( 'NONE',  ( 91.20376352523145158, 6.109999999999998543, 1.122388791418548911E-15 ) ) ;
#92449=VERTEX_POINT ( 'NONE', #104574 ) ;
#92451=CARTESIAN_POINT ( 'NONE',  ( 48.56293019189809712, 1.637169565754157174, 6.110000000000002984 ) ) ;
#92495=CARTESIAN_POINT ( 'NONE',  ( 95.79166666666665719, 3.975000000000003642, -6.884901960086285300 ) ) ;
#92506=CARTESIAN_POINT ( 'NONE',  ( 9.179067077831442489, 8.505508952922598453, 4.232065175675569613 ) ) ;
#92508=CARTESIAN_POINT ( 'NONE',  ( 80.18749999999998579, -5.819803920172573974, 5.819803920172573086 ) ) ;
#92528=CARTESIAN_POINT ( 'NONE',  ( 100.1208603837962272, -6.884901960086286188, 3.974999999999997424 ) ) ;
#92541=CARTESIAN_POINT ( 'NONE',  ( 93.04209685856476142, 5.291415217122923842, -3.054999999999996163 ) ) ;
#92567=CARTESIAN_POINT ( 'NONE',  ( 86.91709685856477563, 3.054999999999998828, 5.291415217122922066 ) ) ;
#92581=CARTESIAN_POINT ( 'NONE',  ( 74.28709685856478018, 3.054999999999997495, 5.291415217122919401 ) ) ;
#92611=DIRECTION ( 'NONE',  ( 0.000000000000000000, 0.000000000000000000, 1.000000000000000000 ) ) ;
#92628=CARTESIAN_POINT ( 'NONE',  ( 72.47959685856477563, 6.109999999999999432, 1.637169565754164280 ) ) ;
#92631=CARTESIAN_POINT ( 'NONE',  ( 94.18750000000000000, -5.819803920172573974, 5.819803920172573086 ) ) ;
#92633=CARTESIAN_POINT ( 'NONE',  ( 110.1045968585647756, 1.637169565754164946, -6.109999999999999432 ) ) ;
#92639=DIRECTION ( 'NONE',  ( -1.000000000000000000, -0.000000000000000000, -0.000000000000000000 ) ) ;
#92657=CARTESIAN_POINT ( 'NONE',  ( 113.5833333333333428, 6.884901960086290629, -3.974999999999994316 ) ) ;
#92666=CARTESIAN_POINT ( 'NONE',  ( 8.378320375002967779, -8.650595726116820927, 3.928333035411932794 ) ) ;
#92667=CARTESIAN_POINT ( 'NONE',  ( 14.67075049121845431, -9.486428195927288698, -0.5820279030346748872 ) ) ;
#92682=ADVANCED_FACE ( 'NONE', ( #45074 ), #79123, .T. ) ;
#92696=AXIS2_PLACEMENT_3D ( 'NONE', #42626, #120115, #20824 ) ;
#92700=CARTESIAN_POINT ( 'NONE',  ( 104.3958333333333286, -2.130196079827389344, 7.950000000000021494 ) ) ;
#92706=CARTESIAN_POINT ( 'NONE',  ( 28.34959685856477662, 6.109999999999997655, 1.637169565754163836 ) ) ;
#92722=CARTESIAN_POINT ( 'NONE',  ( 96.22916666666667140, 7.950000000000001954, -2.130196079827421762 ) ) ;
#92728=CARTESIAN_POINT ( 'NONE',  ( 14.55667305106308973, 9.434713282303595960, 1.148153153331950227 ) ) ;
#92733=CARTESIAN_POINT ( 'NONE',  ( 125.6578181545542918, -1.266560775613104317, -7.692714378292049737 ) ) ;
#92746=CARTESIAN_POINT ( 'NONE',  ( 108.6462635252314186, -4.472830434245840259, 4.472830434245839371 ) ) ;
#92759=CARTESIAN_POINT ( 'NONE',  ( 104.7662635252314516, 4.472830434245839371, -4.472830434245838482 ) ) ;
#92765=AXIS2_PLACEMENT_3D ( 'NONE', #47802, #4182, #70284 ) ;
#92767=( BOUNDED_CURVE ( )  B_SPLINE_CURVE ( 2, ( #54862, #43976, #95653, #63771, #88196, #28279, #105794, #10595, #84113, #40588, #132447, #96337, #121507 ),
 .UNSPECIFIED., .F., .T. ) 
 B_SPLINE_CURVE_WITH_KNOTS ( ( 3, 2, 2, 2, 2, 2, 3 ),
 ( 0.8500000000000000888, 0.8527777777777778567, 0.8555555555555556246, 0.8583333333333333925, 0.8611111111111112715, 0.8638888888888890394, 0.8666666666666668073 ),
 .UNSPECIFIED. ) 
 CURVE ( )  GEOMETRIC_REPRESENTATION_ITEM ( )  RATIONAL_B_SPLINE_CURVE ( ( 0.9999999999999986677, 0.9659258262890696445, 1.000000000000000000, 0.9659258262890683122, 1.000000000000000000, 0.9659258262890683122, 1.000000000000000000, 0.9659258262890683122, 1.000000000000000000, 0.9659258262890683122, 1.000000000000000000, 0.9659258262890669799, 1.000000000000001332 ) ) 
 REPRESENTATION_ITEM ( '' )  );
#92812=CARTESIAN_POINT ( 'NONE',  ( 36.80793019189809456, -6.109999999999998543, 1.637169565754158507 ) ) ;
#92847=CARTESIAN_POINT ( 'NONE',  ( 97.03709685856479439, -3.054999999999999272, -5.291415217122919401 ) ) ;
#92902=CARTESIAN_POINT ( 'NONE',  ( 124.6666666666666572, 6.884901960086285300, 3.975000000000003642 ) ) ;
#92917=CARTESIAN_POINT ( 'NONE',  ( 112.5837635252314470, -6.110000000000001208, -3.741295971395164515E-16 ) ) ;
#92925=CARTESIAN_POINT ( 'NONE',  ( 37.41252705046288440, -7.949999999999998401, -4.867971026610728450E-16 ) ) ;
#92931=CARTESIAN_POINT ( 'NONE',  ( 36.72916666666666430, 7.950000000000001954, -2.130196079827421762 ) ) ;
#92935=EDGE_CURVE ( 'NONE', #90062, #116147, #104635, .T. ) ;
#92945=CARTESIAN_POINT ( 'NONE',  ( 32.52126352523142572, -4.472830434245839371, -4.472830434245840259 ) ) ;
#92966=CARTESIAN_POINT ( 'NONE',  ( 53.28709685856478018, 3.054999999999997495, 5.291415217122919401 ) ) ;
#93000=CARTESIAN_POINT ( 'NONE',  ( 69.03709685856478018, -3.054999999999998828, -5.291415217122919401 ) ) ;
#93042=CARTESIAN_POINT ( 'NONE',  ( 109.0625000000000000, -5.819803920172573086, -5.819803920172573974 ) ) ;
#93077=CARTESIAN_POINT ( 'NONE',  ( 43.07876352523144448, -7.482591942790327058E-16, 6.109999999999999432 ) ) ;
#93102=CARTESIAN_POINT ( 'NONE',  ( 64.82919371712955581, -3.975000000000001865, 6.884901960086284411 ) ) ;
#93106=CARTESIAN_POINT ( 'NONE',  ( 64.43749999999998579, 5.819803920172573974, -5.819803920172572198 ) ) ;
#93113=CARTESIAN_POINT ( 'NONE',  ( 32.79166666666666430, 3.975000000000003642, -6.884901960086285300 ) ) ;
#93117=CARTESIAN_POINT ( 'NONE',  ( 56.14626352523143282, -4.472830434245840259, 4.472830434245839371 ) ) ;
#93143=CARTESIAN_POINT ( 'NONE',  ( 72.41252705046288440, -7.949999999999998401, -4.867971026610728450E-16 ) ) ;
#93151=VERTEX_POINT ( 'NONE', #17052 ) ;
#93152=CARTESIAN_POINT ( 'NONE',  ( 61.91252705046289151, -7.949999999999998401, -4.867971026610728450E-16 ) ) ;
#93164=VERTEX_POINT ( 'NONE', #125824 ) ;
#93167=CARTESIAN_POINT ( 'NONE',  ( 92.22459685856479439, -1.637169565754160949, 6.109999999999997655 ) ) ;
#93191=CARTESIAN_POINT ( 'NONE',  ( 48.85459685856476852, -1.637169565754161615, 6.110000000000000320 ) ) ;
#93210=CIRCLE ( 'NONE', #7509, 6.349999999999997868 ) ;
#93223=DIRECTION ( 'NONE',  ( -1.000000000000000000, -0.000000000000000000, -0.000000000000000000 ) ) ;
#93228=CARTESIAN_POINT ( 'NONE',  ( 95.64583333333332860, 2.130196079827431976, -7.949999999999998401 ) ) ;
#93235=CARTESIAN_POINT ( 'NONE',  ( 95.74586038379622721, 3.974999999999996980, 6.884901960086287964 ) ) ;
#93241=CARTESIAN_POINT ( 'NONE',  ( 70.64126352523145158, 4.472830434245837594, 4.472830434245841147 ) ) ;
#93242=CARTESIAN_POINT ( 'NONE',  ( 81.06249999999998579, -5.819803920172573086, -5.819803920172573974 ) ) ;
#93266=CARTESIAN_POINT ( 'NONE',  ( 91.80836038379622721, 7.949999999999997513, 2.130196079827431088 ) ) ;
#93282=CARTESIAN_POINT ( 'NONE',  ( 81.22959685856476142, -6.110000000000000320, -1.637169565754161393 ) ) ;
#93305=CARTESIAN_POINT ( 'NONE',  ( 80.06293019189810423, 1.637169565754157174, 6.110000000000002984 ) ) ;
#93330=DIRECTION ( 'NONE',  ( -1.000000000000000000, -0.000000000000000000, -0.000000000000000000 ) ) ;
#93349=DIRECTION ( 'NONE',  ( -1.000000000000000000, -0.000000000000000000, -0.000000000000000000 ) ) ;
#93355=LINE ( 'NONE', #71613, #58796 ) ;
#93366=CARTESIAN_POINT ( 'NONE',  ( 76.27126352523144703, 4.472830434245838482, 4.472830434245842035 ) ) ;
#93370=CARTESIAN_POINT ( 'NONE',  ( 111.5629301918981184, 1.637169565754157174, 6.110000000000002984 ) ) ;
#93441=CARTESIAN_POINT ( 'NONE',  ( 29.80793019189811588, -6.109999999999999432, 1.637169565754158507 ) ) ;
#93456=CARTESIAN_POINT ( 'NONE',  ( 89.37500000000000000, 7.950000000000000178, 1.460391307983218535E-15 ) ) ;
#93466=CARTESIAN_POINT ( 'NONE',  ( -7.888753617628999938E-63, -6.350000000000004086, -3.888253587292849040E-16 ) ) ;
#93468=CARTESIAN_POINT ( 'NONE',  ( 126.7090635503642062, 5.466269142923943392, 3.952704227923545144 ) ) ;
#93481=CARTESIAN_POINT ( 'NONE',  ( 111.8545968585647756, -1.637169565754161615, 6.110000000000000320 ) ) ;
#93484=EDGE_CURVE ( 'NONE', #93151, #141150, #97410, .T. ) ;
#93491=CARTESIAN_POINT ( 'NONE',  ( 106.3704301918981230, -3.055000000000001492, 5.291415217122917625 ) ) ;
#93531=CARTESIAN_POINT ( 'NONE',  ( 63.07919371712955581, 3.975000000000002753, -6.884901960086283523 ) ) ;
#93541=CARTESIAN_POINT ( 'NONE',  ( 34.03709685856478018, -3.054999999999998828, -5.291415217122919401 ) ) ;
#93577=CARTESIAN_POINT ( 'NONE',  ( 105.7870968585647802, 3.054999999999997939, 5.291415217122920289 ) ) ;
#93625=CARTESIAN_POINT ( 'NONE',  ( 29.24586038379621655, 3.974999999999996980, 6.884901960086287964 ) ) ;
#93630=CARTESIAN_POINT ( 'NONE',  ( 117.5208333333333428, 7.949999999999999289, 2.130196079827431532 ) ) ;
#93645=CARTESIAN_POINT ( 'NONE',  ( 112.2920968585647756, -5.291415217122921177, 3.054999999999999272 ) ) ;
#93650=CARTESIAN_POINT ( 'NONE',  ( 82.47502705046287019, -5.819803920172573086, 5.819803920172573086 ) ) ;
#93653=DIRECTION ( 'NONE',  ( -1.000000000000000000, -0.000000000000000000, -0.000000000000000000 ) ) ;
#93655=CARTESIAN_POINT ( 'NONE',  ( 33.91252705046289861, -7.949999999999998401, -4.867971026610728450E-16 ) ) ;
#93663=CARTESIAN_POINT ( 'NONE',  ( 38.33333333333332860, -6.884901960086287964, 3.974999999999998312 ) ) ;
#93672=CARTESIAN_POINT ( 'NONE',  ( 128.5370968585647802, -3.054999999999998828, -5.291415217122919401 ) ) ;
#93681=CARTESIAN_POINT ( 'NONE',  ( 53.81293019189810423, -1.637169565754159617, -6.110000000000001208 ) ) ;
#93688=CARTESIAN_POINT ( 'NONE',  ( 47.74543019189811588, -5.291415217122918513, -3.055000000000000160 ) ) ;
#93716=CARTESIAN_POINT ( 'NONE',  ( 61.45376352523145158, -6.109999999999998543, -3.741295971395162543E-16 ) ) ;
#93718=CARTESIAN_POINT ( 'NONE',  ( 46.50000000000000000, 0.000000000000000000, -7.950000000000000178 ) ) ;
#93789=CARTESIAN_POINT ( 'NONE',  ( 50.07876352523145158, -7.482591942790327058E-16, 6.109999999999999432 ) ) ;
#93791=ORIENTED_EDGE ( 'NONE', *, *, #54549, .F. ) ;
#93808=( BOUNDED_CURVE ( )  B_SPLINE_CURVE ( 2, ( #32219, #130110, #86613, #98189, #97447, #40266, #109769, #119207, #130841, #41655, #19196, #31504, #76451 ),
 .UNSPECIFIED., .F., .T. ) 
 B_SPLINE_CURVE_WITH_KNOTS ( ( 3, 2, 2, 2, 2, 2, 3 ),
 ( 0.04999999999999305000, 0.05277777777777043627, 0.05555555555554782948, 0.05833333333332522269, 0.06111111111110260896, 0.06388888888888000217, 0.06666666666665739538 ),
 .UNSPECIFIED. ) 
 CURVE ( )  GEOMETRIC_REPRESENTATION_ITEM ( )  RATIONAL_B_SPLINE_CURVE ( ( 1.000000000000085487, 0.9659258262889831581, 1.000000000000000000, 0.9659258262890683122, 1.000000000000000000, 0.9659258262890683122, 1.000000000000000000, 0.9659258262890683122, 1.000000000000000000, 0.9659258262890683122, 1.000000000000000000, 0.9659258262891819991, 0.9999999999998863132 ) ) 
 REPRESENTATION_ITEM ( '' )  );
#93809=CARTESIAN_POINT ( 'NONE',  ( 104.0583603837961988, -7.949999999999996625, -2.130196079827426203 ) ) ;
#93810=CARTESIAN_POINT ( 'NONE',  ( 66.28752705046289861, 0.000000000000000000, -7.949999999999998401 ) ) ;
#93816=CARTESIAN_POINT ( 'NONE',  ( 67.79166666666667140, 3.975000000000003642, -6.884901960086285300 ) ) ;
#93825=CARTESIAN_POINT ( 'NONE',  ( 58.91709685856477563, 3.054999999999998828, 5.291415217122922066 ) ) ;
#93826=CARTESIAN_POINT ( 'NONE',  ( 0.000000000000000000, 0.000000000000000000, 7.950000000000000178 ) ) ;
#93849=DIRECTION ( 'NONE',  ( -1.000000000000000000, -0.000000000000000000, -0.000000000000000000 ) ) ;
#93850=CARTESIAN_POINT ( 'NONE',  ( 71.53752705046289861, -9.735942053221456900E-16, 7.949999999999998401 ) ) ;
#93867=ORIENTED_EDGE ( 'NONE', *, *, #107812, .F. ) ;
#93873=CARTESIAN_POINT ( 'NONE',  ( 97.32876352523145158, 0.000000000000000000, -6.109999999999998543 ) ) ;
#93884=LINE ( 'NONE', #5428, #11039 ) ;
#93889=CARTESIAN_POINT ( 'NONE',  ( 153.6500000000000057, 0.000000000000000000, 0.000000000000000000 ) ) ;
#93890=ORIENTED_EDGE ( 'NONE', *, *, #141743, .T. ) ;
#93896=CARTESIAN_POINT ( 'NONE',  ( 43.31293019189811133, -1.637169565754159617, -6.110000000000001208 ) ) ;
#93910=ORIENTED_EDGE ( 'NONE', *, *, #35134, .F. ) ;
#93916=ORIENTED_EDGE ( 'NONE', *, *, #57686, .T. ) ;
#93941=VERTEX_POINT ( 'NONE', #92103 ) ;
#93944=CARTESIAN_POINT ( 'NONE',  ( 94.72502705046289861, 5.819803920172573974, -5.819803920172573086 ) ) ;
#93951=CARTESIAN_POINT ( 'NONE',  ( 78.80793019189810877, -6.109999999999999432, 1.637169565754158507 ) ) ;
#93953=CARTESIAN_POINT ( 'NONE',  ( 74.01669371712955581, 7.950000000000000178, -2.130196079827421318 ) ) ;
#93972=CARTESIAN_POINT ( 'NONE',  ( 91.37086038379622721, 6.884901960086289741, -3.974999999999993427 ) ) ;
#93985=CARTESIAN_POINT ( 'NONE',  ( 88.37543019189811844, -5.291415217122920289, -3.055000000000001492 ) ) ;
#94003=CARTESIAN_POINT ( 'NONE',  ( 77.29209685856477563, -5.291415217122921177, 3.054999999999999272 ) ) ;
#94004=VERTEX_POINT ( 'NONE', #138491 ) ;
#94031=CARTESIAN_POINT ( 'NONE',  ( 53.30836038379622721, 7.949999999999996625, 2.130196079827431088 ) ) ;
#94064=CARTESIAN_POINT ( 'NONE',  ( 69.27126352523144703, 4.472830434245838482, 4.472830434245842035 ) ) ;
#94069=CARTESIAN_POINT ( 'NONE',  ( 113.0212635252314044, -4.472830434245838482, -4.472830434245840259 ) ) ;
#94122=CARTESIAN_POINT ( 'NONE',  ( 105.5624999999999858, -5.819803920172573086, -5.819803920172573974 ) ) ;
#94133=CARTESIAN_POINT ( 'NONE',  ( 118.7875270504628986, 0.000000000000000000, -7.949999999999998401 ) ) ;
#94148=CARTESIAN_POINT ( 'NONE',  ( 81.06249999999998579, -5.819803920172572198, -5.819803920172573086 ) ) ;
#94172=CARTESIAN_POINT ( 'NONE',  ( 99.16709685856477563, -3.055000000000000160, -5.291415217122921177 ) ) ;
#94180=CARTESIAN_POINT ( 'NONE',  ( 75.66666666666665719, 6.884901960086285300, 3.975000000000003642 ) ) ;
#94182=CARTESIAN_POINT ( 'NONE',  ( 100.9745968585647660, 1.637169565754164058, -6.109999999999996767 ) ) ;
#94214=CARTESIAN_POINT ( 'NONE',  ( 110.8912635252314658, -4.472830434245838482, -4.472830434245838482 ) ) ;
#94241=CARTESIAN_POINT ( 'NONE',  ( 30.68293019189811943, -1.637169565754158951, -6.109999999999998543 ) ) ;
#94276=CARTESIAN_POINT ( 'NONE',  ( 101.2662635252314374, 4.472830434245839371, -4.472830434245839371 ) ) ;
#94320=CARTESIAN_POINT ( 'NONE',  ( 26.04475813788241112, 1.701477371937655247, -6.349999999999989875 ) ) ;
#94327=CARTESIAN_POINT ( 'NONE',  ( 114.6041666666666572, 2.130196079827422206, 7.950000000000001954 ) ) ;
#94341=CARTESIAN_POINT ( 'NONE',  ( 117.2504301918981042, 3.055000000000002824, -5.291415217122919401 ) ) ;
#94350=CARTESIAN_POINT ( 'NONE',  ( 40.47502705046289861, -5.819803920172572198, 5.819803920172572198 ) ) ;
#94355=CARTESIAN_POINT ( 'NONE',  ( 40.81250000000000711, 5.819803920172571310, 5.819803920172575751 ) ) ;
#94363=CARTESIAN_POINT ( 'NONE',  ( 28.87543019189810067, -5.291415217122920289, -3.055000000000001492 ) ) ;
#94371=CARTESIAN_POINT ( 'NONE',  ( 59.20876352523143993, -7.482591942790329030E-16, 6.110000000000001208 ) ) ;
#94379=CARTESIAN_POINT ( 'NONE',  ( 49.78709685856478018, 3.054999999999997495, 5.291415217122919401 ) ) ;
#94385=ADVANCED_FACE ( 'NONE', ( #98415 ), #18681, .F. ) ;
#94386=ORIENTED_EDGE ( 'NONE', *, *, #88539, .T. ) ;
#94396=ADVANCED_FACE ( 'NONE', ( #96233 ), #131044, .T. ) ;
#94411=CARTESIAN_POINT ( 'NONE',  ( 65.39126352523145158, -4.472830434245838482, -4.472830434245838482 ) ) ;
#94414=DIRECTION ( 'NONE',  ( -1.000000000000000000, -0.000000000000000000, -0.000000000000000000 ) ) ;
#94420=CARTESIAN_POINT ( 'NONE',  ( 101.3333333333333286, -6.884901960086287964, 3.974999999999998312 ) ) ;
#94485=CARTESIAN_POINT ( 'NONE',  ( 45.70376352523145158, 6.109999999999999432, 1.122388791418549108E-15 ) ) ;
#94506=CARTESIAN_POINT ( 'NONE',  ( 61.76669371712955581, -7.949999999999999289, 2.130196079827424427 ) ) ;
#94511=CARTESIAN_POINT ( 'NONE',  ( 63.41666666666666430, -6.884901960086287076, -3.975000000000000977 ) ) ;
#94519=CARTESIAN_POINT ( 'NONE',  ( 56.87543019189809712, -5.291415217122920289, -3.055000000000001492 ) ) ;
#94575=CARTESIAN_POINT ( 'NONE',  ( 94.26626352523143737, 4.472830434245838482, -4.472830434245837594 ) ) ;
#94586=CARTESIAN_POINT ( 'NONE',  ( 153.6500000000000057, 0.000000000000000000, 0.000000000000000000 ) ) ;
#94588=DIRECTION ( 'NONE',  ( -1.000000000000000000, -0.000000000000000000, -0.000000000000000000 ) ) ;
#94601=CARTESIAN_POINT ( 'NONE',  ( 40.83376352523143993, 6.110000000000001208, 1.122388791418549305E-15 ) ) ;
#94636=( BOUNDED_CURVE ( )  B_SPLINE_CURVE ( 2, ( #66029, #42841, #131256, #7305, #120331, #65317, #109501, #95764, #129821, #77613, #24626, #57297, #100769 ),
 .UNSPECIFIED., .F., .T. ) 
 B_SPLINE_CURVE_WITH_KNOTS ( ( 3, 2, 2, 2, 2, 2, 3 ),
 ( 0.3500000000000000333, 0.3527777777777778567, 0.3555555555555556246, 0.3583333333333333925, 0.3611111111111111605, 0.3638888888888889284, 0.3666666666666666963 ),
 .UNSPECIFIED. ) 
 CURVE ( )  GEOMETRIC_REPRESENTATION_ITEM ( )  RATIONAL_B_SPLINE_CURVE ( ( 0.9999999999999993339, 0.9659258262890689783, 1.000000000000000000, 0.9659258262890683122, 1.000000000000000000, 0.9659258262890683122, 1.000000000000000000, 0.9659258262890683122, 1.000000000000000000, 0.9659258262890683122, 1.000000000000000000, 0.9659258262890676461, 1.000000000000000666 ) ) 
 REPRESENTATION_ITEM ( '' )  );
#94649=CARTESIAN_POINT ( 'NONE',  ( 79.24543019189810877, -5.291415217122919401, -3.055000000000000604 ) ) ;
#94650=CARTESIAN_POINT ( 'NONE',  ( 80.91666666666667140, -6.884901960086287076, -3.975000000000000977 ) ) ;
#94671=CARTESIAN_POINT ( 'NONE',  ( 121.1208603837962272, -6.884901960086286188, 3.974999999999997424 ) ) ;
#94674=CARTESIAN_POINT ( 'NONE',  ( 91.95419371712957002, 6.884901960086283523, 3.975000000000002753 ) ) ;
#94684=ADVANCED_FACE ( 'NONE', ( #138186 ), #95382, .T. ) ;
#94687=CARTESIAN_POINT ( 'NONE',  ( 82.39626352523143282, 4.472830434245840259, -4.472830434245839371 ) ) ;
#94704=CARTESIAN_POINT ( 'NONE',  ( 76.27126352523144703, 4.472830434245839371, 4.472830434245842035 ) ) ;
#94747=DIRECTION ( 'NONE',  ( -1.000000000000000000, -0.000000000000000000, -0.000000000000000000 ) ) ;
#94752=CARTESIAN_POINT ( 'NONE',  ( 26.99999999999998934, -5.093796677280518104, -4.382233278760884865 ) ) ;
#94765=CARTESIAN_POINT ( 'NONE',  ( 70.72959685856477563, -6.110000000000000320, -1.637169565754161393 ) ) ;
#94773=CARTESIAN_POINT ( 'NONE',  ( 105.0004301918981184, -3.055000000000002380, 5.291415217122920289 ) ) ;
#94810=ORIENTED_EDGE ( 'NONE', *, *, #76799, .F. ) ;
#94832=CARTESIAN_POINT ( 'NONE',  ( 123.0166937171295416, 7.950000000000001066, -2.130196079827421318 ) ) ;
#94850=CARTESIAN_POINT ( 'NONE',  ( 81.20833333333332860, -3.974999999999999201, -6.884901960086287964 ) ) ;
#94878=CARTESIAN_POINT ( 'NONE',  ( 100.6254301918981042, 5.291415217122919401, 3.055000000000002824 ) ) ;
#94888=CARTESIAN_POINT ( 'NONE',  ( 98.34959685856479439, 6.109999999999996767, 1.637169565754163836 ) ) ;
#94916=CARTESIAN_POINT ( 'NONE',  ( 110.0162635252314374, -4.472830434245838482, 4.472830434245838482 ) ) ;
#94937=VERTEX_POINT ( 'NONE', #55469 ) ;
#94941=CARTESIAN_POINT ( 'NONE',  ( 26.74543019189810877, -5.291415217122918513, -3.055000000000000160 ) ) ;
#94974=CARTESIAN_POINT ( 'NONE',  ( 99.66209685856478018, -5.291415217122919401, 3.054999999999998384 ) ) ;
#95018=CARTESIAN_POINT ( 'NONE',  ( 25.89892480454907542, 0.000000000000000000, -6.350000000000003197 ) ) ;
#95026=CARTESIAN_POINT ( 'NONE',  ( 108.0416666666666714, -3.975000000000002753, 6.884901960086286188 ) ) ;
#95045=CARTESIAN_POINT ( 'NONE',  ( 100.4795968585647614, 6.109999999999999432, 1.637169565754164280 ) ) ;
#95056=CARTESIAN_POINT ( 'NONE',  ( 36.68336038379623432, -2.130196079827426203, 7.949999999999997513 ) ) ;
#95061=CARTESIAN_POINT ( 'NONE',  ( 25.06249999999998934, -5.819803920172572198, -5.819803920172573086 ) ) ;
#95072=CARTESIAN_POINT ( 'NONE',  ( 25.52126352523142927, -4.472830434245839371, -4.472830434245840259 ) ) ;
#95085=CARTESIAN_POINT ( 'NONE',  ( 42.14626352523143282, -4.472830434245840259, 4.472830434245839371 ) ) ;
#95093=CARTESIAN_POINT ( 'NONE',  ( 48.47459685856478728, 1.637169565754164058, -6.109999999999996767 ) ) ;
#95106=CARTESIAN_POINT ( 'NONE',  ( 44.99586038379622721, -3.974999999999998312, -6.884901960086286188 ) ) ;
#95121=ORIENTED_EDGE ( 'NONE', *, *, #109265, .F. ) ;
#95123=CARTESIAN_POINT ( 'NONE',  ( 52.70376352523144448, 6.109999999999998543, 1.122388791418548911E-15 ) ) ;
#95134=CARTESIAN_POINT ( 'NONE',  ( 101.6250000000000000, -7.950000000000000178, -4.867971026610729436E-16 ) ) ;
#95159=CARTESIAN_POINT ( 'NONE',  ( 128.2454301918981230, -5.291415217122919401, -3.055000000000000604 ) ) ;
#95180=CYLINDRICAL_SURFACE ( 'NONE', #60936, 7.950000000000000178 ) ;
#95205=CARTESIAN_POINT ( 'NONE',  ( 46.72459685856476597, -1.637169565754161171, 6.109999999999998543 ) ) ;
#95229=CARTESIAN_POINT ( 'NONE',  ( 67.60002705046289861, 5.819803920172570422, 5.819803920172574863 ) ) ;
#95230=CARTESIAN_POINT ( 'NONE',  ( 127.3989248045490967, 0.000000000000000000, -6.349999999999997868 ) ) ;
#95233=CARTESIAN_POINT ( 'NONE',  ( 52.77083333333332149, -7.949999999999999289, -2.130196079827426203 ) ) ;
#95242=CARTESIAN_POINT ( 'NONE',  ( 54.68793019189810423, 6.110000000000002984, -1.637169565754156730 ) ) ;
#95269=CARTESIAN_POINT ( 'NONE',  ( 77.78709685856478018, 3.054999999999997495, 5.291415217122919401 ) ) ;
#95273=CARTESIAN_POINT ( 'NONE',  ( 72.26669371712955581, -7.949999999999998401, 2.130196079827423983 ) ) ;
#95277=CARTESIAN_POINT ( 'NONE',  ( 0.000000000000000000, 0.000000000000000000, 0.000000000000000000 ) ) ;
#95299=CARTESIAN_POINT ( 'NONE',  ( 87.26626352523145158, 4.472830434245838482, -4.472830434245837594 ) ) ;
#95323=EDGE_CURVE ( 'NONE', #14445, #102139, #33537, .T. ) ;
#95327=CARTESIAN_POINT ( 'NONE',  ( 43.16709685856477563, -3.055000000000000160, -5.291415217122921177 ) ) ;
#95358=CARTESIAN_POINT ( 'NONE',  ( 67.50000000000000000, 0.000000000000000000, -7.950000000000000178 ) ) ;
#95367=ORIENTED_EDGE ( 'NONE', *, *, #108955, .T. ) ;
#95377=CARTESIAN_POINT ( 'NONE',  ( 79.53709685856478018, -3.054999999999999272, -5.291415217122919401 ) ) ;
#95382=CYLINDRICAL_SURFACE ( 'NONE', #11333, 7.950000000000000178 ) ;
#95404=CARTESIAN_POINT ( 'NONE',  ( 94.87086038379621300, 6.884901960086289741, -3.974999999999993427 ) ) ;
#95418=CARTESIAN_POINT ( 'NONE',  ( 83.70876352523143282, -7.482591942790329030E-16, 6.110000000000001208 ) ) ;
#95438=CARTESIAN_POINT ( 'NONE',  ( 70.58376352523143282, -6.110000000000001208, -3.741295971395164515E-16 ) ) ;
#95449=VERTEX_POINT ( 'NONE', #71704 ) ;
#95453=CARTESIAN_POINT ( 'NONE',  ( 33.91252705046289861, -7.949999999999998401, -4.867971026610728450E-16 ) ) ;
#95481=EDGE_LOOP ( 'NONE', ( #85880, #105537, #43071, #125855 ) ) ;
#95483=CARTESIAN_POINT ( 'NONE',  ( 51.31249999999999289, 5.819803920172571310, 5.819803920172576639 ) ) ;
#95491=CARTESIAN_POINT ( 'NONE',  ( 77.00043019189811844, -3.055000000000002380, 5.291415217122920289 ) ) ;
#95495=CARTESIAN_POINT ( 'NONE',  ( 108.2087635252314470, -7.482591942790329030E-16, 6.110000000000001208 ) ) ;
#95527=CARTESIAN_POINT ( 'NONE',  ( 13.79782509673477087, -9.118585253093964837, 2.676058911687216213 ) ) ;
#95566=CARTESIAN_POINT ( 'NONE',  ( 125.0583603837962272, -7.949999999999997513, -2.130196079827425759 ) ) ;
#95583=CARTESIAN_POINT ( 'NONE',  ( 79.74999999999998579, -9.735942053221458872E-16, 7.950000000000000178 ) ) ;
#95587=CARTESIAN_POINT ( 'NONE',  ( 91.07919371712955581, 3.975000000000002753, -6.884901960086283523 ) ) ;
#95592=DIRECTION ( 'NONE',  ( -1.000000000000000000, -0.000000000000000000, -0.000000000000000000 ) ) ;
#95609=CARTESIAN_POINT ( 'NONE',  ( 99.31293019189810423, -1.637169565754159617, -6.110000000000001208 ) ) ;
#95619=CARTESIAN_POINT ( 'NONE',  ( 94.99543019189812298, 5.291415217122916737, 3.055000000000001936 ) ) ;
#95638=EDGE_LOOP ( 'NONE', ( #58233, #15887, #45450, #129538 ) ) ;
#95653=CARTESIAN_POINT ( 'NONE',  ( 37.45833333333332860, 3.974999999999997424, 6.884901960086288852 ) ) ;
#95667=CARTESIAN_POINT ( 'NONE',  ( 32.43293019189810877, 1.637169565754156508, 6.110000000000000320 ) ) ;
#95706=CARTESIAN_POINT ( 'NONE',  ( 90.91209685856478018, 5.291415217122922066, -3.054999999999995275 ) ) ;
#95721=EDGE_LOOP ( 'NONE', ( #69291, #18311, #29665, #93791 ) ) ;
#95751=CARTESIAN_POINT ( 'NONE',  ( 29.53752705046289151, -9.735942053221456900E-16, 7.949999999999998401 ) ) ;
#95759=CARTESIAN_POINT ( 'NONE',  ( 108.4791666666666714, -7.950000000000001066, 2.130196079827424427 ) ) ;
#95764=CARTESIAN_POINT ( 'NONE',  ( 89.22916666666667140, 7.950000000000001954, -2.130196079827421762 ) ) ;
#95770=CARTESIAN_POINT ( 'NONE',  ( 102.5212635252314328, -4.472830434245839371, -4.472830434245840259 ) ) ;
#95775=CARTESIAN_POINT ( 'NONE',  ( 82.03752705046288440, -9.735942053221456900E-16, 7.949999999999998401 ) ) ;
#95779=CARTESIAN_POINT ( 'NONE',  ( 28.66252705046289151, 7.949999999999998401, 1.460391307983218338E-15 ) ) ;
#95786=CARTESIAN_POINT ( 'NONE',  ( 31.04166666666666075, -3.975000000000002753, 6.884901960086286188 ) ) ;
#95794=CARTESIAN_POINT ( 'NONE',  ( 85.53752705046288440, -9.735942053221456900E-16, 7.949999999999998401 ) ) ;
#95795=CARTESIAN_POINT ( 'NONE',  ( 127.8079301918981230, -6.109999999999998543, 1.637169565754158063 ) ) ;
#95806=CARTESIAN_POINT ( 'NONE',  ( 48.56293019189809712, 1.637169565754157174, 6.110000000000002984 ) ) ;
#95815=CARTESIAN_POINT ( 'NONE',  ( 34.91209685856478018, 5.291415217122921177, -3.054999999999994831 ) ) ;
#95822=CARTESIAN_POINT ( 'NONE',  ( 59.28752705046289151, 0.000000000000000000, -7.949999999999998401 ) ) ;
#95844=CARTESIAN_POINT ( 'NONE',  ( 56.20376352523144448, 6.109999999999998543, 1.122388791418548911E-15 ) ) ;
#95864=ORIENTED_EDGE ( 'NONE', *, *, #125081, .F. ) ;
#95877=CARTESIAN_POINT ( 'NONE',  ( 121.2454301918981230, -5.291415217122919401, -3.055000000000000604 ) ) ;
#95878=( BOUNDED_CURVE ( )  B_SPLINE_CURVE ( 2, ( #140722, #98651, #41417, #30565, #19667, #142878, #87784, #74803, #118979, #97189, #33445, #42164, #132016 ),
 .UNSPECIFIED., .F., .T. ) 
 B_SPLINE_CURVE_WITH_KNOTS ( ( 3, 2, 2, 2, 2, 2, 3 ),
 ( 0.5500000000000000444, 0.5527777777777778123, 0.5555555555555555802, 0.5583333333333333481, 0.5611111111111111160, 0.5638888888888888840, 0.5666666666666666519 ),
 .UNSPECIFIED. ) 
 CURVE ( )  GEOMETRIC_REPRESENTATION_ITEM ( )  RATIONAL_B_SPLINE_CURVE ( ( 1.000000000000000000, 0.9659258262890683122, 1.000000000000000000, 0.9659258262890683122, 1.000000000000000000, 0.9659258262890683122, 1.000000000000000000, 0.9659258262890683122, 1.000000000000000000, 0.9659258262890683122, 1.000000000000000000, 0.9659258262890683122, 1.000000000000000000 ) ) 
 REPRESENTATION_ITEM ( '' )  );
#95922=CARTESIAN_POINT ( 'NONE',  ( 36.37043019189811588, -3.055000000000001936, 5.291415217122918513 ) ) ;
#95946=CARTESIAN_POINT ( 'NONE',  ( 69.93336038379619879, 2.130196079827431532, -7.949999999999997513 ) ) ;
#95950=CARTESIAN_POINT ( 'NONE',  ( 52.47916666666665719, -7.950000000000001066, 2.130196079827424427 ) ) ;
#95957=CARTESIAN_POINT ( 'NONE',  ( 50.31293019189810423, -1.637169565754159617, -6.110000000000001208 ) ) ;
#95978=CARTESIAN_POINT ( 'NONE',  ( 78.07876352523145158, -7.482591942790325086E-16, 6.109999999999998543 ) ) ;
#96010=CARTESIAN_POINT ( 'NONE',  ( 84.20376352523145158, 6.109999999999998543, 1.122388791418548911E-15 ) ) ;
#96034=CARTESIAN_POINT ( 'NONE',  ( 32.22959685856477563, -6.110000000000000320, -1.637169565754161393 ) ) ;
#96081=CARTESIAN_POINT ( 'NONE',  ( 71.80793019189812298, -6.109999999999999432, 1.637169565754158507 ) ) ;
#96105=CARTESIAN_POINT ( 'NONE',  ( 92.82919371712955581, -3.975000000000001865, 6.884901960086284411 ) ) ;
#96106=DIRECTION ( 'NONE',  ( -1.000000000000000000, -0.000000000000000000, -0.000000000000000000 ) ) ;
#96122=CARTESIAN_POINT ( 'NONE',  ( 74.95876352523143282, 0.000000000000000000, -6.110000000000001208 ) ) ;
#96128=CARTESIAN_POINT ( 'NONE',  ( 118.4958603837962272, -3.974999999999998312, -6.884901960086286188 ) ) ;
#96137=ORIENTED_EDGE ( 'NONE', *, *, #36159, .T. ) ;
#96138=CARTESIAN_POINT ( 'NONE',  ( 72.18793019189810423, 6.110000000000002984, -1.637169565754156730 ) ) ;
#96142=CARTESIAN_POINT ( 'NONE',  ( 0.000000000000000000, 9.735942053221458872E-16, -7.950000000000000178 ) ) ;
#96189=CARTESIAN_POINT ( 'NONE',  ( 62.85459685856477563, -1.637169565754161615, 6.110000000000000320 ) ) ;
#96197=CARTESIAN_POINT ( 'NONE',  ( 101.0629301918980900, 1.637169565754157174, 6.110000000000002984 ) ) ;
#96209=ORIENTED_EDGE ( 'NONE', *, *, #105058, .F. ) ;
#96222=CARTESIAN_POINT ( 'NONE',  ( 10.61403459356125190, -8.436352015943745286, -4.367863059733367415 ) ) ;
#96223=VERTEX_POINT ( 'NONE', #114135 ) ;
#96233=FACE_OUTER_BOUND ( 'NONE', #129029, .T. ) ;
#96234=CARTESIAN_POINT ( 'NONE',  ( 30.62543019189810423, 5.291415217122919401, 3.055000000000002824 ) ) ;
#96252=CARTESIAN_POINT ( 'NONE',  ( 125.3500270504628986, -5.819803920172572198, -5.819803920172572198 ) ) ;
#96292=CARTESIAN_POINT ( 'NONE',  ( 106.0212635252314470, -4.472830434245839371, -4.472830434245840259 ) ) ;
#96298=ORIENTED_EDGE ( 'NONE', *, *, #2876, .T. ) ;
#96302=CARTESIAN_POINT ( 'NONE',  ( 97.76626352523143737, 4.472830434245839371, -4.472830434245838482 ) ) ;
#96308=VERTEX_POINT ( 'NONE', #95230 ) ;
#96325=ADVANCED_FACE ( 'NONE', ( #82252 ), #114817, .T. ) ;
#96328=ORIENTED_EDGE ( 'NONE', *, *, #60905, .F. ) ;
#96337=CARTESIAN_POINT ( 'NONE',  ( 36.14583333333331439, 2.130196079827356037, -7.950000000000043698 ) ) ;
#96392=CARTESIAN_POINT ( 'NONE',  ( 90.47459685856479439, 1.637169565754164280, -6.109999999999997655 ) ) ;
#96436=CARTESIAN_POINT ( 'NONE',  ( 113.7291666666666572, 7.950000000000001954, -2.130196079827421762 ) ) ;
#96449=CARTESIAN_POINT ( 'NONE',  ( 105.4379301918981042, -6.110000000000001208, 1.637169565754158951 ) ) ;
#96459=CARTESIAN_POINT ( 'NONE',  ( 28.22502705046288440, 5.819803920172573086, -5.819803920172572198 ) ) ;
#96464=CARTESIAN_POINT ( 'NONE',  ( 26.95833333333332149, 3.974999999999997424, 6.884901960086288852 ) ) ;
#96469=CARTESIAN_POINT ( 'NONE',  ( 0.000000000000000000, 0.000000000000000000, 0.000000000000000000 ) ) ;
#96474=CARTESIAN_POINT ( 'NONE',  ( 120.8079301918980946, -6.109999999999998543, 1.637169565754158063 ) ) ;
#96484=CARTESIAN_POINT ( 'NONE',  ( 47.54209685856476852, 5.291415217122923842, -3.054999999999996163 ) ) ;
#96494=CARTESIAN_POINT ( 'NONE',  ( 39.43293019189811588, 1.637169565754156508, 6.110000000000000320 ) ) ;
#96507=CARTESIAN_POINT ( 'NONE',  ( 44.26669371712954870, -7.949999999999998401, 2.130196079827423983 ) ) ;
#96525=CARTESIAN_POINT ( 'NONE',  ( 60.28709685856478728, 3.054999999999997495, 5.291415217122919401 ) ) ;
#96534=( BOUNDED_CURVE ( )  B_SPLINE_CURVE ( 2, ( #116463, #39645, #18537, #61418, #83871, #126601, #83128, #127326, #62822, #28030, #27292, #128075, #104868 ),
 .UNSPECIFIED., .F., .F. ) 
 B_SPLINE_CURVE_WITH_KNOTS ( ( 3, 2, 2, 2, 2, 2, 3 ),
 ( 0.7833333333333333259, 0.7861111111111110938, 0.7888888888888888618, 0.7916666666666666297, 0.7944444444444443976, 0.7972222222222222765, 0.8000000000000000444 ),
 .UNSPECIFIED. ) 
 CURVE ( )  GEOMETRIC_REPRESENTATION_ITEM ( )  RATIONAL_B_SPLINE_CURVE ( ( 1.000000000000000000, 0.9659258262890683122, 1.000000000000000000, 0.9659258262890683122, 1.000000000000000000, 0.9659258262890683122, 1.000000000000000000, 0.9659258262890683122, 1.000000000000000000, 0.9659258262890683122, 1.000000000000000000, 0.9659258262890683122, 1.000000000000000000 ) ) 
 REPRESENTATION_ITEM ( '' )  );
#96558=CARTESIAN_POINT ( 'NONE',  ( 115.8495968585647802, 6.109999999999997655, 1.637169565754163836 ) ) ;
#96584=AXIS2_PLACEMENT_3D ( 'NONE', #77155, #111142, #23441 ) ;
#96596=CARTESIAN_POINT ( 'NONE',  ( 34.47459685856478018, 1.637169565754164280, -6.109999999999997655 ) ) ;
#96622=CARTESIAN_POINT ( 'NONE',  ( 59.14169371712955581, -2.130196079827424871, -7.949999999999999289 ) ) ;
#96628=CARTESIAN_POINT ( 'NONE',  ( 56.70833333333333570, -3.974999999999999201, -6.884901960086287964 ) ) ;
#96636=CARTESIAN_POINT ( 'NONE',  ( 52.06293019189809712, 1.637169565754157174, 6.110000000000002984 ) ) ;
#96650=CARTESIAN_POINT ( 'NONE',  ( 85.75043019189810423, 3.055000000000002824, -5.291415217122919401 ) ) ;
#96660=CARTESIAN_POINT ( 'NONE',  ( 64.37043019189810877, -3.055000000000001492, 5.291415217122917625 ) ) ;
#96686=CYLINDRICAL_SURFACE ( 'NONE', #126715, 7.950000000000000178 ) ;
#96688=EDGE_LOOP ( 'NONE', ( #114579, #27818, #61164, #54469 ) ) ;
#96694=CARTESIAN_POINT ( 'NONE',  ( 84.34959685856478018, 6.109999999999996767, 1.637169565754163836 ) ) ;
#96695=VERTEX_POINT ( 'NONE', #126277 ) ;
#96716=ORIENTED_EDGE ( 'NONE', *, *, #103670, .F. ) ;
#96717=CARTESIAN_POINT ( 'NONE',  ( 39.37543019189809712, -5.291415217122920289, -3.055000000000001492 ) ) ;
#96728=DIRECTION ( 'NONE',  ( -1.000000000000000000, -0.000000000000000000, -0.000000000000000000 ) ) ;
#96739=PRODUCT ( '1.2 Vise Screw', '1.2 Vise Screw', '', ( #17713 ) ) ;
#96747=CARTESIAN_POINT ( 'NONE',  ( 150.3000000000000114, 7.776507174585691177E-16, -6.349999999999997868 ) ) ;
#96763=CARTESIAN_POINT ( 'NONE',  ( 61.45376352523145158, -6.109999999999999432, -3.741295971395163529E-16 ) ) ;
#96795=CARTESIAN_POINT ( 'NONE',  ( 82.47502705046287019, -5.819803920172572198, 5.819803920172572198 ) ) ;
#96811=CARTESIAN_POINT ( 'NONE',  ( 73.64626352523141861, -4.472830434245840259, 4.472830434245839371 ) ) ;
#96832=CARTESIAN_POINT ( 'NONE',  ( 74.95876352523143282, 0.000000000000000000, -6.110000000000001208 ) ) ;
#96854=CARTESIAN_POINT ( 'NONE',  ( 128.0136022459138303, -6.349999999999999645, -3.888253587292846081E-16 ) ) ;
#96868=CARTESIAN_POINT ( 'NONE',  ( 68.32919371712955581, -3.975000000000001865, 6.884901960086284411 ) ) ;
#96872=CARTESIAN_POINT ( 'NONE',  ( 58.41252705046289151, -7.949999999999998401, -4.867971026610728450E-16 ) ) ;
#96888=CARTESIAN_POINT ( 'NONE',  ( 65.33376352523143282, 6.110000000000001208, 1.122388791418549305E-15 ) ) ;
#96895=CARTESIAN_POINT ( 'NONE',  ( 103.5420968585647756, 5.291415217122923842, -3.054999999999996163 ) ) ;
#96910=CARTESIAN_POINT ( 'NONE',  ( 125.1829301918981372, -1.637169565754158951, -6.109999999999998543 ) ) ;
#96938=CARTESIAN_POINT ( 'NONE',  ( 34.27126352523143993, 4.472830434245839371, 4.472830434245842035 ) ) ;
#96946=DIRECTION ( 'NONE',  ( 0.000000000000000000, 0.000000000000000000, 1.000000000000000000 ) ) ;
#96955=CARTESIAN_POINT ( 'NONE',  ( 92.68336038379624142, -2.130196079827426203, 7.949999999999996625 ) ) ;
#96956=CARTESIAN_POINT ( 'NONE',  ( 125.7875270504628986, 0.000000000000000000, -7.949999999999998401 ) ) ;
#96974=EDGE_CURVE ( 'NONE', #20610, #79882, #4652, .T. ) ;
#96985=CARTESIAN_POINT ( 'NONE',  ( 92.14583333333334281, 2.130196079827431976, -7.949999999999998401 ) ) ;
#96989=CARTESIAN_POINT ( 'NONE',  ( 39.64583333333332149, 2.130196079827356037, -7.950000000000043698 ) ) ;
#96998=CARTESIAN_POINT ( 'NONE',  ( 101.9379301918980900, -6.110000000000001208, 1.637169565754158951 ) ) ;
#97004=CARTESIAN_POINT ( 'NONE',  ( 75.37500000000000000, 7.950000000000000178, 1.460391307983218535E-15 ) ) ;
#97007=CARTESIAN_POINT ( 'NONE',  ( 95.72459685856476597, -1.637169565754160949, 6.109999999999997655 ) ) ;
#97054=CARTESIAN_POINT ( 'NONE',  ( 28.93293019189811943, 1.637169565754156508, 6.110000000000000320 ) ) ;
#97082=ADVANCED_FACE ( 'NONE', ( #63559 ), #73982, .T. ) ;
#97092=ORIENTED_EDGE ( 'NONE', *, *, #64493, .T. ) ;
#97093=CARTESIAN_POINT ( 'NONE',  ( 94.55793019189810877, 6.110000000000001208, -1.637169565754156286 ) ) ;
#97133=CARTESIAN_POINT ( 'NONE',  ( 31.91666666666666430, -6.884901960086287076, -3.975000000000000977 ) ) ;
#97148=CARTESIAN_POINT ( 'NONE',  ( 106.2916666666666714, 3.975000000000003642, -6.884901960086285300 ) ) ;
#97160=CARTESIAN_POINT ( 'NONE',  ( 107.0420968585647756, 5.291415217122923842, -3.054999999999996163 ) ) ;
#97168=CARTESIAN_POINT ( 'NONE',  ( 28.80836038379621655, 7.949999999999997513, 2.130196079827431088 ) ) ;
#97173=CARTESIAN_POINT ( 'NONE',  ( 29.29166666666666075, 3.975000000000003642, -6.884901960086285300 ) ) ;
#97183=CARTESIAN_POINT ( 'NONE',  ( 119.6412635252314658, 4.472830434245836706, 4.472830434245840259 ) ) ;
#97189=CARTESIAN_POINT ( 'NONE',  ( 70.22502705046288440, 5.819803920172573974, -5.819803920172573086 ) ) ;
#97198=CARTESIAN_POINT ( 'NONE',  ( 43.31293019189810423, -1.637169565754159617, -6.110000000000001208 ) ) ;
#97207=CARTESIAN_POINT ( 'NONE',  ( 43.51626352523143737, -4.472830434245839371, 4.472830434245839371 ) ) ;
#97237=CARTESIAN_POINT ( 'NONE',  ( 57.80793019189810877, -6.109999999999998543, 1.637169565754158507 ) ) ;
#97260=EDGE_CURVE ( 'NONE', #66284, #87171, #118603, .T. ) ;
#97269=CARTESIAN_POINT ( 'NONE',  ( 122.7037635252314516, 6.109999999999999432, 1.122388791418549108E-15 ) ) ;
#97275=CARTESIAN_POINT ( 'NONE',  ( 66.43336038379622721, 2.130196079827431532, -7.949999999999996625 ) ) ;
#97314=CARTESIAN_POINT ( 'NONE',  ( 38.12043019189811588, 3.055000000000002380, -5.291415217122917625 ) ) ;
#97334=CARTESIAN_POINT ( 'NONE',  ( 81.64583333333330017, 2.130196079827356037, -7.950000000000043698 ) ) ;
#97346=CARTESIAN_POINT ( 'NONE',  ( 56.51669371712956291, 7.950000000000001066, -2.130196079827421318 ) ) ;
#97352=CARTESIAN_POINT ( 'NONE',  ( 58.31249999999997868, 5.819803920172571310, 5.819803920172575751 ) ) ;
#97361=CARTESIAN_POINT ( 'NONE',  ( 51.91709685856476852, 3.054999999999998828, 5.291415217122922066 ) ) ;
#97377=CARTESIAN_POINT ( 'NONE',  ( 86.62543019189811844, 5.291415217122919401, 3.055000000000002824 ) ) ;
#97387=CARTESIAN_POINT ( 'NONE',  ( 88.30836038379621300, 7.949999999999996625, 2.130196079827431088 ) ) ;
#97388=CARTESIAN_POINT ( 'NONE',  ( 69.91209685856478018, 5.291415217122921177, -3.054999999999994831 ) ) ;
#97410=( BOUNDED_CURVE ( )  B_SPLINE_CURVE ( 2, ( #124209, #14733, #50943, #37937, #115426, #83581, #95134, #92272, #94420, #114735, #71276, #59688, #29174 ),
 .UNSPECIFIED., .F., .F. ) 
 B_SPLINE_CURVE_WITH_KNOTS ( ( 3, 2, 2, 2, 2, 2, 3 ),
 ( 0.2333333333333332815, 0.2361111111111110494, 0.2388888888888888451, 0.2416666666666666130, 0.2444444444444443809, 0.2472222222222221766, 0.2499999999999999445 ),
 .UNSPECIFIED. ) 
 CURVE ( )  GEOMETRIC_REPRESENTATION_ITEM ( )  RATIONAL_B_SPLINE_CURVE ( ( 1.000000000000000666, 0.9659258262890676461, 1.000000000000000000, 0.9659258262890683122, 1.000000000000000000, 0.9659258262890683122, 1.000000000000000000, 0.9659258262890683122, 1.000000000000000000, 0.9659258262890683122, 1.000000000000000000, 0.9659258262890689783, 0.9999999999999993339 ) ) 
 REPRESENTATION_ITEM ( '' )  );
#97424=CARTESIAN_POINT ( 'NONE',  ( 83.18293019189810877, -1.637169565754158951, -6.109999999999998543 ) ) ;
#97447=CARTESIAN_POINT ( 'NONE',  ( 123.4541937171295700, 6.884901960086283523, 3.975000000000002753 ) ) ;
#97454=ORIENTED_EDGE ( 'NONE', *, *, #24678, .F. ) ;
#97455=CARTESIAN_POINT ( 'NONE',  ( 39.52126352523143282, -4.472830434245838482, -4.472830434245840259 ) ) ;
#97477=CARTESIAN_POINT ( 'NONE',  ( 109.8916937171295558, 2.130196079827421762, 7.950000000000000178 ) ) ;
#97487=CARTESIAN_POINT ( 'NONE',  ( 118.7875270504628986, 0.000000000000000000, -7.949999999999998401 ) ) ;
#97489=CARTESIAN_POINT ( 'NONE',  ( 96.62086038379621300, -6.884901960086286188, 3.974999999999997424 ) ) ;
#97507=CARTESIAN_POINT ( 'NONE',  ( 68.01626352523145158, -4.472830434245839371, 4.472830434245839371 ) ) ;
#97520=VECTOR ( 'NONE', #51018, 1000.000000000000000 ) ;
#97541=CARTESIAN_POINT ( 'NONE',  ( 86.41252705046289861, -7.949999999999998401, -4.867971026610728450E-16 ) ) ;
#97555=CARTESIAN_POINT ( 'NONE',  ( 75.39626352523141861, 4.472830434245840259, -4.472830434245839371 ) ) ;
#97575=CARTESIAN_POINT ( 'NONE',  ( 62.56293019189811133, 1.637169565754157174, 6.110000000000002984 ) ) ;
#97602=CARTESIAN_POINT ( 'NONE',  ( 114.5370968585647802, -3.054999999999998828, -5.291415217122919401 ) ) ;
#97636=CARTESIAN_POINT ( 'NONE',  ( 60.52126352523143282, -4.472830434245838482, -4.472830434245840259 ) ) ;
#97643=CARTESIAN_POINT ( 'NONE',  ( 98.29209685856477563, -5.291415217122921177, 3.054999999999999272 ) ) ;
#97651=CARTESIAN_POINT ( 'NONE',  ( 90.97916666666667140, -7.950000000000000178, 2.130196079827424427 ) ) ;
#97662=CARTESIAN_POINT ( 'NONE',  ( 119.0579301918981230, 6.110000000000000320, -1.637169565754156064 ) ) ;
#97664=VECTOR ( 'NONE', #5528, 1000.000000000000000 ) ;
#97691=CARTESIAN_POINT ( 'NONE',  ( 28.58376352523143993, -6.110000000000001208, -3.741295971395164515E-16 ) ) ;
#97713=CARTESIAN_POINT ( 'NONE',  ( 108.8708603837962272, 6.884901960086289741, -3.974999999999993427 ) ) ;
#97734=CARTESIAN_POINT ( 'NONE',  ( 90.93336038379622721, 2.130196079827431532, -7.949999999999996625 ) ) ;
#97744=CARTESIAN_POINT ( 'NONE',  ( 92.87500000000000000, 7.950000000000000178, 1.460391307983218535E-15 ) ) ;
#97757=CARTESIAN_POINT ( 'NONE',  ( 92.31293019189811844, -1.637169565754159617, -6.110000000000001208 ) ) ;
#97766=CARTESIAN_POINT ( 'NONE',  ( 93.24543019189812298, -5.291415217122918513, -3.055000000000000160 ) ) ;
#97771=CARTESIAN_POINT ( 'NONE',  ( 116.2083333333333286, -3.974999999999999201, -6.884901960086287964 ) ) ;
#97777=EDGE_CURVE ( 'NONE', #143427, #112319, #103761, .T. ) ;
#97791=B_SPLINE_CURVE_WITH_KNOTS ( 'NONE', 3,
 ( #40421, #7746, #49158, #17891, #139010, #17217, #128826, #51997, #85308, #94752, #82485, #61479, #29503, #73736 ),
 .UNSPECIFIED., .F., .F.,
 ( 4, 2, 2, 2, 2, 2, 4 ),
 ( 1.498279533920597479E-16, 0.001332397885839088636, 0.001998596828758557493, 0.002664795771678026351, 0.003997193657516964933, 0.004663392600436432923, 0.005329591543355900914 ),
 .UNSPECIFIED. ) ;
#97798=DIRECTION ( 'NONE',  ( -1.000000000000000000, -0.000000000000000000, -0.000000000000000000 ) ) ;
#97800=CARTESIAN_POINT ( 'NONE',  ( 120.0000000000000000, 0.000000000000000000, -7.950000000000000178 ) ) ;
#97860=CARTESIAN_POINT ( 'NONE',  ( 96.16209685856478018, -5.291415217122919401, 3.054999999999998384 ) ) ;
#97879=ORIENTED_EDGE ( 'NONE', *, *, #68126, .T. ) ;
#97884=ORIENTED_EDGE ( 'NONE', *, *, #48408, .F. ) ;
#97897=CARTESIAN_POINT ( 'NONE',  ( 113.0000000000000000, 0.000000000000000000, -7.950000000000000178 ) ) ;
#97912=CARTESIAN_POINT ( 'NONE',  ( 104.8333333333333286, -6.884901960086287964, 3.974999999999998312 ) ) ;
#97933=CARTESIAN_POINT ( 'NONE',  ( 30.26669371712955581, -7.949999999999999289, 2.130196079827424427 ) ) ;
#97937=CARTESIAN_POINT ( 'NONE',  ( 27.97916666666666430, -7.950000000000001066, 2.130196079827424427 ) ) ;
#97948=CARTESIAN_POINT ( 'NONE',  ( 127.3704301918981088, -3.055000000000001492, 5.291415217122917625 ) ) ;
#97959=CARTESIAN_POINT ( 'NONE',  ( 44.33376352523143993, 6.110000000000001208, 1.122388791418549305E-15 ) ) ;
#97968=CARTESIAN_POINT ( 'NONE',  ( 43.07876352523144448, -7.482591942790325086E-16, 6.109999999999998543 ) ) ;
#97976=CARTESIAN_POINT ( 'NONE',  ( 78.97502705046288440, -5.819803920172573086, 5.819803920172573086 ) ) ;
#97988=ORIENTED_EDGE ( 'NONE', *, *, #122637, .F. ) ;
#97994=CARTESIAN_POINT ( 'NONE',  ( 58.97459685856478018, 1.637169565754164280, -6.109999999999996767 ) ) ;
#97997=( BOUNDED_CURVE ( )  B_SPLINE_CURVE ( 2, ( #82565, #54079, #119970, #115146, #98267, #126755, #141783, #41739, #130189, #119277, #15819, #37651, #71699 ),
 .UNSPECIFIED., .F., .T. ) 
 B_SPLINE_CURVE_WITH_KNOTS ( ( 3, 2, 2, 2, 2, 2, 3 ),
 ( 0.1833333333333333481, 0.1861111111111111438, 0.1888888888888889117, 0.1916666666666667074, 0.1944444444444444753, 0.1972222222222222432, 0.2000000000000000389 ),
 .UNSPECIFIED. ) 
 CURVE ( )  GEOMETRIC_REPRESENTATION_ITEM ( )  RATIONAL_B_SPLINE_CURVE ( ( 0.9999999999999996669, 0.9659258262890686453, 1.000000000000000000, 0.9659258262890683122, 1.000000000000000000, 0.9659258262890683122, 1.000000000000000000, 0.9659258262890683122, 1.000000000000000000, 0.9659258262890683122, 1.000000000000000000, 0.9659258262890679791, 1.000000000000000444 ) ) 
 REPRESENTATION_ITEM ( '' )  );
#98036=CARTESIAN_POINT ( 'NONE',  ( 120.8079301918980946, -6.109999999999999432, 1.637169565754158507 ) ) ;
#98074=CARTESIAN_POINT ( 'NONE',  ( 34.62043019189811588, 3.055000000000002380, -5.291415217122917625 ) ) ;
#98103=CARTESIAN_POINT ( 'NONE',  ( 55.78752705046288440, 0.000000000000000000, -7.949999999999998401 ) ) ;
#98108=CARTESIAN_POINT ( 'NONE',  ( 52.91666666666666430, -6.884901960086287076, -3.975000000000000977 ) ) ;
#98116=CARTESIAN_POINT ( 'NONE',  ( 47.39626352523143282, 4.472830434245840259, -4.472830434245839371 ) ) ;
#98133=CARTESIAN_POINT ( 'NONE',  ( 80.35459685856476142, -1.637169565754161615, 6.110000000000000320 ) ) ;
#98144=CARTESIAN_POINT ( 'NONE',  ( 68.59959685856476597, -6.109999999999997655, -1.637169565754160283 ) ) ;
#98172=CARTESIAN_POINT ( 'NONE',  ( 80.41209685856479439, 5.291415217122921177, -3.054999999999994831 ) ) ;
#98175=EDGE_CURVE ( 'NONE', #96223, #135001, #74292, .T. ) ;
#98180=CARTESIAN_POINT ( 'NONE',  ( 0.000000000000000000, 9.735942053221458872E-16, -7.950000000000000178 ) ) ;
#98189=CARTESIAN_POINT ( 'NONE',  ( 123.6000270504628844, 5.819803920172570422, 5.819803920172575751 ) ) ;
#98198=CARTESIAN_POINT ( 'NONE',  ( 32.52126352523143282, -4.472830434245838482, -4.472830434245840259 ) ) ;
#98252=CARTESIAN_POINT ( 'NONE',  ( 69.32876352523145158, 0.000000000000000000, -6.109999999999999432 ) ) ;
#98253=VECTOR ( 'NONE', #66450, 1000.000000000000000 ) ;
#98257=CARTESIAN_POINT ( 'NONE',  ( 83.83333333333332860, -6.884901960086287964, 3.974999999999998312 ) ) ;
#98263=EDGE_LOOP ( 'NONE', ( #23255, #4104 ) ) ;
#98267=CARTESIAN_POINT ( 'NONE',  ( 107.1666666666666572, 6.884901960086285300, 3.975000000000003642 ) ) ;
#98272=CARTESIAN_POINT ( 'NONE',  ( 127.1386022459138019, -7.776507174585692163E-16, 6.349999999999999645 ) ) ;
#98278=CARTESIAN_POINT ( 'NONE',  ( 83.64169371712955581, -2.130196079827424871, -7.949999999999999289 ) ) ;
#98283=CARTESIAN_POINT ( 'NONE',  ( 86.45833333333332860, 3.974999999999997424, 6.884901960086288852 ) ) ;
#98294=CARTESIAN_POINT ( 'NONE',  ( 71.45876352523143282, 0.000000000000000000, -6.110000000000001208 ) ) ;
#98314=CARTESIAN_POINT ( 'NONE',  ( 69.12543019189809002, 5.291415217122919401, 3.055000000000002824 ) ) ;
#98322=DIRECTION ( 'NONE',  ( -1.000000000000000000, -0.000000000000000000, -0.000000000000000000 ) ) ;
#98335=ORIENTED_EDGE ( 'NONE', *, *, #131079, .F. ) ;
#98339=CARTESIAN_POINT ( 'NONE',  ( 60.79166666666665719, 3.975000000000003642, -6.884901960086285300 ) ) ;
#98346=CARTESIAN_POINT ( 'NONE',  ( 108.9954301918981088, 5.291415217122916737, 3.055000000000001936 ) ) ;
#98371=CARTESIAN_POINT ( 'NONE',  ( 68.39626352523143282, 4.472830434245840259, -4.472830434245838482 ) ) ;
#98376=CARTESIAN_POINT ( 'NONE',  ( 100.0420968585647756, 5.291415217122923842, -3.054999999999996163 ) ) ;
#98393=CARTESIAN_POINT ( 'NONE',  ( 121.8287635252314516, 0.000000000000000000, -6.109999999999998543 ) ) ;
#98408=CARTESIAN_POINT ( 'NONE',  ( 10.32500000000000107, -8.432637487761466488, -4.375000000000001776 ) ) ;
#98415=FACE_OUTER_BOUND ( 'NONE', #14826, .T. ) ;
#98416=CARTESIAN_POINT ( 'NONE',  ( 29.02126352523143282, -4.472830434245839371, -4.472830434245840259 ) ) ;
#98430=DIRECTION ( 'NONE',  ( -1.000000000000000000, -0.000000000000000000, -0.000000000000000000 ) ) ;
#98434=CARTESIAN_POINT ( 'NONE',  ( 113.3916937171295700, 2.130196079827421762, 7.950000000000001066 ) ) ;
#98444=ORIENTED_EDGE ( 'NONE', *, *, #104833, .F. ) ;
#98450=EDGE_LOOP ( 'NONE', ( #82172, #126849, #50345, #107741 ) ) ;
#98471=CARTESIAN_POINT ( 'NONE',  ( 93.04209685856476142, 5.291415217122923842, -3.054999999999996163 ) ) ;
#98481=CARTESIAN_POINT ( 'NONE',  ( 89.74543019189812298, -5.291415217122918513, -3.055000000000000160 ) ) ;
#98531=CARTESIAN_POINT ( 'NONE',  ( 123.9587635252314470, 0.000000000000000000, -6.110000000000001208 ) ) ;
#98560=CARTESIAN_POINT ( 'NONE',  ( 92.22459685856479439, -1.637169565754161171, 6.109999999999998543 ) ) ;
#98605=CARTESIAN_POINT ( 'NONE',  ( 110.9583333333333286, 3.974999999999997424, 6.884901960086288852 ) ) ;
#98609=CARTESIAN_POINT ( 'NONE',  ( 97.25000000000000000, -9.735942053221458872E-16, 7.950000000000000178 ) ) ;
#98622=CARTESIAN_POINT ( 'NONE',  ( 25.02392480454907187, -6.350000000000004974, -3.888253587292851012E-16 ) ) ;
#98628=CARTESIAN_POINT ( 'NONE',  ( 27.05836038379621655, -7.949999999999997513, -2.130196079827425759 ) ) ;
#98634=ORIENTED_EDGE ( 'NONE', *, *, #62571, .T. ) ;
#98635=CARTESIAN_POINT ( 'NONE',  ( 116.5212635252314328, -4.472830434245839371, -4.472830434245840259 ) ) ;
#98648=CARTESIAN_POINT ( 'NONE',  ( 114.5370968585647802, -3.054999999999998828, -5.291415217122919401 ) ) ;
#98651=CARTESIAN_POINT ( 'NONE',  ( 71.39169371712955581, 2.130196079827421762, 7.950000000000000178 ) ) ;
#98655=CARTESIAN_POINT ( 'NONE',  ( 34.85459685856477563, -1.637169565754161615, 6.110000000000000320 ) ) ;
#98661=CIRCLE ( 'NONE', #6105, 4.749999999999997335 ) ;
#98662=CARTESIAN_POINT ( 'NONE',  ( 40.01626352523144448, -4.472830434245839371, 4.472830434245839371 ) ) ;
#98692=CARTESIAN_POINT ( 'NONE',  ( 44.09959685856477307, -6.109999999999997655, -1.637169565754160283 ) ) ;
#98697=VERTEX_POINT ( 'NONE', #40065 ) ;
#98724=CARTESIAN_POINT ( 'NONE',  ( 117.0162635252314374, -4.472830434245839371, 4.472830434245839371 ) ) ;
#98737=EDGE_CURVE ( 'NONE', #74867, #121255, #18989, .T. ) ;
#98750=DIRECTION ( 'NONE',  ( 0.000000000000000000, 0.000000000000000000, 1.000000000000000000 ) ) ;
#98762=CARTESIAN_POINT ( 'NONE',  ( 36.51626352523145158, -4.472830434245839371, 4.472830434245839371 ) ) ;
#98766=CARTESIAN_POINT ( 'NONE',  ( 126.8541666666666572, -2.130196079827425315, -7.950000000000001066 ) ) ;
#98778=CARTESIAN_POINT ( 'NONE',  ( 120.3129301918980758, -1.637169565754159617, -6.110000000000001208 ) ) ;
#98782=CARTESIAN_POINT ( 'NONE',  ( 78.14583333333332860, 2.130196079827431976, -7.949999999999998401 ) ) ;
#98789=CARTESIAN_POINT ( 'NONE',  ( 60.01669371712956291, 7.950000000000001066, -2.130196079827421318 ) ) ;
#98795=CARTESIAN_POINT ( 'NONE',  ( 41.54166666666665719, -3.975000000000002753, 6.884901960086286188 ) ) ;
#98805=CARTESIAN_POINT ( 'NONE',  ( 46.52126352523142572, -4.472830434245839371, -4.472830434245840259 ) ) ;
#98821=CARTESIAN_POINT ( 'NONE',  ( 78.45876352523144703, 0.000000000000000000, -6.110000000000001208 ) ) ;
#98831=( BOUNDED_CURVE ( )  B_SPLINE_CURVE ( 2, ( #137204, #47382, #16075, #60371, #91551, #125616, #104551, #16839, #14696, #26294, #103130, #70552, #127753 ),
 .UNSPECIFIED., .F., .T. ) 
 B_SPLINE_CURVE_WITH_KNOTS ( ( 3, 2, 2, 2, 2, 2, 3 ),
 ( 0.01666666666666668031, 0.01944444444444446210, 0.02222222222222224042, 0.02500000000000002220, 0.02777777777777779705, 0.03055555555555557884, 0.03333333333333336063 ),
 .UNSPECIFIED. ) 
 CURVE ( )  GEOMETRIC_REPRESENTATION_ITEM ( )  RATIONAL_B_SPLINE_CURVE ( ( 0.9999999999999997780, 0.9659258262890685343, 1.000000000000000000, 0.9659258262890683122, 1.000000000000000000, 0.9659258262890683122, 1.000000000000000000, 0.9659258262890683122, 1.000000000000000000, 0.9659258262890683122, 1.000000000000000000, 0.9659258262890679791, 1.000000000000000444 ) ) 
 REPRESENTATION_ITEM ( '' )  );
#98833=CARTESIAN_POINT ( 'NONE',  ( 65.82876352523145158, 0.000000000000000000, -6.109999999999998543 ) ) ;
#98838=VERTEX_POINT ( 'NONE', #776 ) ;
#98858=CARTESIAN_POINT ( 'NONE',  ( 75.89126352523143737, -4.472830434245838482, -4.472830434245838482 ) ) ;
#98882=CARTESIAN_POINT ( 'NONE',  ( 36.45876352523143282, 0.000000000000000000, -6.110000000000001208 ) ) ;
#98936=CARTESIAN_POINT ( 'NONE',  ( 68.74543019189812298, -5.291415217122919401, -3.055000000000000604 ) ) ;
#98955=CARTESIAN_POINT ( 'NONE',  ( 90.78752705046288440, 0.000000000000000000, -7.949999999999998401 ) ) ;
#98958=CARTESIAN_POINT ( 'NONE',  ( 88.45419371712957002, 6.884901960086283523, 3.975000000000002753 ) ) ;
#98964=CARTESIAN_POINT ( 'NONE',  ( 81.35416666666667140, -2.130196079827425315, -7.950000000000001066 ) ) ;
#98976=CARTESIAN_POINT ( 'NONE',  ( 73.20876352523143282, -7.482591942790329030E-16, 6.110000000000001208 ) ) ;
#98979=DIRECTION ( 'NONE',  ( -0.000000000000000000, 0.000000000000000000, 1.000000000000000000 ) ) ;
#98998=CARTESIAN_POINT ( 'NONE',  ( 60.37543019189810423, -5.291415217122920289, -3.055000000000001492 ) ) ;
#99002=CARTESIAN_POINT ( 'NONE',  ( 125.2041937171295700, -6.884901960086285300, -3.975000000000000089 ) ) ;
#99004=ORIENTED_EDGE ( 'NONE', *, *, #84884, .F. ) ;
#99027=CARTESIAN_POINT ( 'NONE',  ( 117.1620968585647802, -5.291415217122919401, 3.054999999999997939 ) ) ;
#99034=CARTESIAN_POINT ( 'NONE',  ( 68.03752705046289861, -9.735942053221456900E-16, 7.949999999999998401 ) ) ;
#99046=CARTESIAN_POINT ( 'NONE',  ( 63.58376352523143993, -6.110000000000001208, -3.741295971395164515E-16 ) ) ;
#99051=CARTESIAN_POINT ( 'NONE',  ( 101.9379301918980900, -6.110000000000001208, 1.637169565754158951 ) ) ;
#99064=CARTESIAN_POINT ( 'NONE',  ( 125.7662635252314658, 4.472830434245838482, -4.472830434245837594 ) ) ;
#99100=( BOUNDED_CURVE ( )  B_SPLINE_CURVE ( 2, ( #130363, #18699, #42653, #62978, #120141, #107153, #140495, #84701, #43346, #86134, #40502, #96955, #119438 ),
 .UNSPECIFIED., .F., .T. ) 
 B_SPLINE_CURVE_WITH_KNOTS ( ( 3, 2, 2, 2, 2, 2, 3 ),
 ( 0.3333333333333333148, 0.3361111111111111382, 0.3388888888888889062, 0.3416666666666666741, 0.3444444444444444420, 0.3472222222222222099, 0.3499999999999999778 ),
 .UNSPECIFIED. ) 
 CURVE ( )  GEOMETRIC_REPRESENTATION_ITEM ( )  RATIONAL_B_SPLINE_CURVE ( ( 1.000000000000000000, 0.9659258262890683122, 1.000000000000000000, 0.9659258262890683122, 1.000000000000000000, 0.9659258262890683122, 1.000000000000000000, 0.9659258262890683122, 1.000000000000000000, 0.9659258262890683122, 1.000000000000000000, 0.9659258262890683122, 1.000000000000000000 ) ) 
 REPRESENTATION_ITEM ( '' )  );
#99103=CARTESIAN_POINT ( 'NONE',  ( 42.85416666666666430, -2.130196079827425759, -7.950000000000000178 ) ) ;
#99113=CARTESIAN_POINT ( 'NONE',  ( 109.6000270504628844, 5.819803920172570422, 5.819803920172574863 ) ) ;
#99114=CARTESIAN_POINT ( 'NONE',  ( 153.6500000000000057, 0.000000000000000000, 0.000000000000000000 ) ) ;
#99153=CARTESIAN_POINT ( 'NONE',  ( 96.10459685856477563, 1.637169565754164946, -6.109999999999999432 ) ) ;
#99162=CARTESIAN_POINT ( 'NONE',  ( 49.41666666666666430, -6.884901960086287076, -3.975000000000000977 ) ) ;
#99163=CARTESIAN_POINT ( 'NONE',  ( 87.41209685856478018, 5.291415217122921177, -3.054999999999994831 ) ) ;
#99166=CARTESIAN_POINT ( 'NONE',  ( 115.6250000000000000, -7.950000000000000178, -4.867971026610729436E-16 ) ) ;
#99197=DIRECTION ( 'NONE',  ( 0.000000000000000000, 0.000000000000000000, 1.000000000000000000 ) ) ;
#99198=CARTESIAN_POINT ( 'NONE',  ( 119.4166666666666714, -6.884901960086287076, -3.975000000000000977 ) ) ;
#99205=ORIENTED_EDGE ( 'NONE', *, *, #10608, .T. ) ;
#99206=CARTESIAN_POINT ( 'NONE',  ( 115.4333603837962130, 2.130196079827431532, -7.949999999999996625 ) ) ;
#99217=CARTESIAN_POINT ( 'NONE',  ( 123.3754301918981184, -5.291415217122920289, -3.055000000000001492 ) ) ;
#99236=CARTESIAN_POINT ( 'NONE',  ( 107.1208603837962272, -6.884901960086286188, 3.974999999999997424 ) ) ;
#99244=EDGE_CURVE ( 'NONE', #46491, #94937, #141920, .T. ) ;
#99248=CARTESIAN_POINT ( 'NONE',  ( 81.57876352523143737, -7.482591942790327058E-16, 6.109999999999999432 ) ) ;
#99260=ORIENTED_EDGE ( 'NONE', *, *, #114098, .F. ) ;
#99303=CARTESIAN_POINT ( 'NONE',  ( 103.0833333333333286, 6.884901960086290629, -3.974999999999994316 ) ) ;
#99332=CARTESIAN_POINT ( 'NONE',  ( 123.8129301918981184, -1.637169565754159617, -6.110000000000001208 ) ) ;
#99342=CARTESIAN_POINT ( 'NONE',  ( 111.0370968585647944, -3.054999999999998828, -5.291415217122919401 ) ) ;
#99348=CARTESIAN_POINT ( 'NONE',  ( 38.20876352523143282, -7.482591942790329030E-16, 6.110000000000001208 ) ) ;
#99355=CARTESIAN_POINT ( 'NONE',  ( 32.43293019189810877, 1.637169565754156508, 6.110000000000000320 ) ) ;
#99361=EDGE_CURVE ( 'NONE', #5013, #10004, #70911, .T. ) ;
#99384=CARTESIAN_POINT ( 'NONE',  ( 44.68293019189811588, -1.637169565754158951, -6.109999999999998543 ) ) ;
#99426=CARTESIAN_POINT ( 'NONE',  ( 112.6412635252314658, 4.472830434245837594, 4.472830434245841147 ) ) ;
#99434=ORIENTED_EDGE ( 'NONE', *, *, #88489, .T. ) ;
#99438=CARTESIAN_POINT ( 'NONE',  ( 120.5833333333333286, 6.884901960086290629, -3.974999999999994316 ) ) ;
#99454=EDGE_CURVE ( 'NONE', #75066, #139700, #97791, .T. ) ;
#99464=CARTESIAN_POINT ( 'NONE',  ( 27.03709685856478373, -3.054999999999999272, -5.291415217122919401 ) ) ;
#99484=CARTESIAN_POINT ( 'NONE',  ( 118.1254301918981184, 5.291415217122919401, 3.055000000000002824 ) ) ;
#99493=CARTESIAN_POINT ( 'NONE',  ( 56.80836038379622721, 7.949999999999997513, 2.130196079827431088 ) ) ;
#99499=CARTESIAN_POINT ( 'NONE',  ( 45.33333333333332149, -6.884901960086287964, 3.974999999999998312 ) ) ;
#99508=CARTESIAN_POINT ( 'NONE',  ( 35.72959685856475431, -6.110000000000000320, -1.637169565754161393 ) ) ;
#99525=CARTESIAN_POINT ( 'NONE',  ( 83.85459685856476142, -1.637169565754161615, 6.110000000000000320 ) ) ;
#99535=CARTESIAN_POINT ( 'NONE',  ( 64.80793019189812298, -6.109999999999998543, 1.637169565754158063 ) ) ;
#99558=CARTESIAN_POINT ( 'NONE',  ( 50.97502705046288440, -5.819803920172573086, 5.819803920172573086 ) ) ;
#99564=CARTESIAN_POINT ( 'NONE',  ( 72.24543019189810877, -5.291415217122918513, -3.055000000000000160 ) ) ;
#99571=CARTESIAN_POINT ( 'NONE',  ( 0.000000000000000000, 0.000000000000000000, 7.950000000000000178 ) ) ;
#99590=CARTESIAN_POINT ( 'NONE',  ( 27.56293019189810778, 1.637169565754157174, 6.110000000000002984 ) ) ;
#99594=CARTESIAN_POINT ( 'NONE',  ( 89.18336038379622721, -2.130196079827426203, 7.949999999999996625 ) ) ;
#99602=ORIENTED_EDGE ( 'NONE', *, *, #139695, .F. ) ;
#99621=CARTESIAN_POINT ( 'NONE',  ( 28.99999999999999645, 0.000000000000000000, -7.950000000000000178 ) ) ;
#99649=CARTESIAN_POINT ( 'NONE',  ( 52.47916666666665009, -7.950000000000000178, 2.130196079827424427 ) ) ;
#99651=CARTESIAN_POINT ( 'NONE',  ( 59.99543019189810877, 5.291415217122917625, 3.055000000000002380 ) ) ;
#99653=CARTESIAN_POINT ( 'NONE',  ( 0.000000000000000000, 0.000000000000000000, 0.000000000000000000 ) ) ;
#99655=CARTESIAN_POINT ( 'NONE',  ( 32.60002705046288440, 5.819803920172570422, 5.819803920172575751 ) ) ;
#99678=CARTESIAN_POINT ( 'NONE',  ( 87.43336038379624142, 2.130196079827431532, -7.949999999999997513 ) ) ;
#99683=CARTESIAN_POINT ( 'NONE',  ( 69.39583333333331439, -2.130196079827427091, 7.949999999999999289 ) ) ;
#99696=CARTESIAN_POINT ( 'NONE',  ( 62.56293019189811133, 1.637169565754157174, 6.110000000000002984 ) ) ;
#99703=FACE_OUTER_BOUND ( 'NONE', #22259, .T. ) ;
#99718=CARTESIAN_POINT ( 'NONE',  ( 67.81293019189807580, -1.637169565754159617, -6.110000000000001208 ) ) ;
#99752=CARTESIAN_POINT ( 'NONE',  ( 106.0787635252314516, -7.482591942790325086E-16, 6.109999999999998543 ) ) ;
#99777=CARTESIAN_POINT ( 'NONE',  ( 55.41709685856477563, 3.054999999999998828, 5.291415217122922066 ) ) ;
#99783=CARTESIAN_POINT ( 'NONE',  ( 88.66709685856477563, -3.055000000000000160, -5.291415217122921177 ) ) ;
#99803=CARTESIAN_POINT ( 'NONE',  ( 122.5579301918981088, 6.110000000000000320, -1.637169565754156064 ) ) ;
#99844=VECTOR ( 'NONE', #110708, 1000.000000000000000 ) ;
#99859=CARTESIAN_POINT ( 'NONE',  ( 112.2250270504628986, 5.819803920172573086, -5.819803920172572198 ) ) ;
#99860=CARTESIAN_POINT ( 'NONE',  ( 92.00000000000000000, 0.000000000000000000, -7.950000000000000178 ) ) ;
#99876=CARTESIAN_POINT ( 'NONE',  ( 105.0004301918981184, -3.055000000000002380, 5.291415217122920289 ) ) ;
#99899=CARTESIAN_POINT ( 'NONE',  ( 89.83376352523143282, 6.110000000000001208, 1.122388791418549305E-15 ) ) ;
#99904=CARTESIAN_POINT ( 'NONE',  ( 84.37086038379624142, 6.884901960086289741, -3.974999999999993427 ) ) ;
#99911=CARTESIAN_POINT ( 'NONE',  ( 87.26626352523145158, 4.472830434245839371, -4.472830434245838482 ) ) ;
#99934=ORIENTED_EDGE ( 'NONE', *, *, #32853, .F. ) ;
#99945=CARTESIAN_POINT ( 'NONE',  ( 55.78752705046288440, 0.000000000000000000, -7.949999999999998401 ) ) ;
#99951=CARTESIAN_POINT ( 'NONE',  ( 118.6874999999999716, -5.819803920172573974, 5.819803920172573086 ) ) ;
#99965=EDGE_CURVE ( 'NONE', #10004, #85083, #65404, .T. ) ;
#99987=ORIENTED_EDGE ( 'NONE', *, *, #84884, .T. ) ;
#100004=CARTESIAN_POINT ( 'NONE',  ( 84.34959685856478018, 6.109999999999997655, 1.637169565754163836 ) ) ;
#100057=VECTOR ( 'NONE', #14365, 1000.000000000000000 ) ;
#100059=CARTESIAN_POINT ( 'NONE',  ( 101.6250000000000000, -7.950000000000000178, -4.867971026610729436E-16 ) ) ;
#100076=VECTOR ( 'NONE', #111736, 1000.000000000000000 ) ;
#100079=CARTESIAN_POINT ( 'NONE',  ( 85.82919371712955581, -3.975000000000001865, 6.884901960086284411 ) ) ;
#100083=CARTESIAN_POINT ( 'NONE',  ( 116.9587635252314470, 0.000000000000000000, -6.110000000000001208 ) ) ;
#100091=CARTESIAN_POINT ( 'NONE',  ( 109.7245968585647660, -1.637169565754160949, 6.109999999999997655 ) ) ;
#100099=CARTESIAN_POINT ( 'NONE',  ( 40.25043019189809712, 3.055000000000002824, -5.291415217122919401 ) ) ;
#100108=CARTESIAN_POINT ( 'NONE',  ( 31.26626352523144092, 4.472830434245839371, -4.472830434245838482 ) ) ;
#100142=CARTESIAN_POINT ( 'NONE',  ( 49.64126352523144448, 4.472830434245835818, 4.472830434245840259 ) ) ;
#100166=CARTESIAN_POINT ( 'NONE',  ( 36.39169371712955581, 2.130196079827421762, 7.950000000000000178 ) ) ;
#100167=ORIENTED_EDGE ( 'NONE', *, *, #128286, .T. ) ;
#100180=CARTESIAN_POINT ( 'NONE',  ( 109.7245968585647660, -1.637169565754161171, 6.109999999999998543 ) ) ;
#100218=CARTESIAN_POINT ( 'NONE',  ( 28.64126352523144092, 4.472830434245837594, 4.472830434245841147 ) ) ;
#100235=CARTESIAN_POINT ( 'NONE',  ( 125.8545968585647756, -1.637169565754161615, 6.110000000000000320 ) ) ;
#100244=CARTESIAN_POINT ( 'NONE',  ( 49.80836038379622721, 7.949999999999997513, 2.130196079827431088 ) ) ;
#100250=CARTESIAN_POINT ( 'NONE',  ( 49.41666666666666430, -6.884901960086287076, -3.975000000000000977 ) ) ;
#100258=CARTESIAN_POINT ( 'NONE',  ( 38.35459685856476852, -1.637169565754161615, 6.110000000000000320 ) ) ;
#100286=CARTESIAN_POINT ( 'NONE',  ( 54.59959685856476597, -6.109999999999997655, -1.637169565754160283 ) ) ;
#100287=CARTESIAN_POINT ( 'NONE',  ( 48.78752705046289151, 0.000000000000000000, -7.949999999999998401 ) ) ;
#100315=CARTESIAN_POINT ( 'NONE',  ( 74.43293019189810877, 1.637169565754156508, 6.110000000000000320 ) ) ;
#100340=CARTESIAN_POINT ( 'NONE',  ( 25.95876352523143638, 0.000000000000000000, -6.110000000000001208 ) ) ;
#100368=CARTESIAN_POINT ( 'NONE',  ( 28.56249999999998934, -5.819803920172573086, -5.819803920172573974 ) ) ;
#100379=CARTESIAN_POINT ( 'NONE',  ( 25.16975813788240046, -6.350000000000002309, -1.701477371937631267 ) ) ;
#100396=CARTESIAN_POINT ( 'NONE',  ( 58.39126352523145158, -4.472830434245839371, -4.472830434245839371 ) ) ;
#100411=CARTESIAN_POINT ( 'NONE',  ( 106.5375270504628844, -9.735942053221456900E-16, 7.949999999999998401 ) ) ;
#100420=CARTESIAN_POINT ( 'NONE',  ( 71.97502705046289861, -5.819803920172572198, 5.819803920172572198 ) ) ;
#100425=CARTESIAN_POINT ( 'NONE',  ( 75.52083333333332860, 7.949999999999999289, 2.130196079827431532 ) ) ;
#100432=CARTESIAN_POINT ( 'NONE',  ( 68.97959685856477563, 6.109999999999999432, 1.637169565754164280 ) ) ;
#100438=CARTESIAN_POINT ( 'NONE',  ( 43.43749999999999289, 5.819803920172574863, -5.819803920172573086 ) ) ;
#100452=CARTESIAN_POINT ( 'NONE',  ( 67.66709685856477563, -3.055000000000000160, -5.291415217122921177 ) ) ;
#100470=CARTESIAN_POINT ( 'NONE',  ( 10.32500000000000107, -9.500000000000001776, 4.375000000000001776 ) ) ;
#100481=CARTESIAN_POINT ( 'NONE',  ( 0.000000000000000000, 0.000000000000000000, 0.000000000000000000 ) ) ;
#100490=CARTESIAN_POINT ( 'NONE',  ( 103.0162635252314374, -4.472830434245838482, 4.472830434245838482 ) ) ;
#100491=ORIENTED_EDGE ( 'NONE', *, *, #76799, .T. ) ;
#100514=CARTESIAN_POINT ( 'NONE',  ( 52.79209685856476852, -5.291415217122921177, 3.054999999999999272 ) ) ;
#100515=ORIENTED_EDGE ( 'NONE', *, *, #120721, .T. ) ;
#100520=CARTESIAN_POINT ( 'NONE',  ( 92.45876352523144703, 0.000000000000000000, -6.110000000000001208 ) ) ;
#100539=ADVANCED_FACE ( 'NONE', ( #13648 ), #81827, .T. ) ;
#100558=CARTESIAN_POINT ( 'NONE',  ( 57.29166666666665719, 3.975000000000003642, -6.884901960086285300 ) ) ;
#100588=CARTESIAN_POINT ( 'NONE',  ( 110.3291937171295700, -3.975000000000001865, 6.884901960086284411 ) ) ;
#100606=CARTESIAN_POINT ( 'NONE',  ( 95.08376352523144703, -6.110000000000001208, -3.741295971395164515E-16 ) ) ;
#100627=CARTESIAN_POINT ( 'NONE',  ( 93.62543019189811844, 5.291415217122919401, 3.055000000000002824 ) ) ;
#100641=CARTESIAN_POINT ( 'NONE',  ( 85.07876352523143737, -7.482591942790325086E-16, 6.109999999999998543 ) ) ;
#100690=CARTESIAN_POINT ( 'NONE',  ( 122.7920968585647756, -5.291415217122921177, 3.054999999999999272 ) ) ;
#100720=CARTESIAN_POINT ( 'NONE',  ( 85.95376352523145158, -6.109999999999999432, -3.741295971395163529E-16 ) ) ;
#100721=CARTESIAN_POINT ( 'NONE',  ( 9.748460325766547641, -8.447629293701412578, 4.346447159401130023 ) ) ;
#100732=CARTESIAN_POINT ( 'NONE',  ( 0.000000000000000000, 0.000000000000000000, 0.000000000000000000 ) ) ;
#100763=CARTESIAN_POINT ( 'NONE',  ( 102.0625000000000000, -5.819803920172572198, -5.819803920172573086 ) ) ;
#100769=CARTESIAN_POINT ( 'NONE',  ( 88.50000000000000000, 0.000000000000000000, -7.950000000000000178 ) ) ;
#100791=CARTESIAN_POINT ( 'NONE',  ( 120.1670968585647756, -3.055000000000000160, -5.291415217122921177 ) ) ;
#100801=CARTESIAN_POINT ( 'NONE',  ( 113.6620968585647944, -5.291415217122919401, 3.054999999999997939 ) ) ;
#100807=CARTESIAN_POINT ( 'NONE',  ( 38.35459685856476852, -1.637169565754161615, 6.110000000000000320 ) ) ;
#100822=LINE ( 'NONE', #12374, #129848 ) ;
#100844=CARTESIAN_POINT ( 'NONE',  ( 51.97459685856478728, 1.637169565754164280, -6.109999999999996767 ) ) ;
#100861=CARTESIAN_POINT ( 'NONE',  ( 35.80836038379622721, 7.949999999999996625, 2.130196079827431088 ) ) ;
#100874=CARTESIAN_POINT ( 'NONE',  ( 108.5579301918980946, 6.110000000000001208, -1.637169565754156286 ) ) ;
#100886=DIRECTION ( 'NONE',  ( 0.000000000000000000, 0.000000000000000000, -1.000000000000000000 ) ) ;
#100887=CARTESIAN_POINT ( 'NONE',  ( 120.8750000000000000, 7.950000000000000178, 1.460391307983218535E-15 ) ) ;
#100914=CARTESIAN_POINT ( 'NONE',  ( 31.70376352523145158, 6.109999999999999432, 1.122388791418549108E-15 ) ) ;
#100932=CARTESIAN_POINT ( 'NONE',  ( 121.0420968585647756, 5.291415217122923842, -3.054999999999996163 ) ) ;
#100936=CARTESIAN_POINT ( 'NONE',  ( 78.72916666666665719, 7.950000000000001954, -2.130196079827421762 ) ) ;
#100941=CARTESIAN_POINT ( 'NONE',  ( 48.93336038379622721, 2.130196079827431532, -7.949999999999997513 ) ) ;
#100947=CARTESIAN_POINT ( 'NONE',  ( 48.97916666666665009, -7.950000000000001066, 2.130196079827424427 ) ) ;
#100956=CARTESIAN_POINT ( 'NONE',  ( 36.75043019189811133, 3.055000000000002824, -5.291415217122919401 ) ) ;
#100980=CARTESIAN_POINT ( 'NONE',  ( 60.14126352523143737, 4.472830434245836706, 4.472830434245840259 ) ) ;
#100998=DIRECTION ( 'NONE',  ( -1.000000000000000000, -0.000000000000000000, -0.000000000000000000 ) ) ;
#101007=CARTESIAN_POINT ( 'NONE',  ( 78.66209685856479439, -5.291415217122919401, 3.054999999999997939 ) ) ;
#101050=VECTOR ( 'NONE', #59161, 1000.000000000000000 ) ;
#101080=CARTESIAN_POINT ( 'NONE',  ( 111.5416666666666572, -3.975000000000002753, 6.884901960086286188 ) ) ;
#101085=CARTESIAN_POINT ( 'NONE',  ( 56.64126352523144448, 4.472830434245837594, 4.472830434245841147 ) ) ;
#101109=CARTESIAN_POINT ( 'NONE',  ( 77.07919371712957002, 3.975000000000002753, -6.884901960086283523 ) ) ;
#101114=CARTESIAN_POINT ( 'NONE',  ( 73.04166666666667140, -3.975000000000002753, 6.884901960086286188 ) ) ;
#101124=CARTESIAN_POINT ( 'NONE',  ( 69.56293019189810423, 1.637169565754157174, 6.110000000000002984 ) ) ;
#101144=CARTESIAN_POINT ( 'NONE',  ( 57.89626352523144703, 4.472830434245840259, -4.472830434245839371 ) ) ;
#101161=CARTESIAN_POINT ( 'NONE',  ( 112.5166937171295700, 7.950000000000000178, -2.130196079827421318 ) ) ;
#101169=CARTESIAN_POINT ( 'NONE',  ( 37.12086038379622011, -6.884901960086286188, 3.974999999999997424 ) ) ;
#101176=EDGE_CURVE ( 'NONE', #20563, #133316, #86635, .T. ) ;
#101178=CARTESIAN_POINT ( 'NONE',  ( 100.3912635252314516, -4.472830434245838482, -4.472830434245838482 ) ) ;
#101193=CARTESIAN_POINT ( 'NONE',  ( 68.95833333333332860, 3.974999999999997424, 6.884901960086288852 ) ) ;
#101204=CARTESIAN_POINT ( 'NONE',  ( 53.66709685856477563, -3.055000000000000160, -5.291415217122921177 ) ) ;
#101210=CARTESIAN_POINT ( 'NONE',  ( 88.37543019189811844, -5.291415217122920289, -3.055000000000001492 ) ) ;
#101218=( BOUNDED_CURVE ( )  B_SPLINE_CURVE ( 2, ( #125784, #26459, #5387, #113446, #27875, #125047, #50359, #6084, #72146, #138075, #70710, #116318, #15533 ),
 .UNSPECIFIED., .F., .F. ) 
 B_SPLINE_CURVE_WITH_KNOTS ( ( 3, 2, 2, 2, 2, 2, 3 ),
 ( 0.1666666666666666574, 0.1694444444444444531, 0.1722222222222222210, 0.1749999999999999889, 0.1777777777777777846, 0.1805555555555555525, 0.1833333333333333204 ),
 .UNSPECIFIED. ) 
 CURVE ( )  GEOMETRIC_REPRESENTATION_ITEM ( )  RATIONAL_B_SPLINE_CURVE ( ( 1.000000000000000000, 0.9659258262890683122, 1.000000000000000000, 0.9659258262890683122, 1.000000000000000000, 0.9659258262890683122, 1.000000000000000000, 0.9659258262890683122, 1.000000000000000000, 0.9659258262890683122, 1.000000000000000000, 0.9659258262890683122, 1.000000000000000000 ) ) 
 REPRESENTATION_ITEM ( '' )  );
#101246=AXIS2_PLACEMENT_3D ( 'NONE', #32744, #44341, #43595 ) ;
#101252=CARTESIAN_POINT ( 'NONE',  ( 57.72916666666665009, 7.950000000000001954, -2.130196079827421762 ) ) ;
#101284=CARTESIAN_POINT ( 'NONE',  ( 98.80836038379622721, 7.949999999999997513, 2.130196079827431088 ) ) ;
#101300=CARTESIAN_POINT ( 'NONE',  ( 92.31293019189811844, -1.637169565754159617, -6.110000000000001208 ) ) ;
#101325=CARTESIAN_POINT ( 'NONE',  ( 79.77126352523144703, 4.472830434245839371, 4.472830434245842035 ) ) ;
#101336=CARTESIAN_POINT ( 'NONE',  ( 87.55793019189812298, 6.110000000000000320, -1.637169565754156064 ) ) ;
#101363=CARTESIAN_POINT ( 'NONE',  ( 56.80836038379622011, 7.949999999999996625, 2.130196079827431088 ) ) ;
#101372=CARTESIAN_POINT ( 'NONE',  ( 0.000000000000000000, 0.000000000000000000, 0.000000000000000000 ) ) ;
#101383=CARTESIAN_POINT ( 'NONE',  ( 94.77083333333331439, -7.949999999999998401, -2.130196079827426203 ) ) ;
#101387=CARTESIAN_POINT ( 'NONE',  ( 117.3962635252314470, 4.472830434245840259, -4.472830434245838482 ) ) ;
#101414=CARTESIAN_POINT ( 'NONE',  ( 83.47459685856478018, 1.637169565754164280, -6.109999999999997655 ) ) ;
#101463=CARTESIAN_POINT ( 'NONE',  ( 87.77083333333331439, -7.949999999999999289, -2.130196079827426203 ) ) ;
#101492=CARTESIAN_POINT ( 'NONE',  ( 122.7920968585647756, -5.291415217122921177, 3.054999999999999272 ) ) ;
#101500=CARTESIAN_POINT ( 'NONE',  ( 117.4537635252314516, -6.109999999999998543, -3.741295971395162543E-16 ) ) ;
#101515=CARTESIAN_POINT ( 'NONE',  ( 28.64126352523144092, 4.472830434245836706, 4.472830434245840259 ) ) ;
#101541=ORIENTED_EDGE ( 'NONE', *, *, #93484, .F. ) ;
#101544=CARTESIAN_POINT ( 'NONE',  ( 45.84959685856478018, 6.109999999999996767, 1.637169565754163836 ) ) ;
#101578=CARTESIAN_POINT ( 'NONE',  ( 113.2245968585647944, -1.637169565754161171, 6.109999999999998543 ) ) ;
#101601=ORIENTED_EDGE ( 'NONE', *, *, #70004, .F. ) ;
#101633=CARTESIAN_POINT ( 'NONE',  ( 123.2083333333333428, -3.974999999999999201, -6.884901960086287964 ) ) ;
#101636=ORIENTED_EDGE ( 'NONE', *, *, #69297, .T. ) ;
#101645=CARTESIAN_POINT ( 'NONE',  ( 118.2712635252314470, 4.472830434245839371, 4.472830434245842035 ) ) ;
#101649=CARTESIAN_POINT ( 'NONE',  ( 105.9541937171295700, 6.884901960086283523, 3.975000000000002753 ) ) ;
#101656=CARTESIAN_POINT ( 'NONE',  ( 43.82919371712955581, -3.975000000000001865, 6.884901960086284411 ) ) ;
#101662=CARTESIAN_POINT ( 'NONE',  ( 45.91666666666666430, -6.884901960086287076, -3.975000000000000977 ) ) ;
#101668=CARTESIAN_POINT ( 'NONE',  ( 40.54209685856477563, 5.291415217122923842, -3.054999999999996163 ) ) ;
#101681=AXIS2_PLACEMENT_3D ( 'NONE', #67335, #111528, #102815 ) ;
#101693=CARTESIAN_POINT ( 'NONE',  ( 87.72502705046289861, 5.819803920172573974, -5.819803920172573086 ) ) ;
#101694=CARTESIAN_POINT ( 'NONE',  ( 62.03709685856478728, -3.054999999999998828, -5.291415217122919401 ) ) ;
#101726=AXIS2_PLACEMENT_3D ( 'NONE', #17760, #53072, #115629 ) ;
#101730=CARTESIAN_POINT ( 'NONE',  ( 76.91209685856479439, 5.291415217122921177, -3.054999999999994831 ) ) ;
#101741=CYLINDRICAL_SURFACE ( 'NONE', #34331, 7.950000000000000178 ) ;
#101745=ORIENTED_EDGE ( 'NONE', *, *, #73493, .F. ) ;
#101753=CARTESIAN_POINT ( 'NONE',  ( 30.91709685856476497, 3.054999999999998828, 5.291415217122922066 ) ) ;
#101807=CARTESIAN_POINT ( 'NONE',  ( 59.84959685856477307, 6.109999999999997655, 1.637169565754163836 ) ) ;
#101833=CARTESIAN_POINT ( 'NONE',  ( 74.30836038379624142, 7.949999999999997513, 2.130196079827431088 ) ) ;
#101838=CARTESIAN_POINT ( 'NONE',  ( 77.85416666666667140, -2.130196079827425315, -7.950000000000001066 ) ) ;
#101847=CARTESIAN_POINT ( 'NONE',  ( 68.83376352523143282, 6.110000000000001208, 1.122388791418549305E-15 ) ) ;
#101848=DIRECTION ( 'NONE',  ( -1.000000000000000000, -0.000000000000000000, -0.000000000000000000 ) ) ;
#101856=CARTESIAN_POINT ( 'NONE',  ( 84.99999999999998579, 0.000000000000000000, -7.950000000000000178 ) ) ;
#101864=CARTESIAN_POINT ( 'NONE',  ( 56.29209685856477563, -5.291415217122921177, 3.054999999999999272 ) ) ;
#101878=CARTESIAN_POINT ( 'NONE',  ( 113.2458603837962272, 3.974999999999996980, 6.884901960086287964 ) ) ;
#101899=CARTESIAN_POINT ( 'NONE',  ( 100.6829301918981088, -1.637169565754158951, -6.109999999999998543 ) ) ;
#101927=CARTESIAN_POINT ( 'NONE',  ( 57.02126352523143993, -4.472830434245838482, -4.472830434245840259 ) ) ;
#101932=CARTESIAN_POINT ( 'NONE',  ( 90.70876352523143282, -7.482591942790329030E-16, 6.110000000000001208 ) ) ;
#101945=CARTESIAN_POINT ( 'NONE',  ( 125.6204301918981088, 3.055000000000002380, -5.291415217122917625 ) ) ;
#101976=CARTESIAN_POINT ( 'NONE',  ( 6.536636313907743911, 9.243372422612678108, -2.206661907051261640 ) ) ;
#102004=CARTESIAN_POINT ( 'NONE',  ( 102.3083603837962130, 7.949999999999997513, 2.130196079827431088 ) ) ;
#102021=CARTESIAN_POINT ( 'NONE',  ( 95.52126352523141861, -4.472830434245839371, -4.472830434245840259 ) ) ;
#102045=CARTESIAN_POINT ( 'NONE',  ( 87.35459685856476142, -1.637169565754161615, 6.110000000000000320 ) ) ;
#102052=ORIENTED_EDGE ( 'NONE', *, *, #70240, .F. ) ;
#102056=CARTESIAN_POINT ( 'NONE',  ( 78.51626352523145158, -4.472830434245839371, 4.472830434245839371 ) ) ;
#102116=CARTESIAN_POINT ( 'NONE',  ( 95.06250000000000000, -5.819803920172573086, -5.819803920172573974 ) ) ;
#102120=CARTESIAN_POINT ( 'NONE',  ( 121.1879301918980900, 6.110000000000002984, -1.637169565754156730 ) ) ;
#102139=VERTEX_POINT ( 'NONE', #24939 ) ;
#102157=CARTESIAN_POINT ( 'NONE',  ( 98.37086038379622721, 6.884901960086289741, -3.974999999999993427 ) ) ;
#102205=CARTESIAN_POINT ( 'NONE',  ( 95.50000000000000000, 0.000000000000000000, -7.950000000000000178 ) ) ;
#102217=CARTESIAN_POINT ( 'NONE',  ( 12.99859279590333472, 8.843460517209971172, -3.474509921214832708 ) ) ;
#102223=CARTESIAN_POINT ( 'NONE',  ( 126.2410695880550833, 6.589327892697261824, -2.966880743088488259 ) ) ;
#102225=CARTESIAN_POINT ( 'NONE',  ( 127.2245968585647660, -1.637169565754160949, 6.109999999999997655 ) ) ;
#102237=CARTESIAN_POINT ( 'NONE',  ( 107.1879301918980900, 6.110000000000002984, -1.637169565754156730 ) ) ;
#102245=CARTESIAN_POINT ( 'NONE',  ( 102.4329301918980946, 1.637169565754156508, 6.110000000000000320 ) ) ;
#102261=CARTESIAN_POINT ( 'NONE',  ( 33.30793019189810877, -6.109999999999998543, 1.637169565754158063 ) ) ;
#102287=CARTESIAN_POINT ( 'NONE',  ( 62.78752705046289151, 0.000000000000000000, -7.949999999999998401 ) ) ;
#102298=CARTESIAN_POINT ( 'NONE',  ( 42.20376352523144448, 6.109999999999998543, 1.122388791418548911E-15 ) ) ;
#102333=CARTESIAN_POINT ( 'NONE',  ( 108.7037635252314516, 6.109999999999999432, 1.122388791418549108E-15 ) ) ;
#102366=CARTESIAN_POINT ( 'NONE',  ( 53.49999999999999289, 0.000000000000000000, -7.950000000000000178 ) ) ;
#102382=CARTESIAN_POINT ( 'NONE',  ( 122.0416666666666714, -3.975000000000002753, 6.884901960086286188 ) ) ;
#102395=CARTESIAN_POINT ( 'NONE',  ( 116.5212635252314328, -4.472830434245839371, -4.472830434245840259 ) ) ;
#102407=CARTESIAN_POINT ( 'NONE',  ( 43.24586038379622721, 3.974999999999996980, 6.884901960086287964 ) ) ;
#102412=CARTESIAN_POINT ( 'NONE',  ( 38.04166666666665719, -3.975000000000002753, 6.884901960086286188 ) ) ;
#102425=CARTESIAN_POINT ( 'NONE',  ( 33.68793019189809712, 6.110000000000002984, -1.637169565754156730 ) ) ;
#102436=CARTESIAN_POINT ( 'NONE',  ( 38.28752705046288440, 0.000000000000000000, -7.949999999999998401 ) ) ;
#102442=CARTESIAN_POINT ( 'NONE',  ( 55.03709685856478018, -3.054999999999998828, -5.291415217122919401 ) ) ;
#102449=FACE_OUTER_BOUND ( 'NONE', #76043, .T. ) ;
#102471=CARTESIAN_POINT ( 'NONE',  ( 62.91209685856477307, 5.291415217122921177, -3.054999999999994831 ) ) ;
#102487=VECTOR ( 'NONE', #7153, 1000.000000000000227 ) ;
#102497=DIRECTION ( 'NONE',  ( -1.000000000000000000, -0.000000000000000000, -0.000000000000000000 ) ) ;
#102536=CARTESIAN_POINT ( 'NONE',  ( 65.12086038379621300, -6.884901960086286188, 3.974999999999997424 ) ) ;
#102545=CARTESIAN_POINT ( 'NONE',  ( 57.66209685856478728, -5.291415217122919401, 3.054999999999998384 ) ) ;
#102571=CARTESIAN_POINT ( 'NONE',  ( 74.74586038379622721, 3.974999999999996980, 6.884901960086287964 ) ) ;
#102575=CARTESIAN_POINT ( 'NONE',  ( 71.29166666666667140, 3.975000000000003642, -6.884901960086285300 ) ) ;
#102585=CARTESIAN_POINT ( 'NONE',  ( 65.33376352523143282, 6.110000000000001208, 1.122388791418549305E-15 ) ) ;
#102594=CARTESIAN_POINT ( 'NONE',  ( 85.14583333333334281, 2.130196079827394229, -7.950000000000021494 ) ) ;
#102597=FACE_OUTER_BOUND ( 'NONE', #77482, .T. ) ;
#102607=CARTESIAN_POINT ( 'NONE',  ( 0.000000000000000000, 7.776507174585697093E-16, -6.350000000000004086 ) ) ;
#102608=CARTESIAN_POINT ( 'NONE',  ( 53.49999999999999289, 0.000000000000000000, -7.950000000000000178 ) ) ;
#102634=CARTESIAN_POINT ( 'NONE',  ( 105.0579301918981230, 6.110000000000000320, -1.637169565754156064 ) ) ;
#102661=CARTESIAN_POINT ( 'NONE',  ( 53.52126352523143993, -4.472830434245838482, -4.472830434245840259 ) ) ;
#102691=LINE ( 'NONE', #125133, #139730 ) ;
#102697=ORIENTED_EDGE ( 'NONE', *, *, #139990, .T. ) ;
#102700=CARTESIAN_POINT ( 'NONE',  ( 95.16252705046289861, 7.949999999999998401, 1.460391307983218338E-15 ) ) ;
#102703=CARTESIAN_POINT ( 'NONE',  ( 5.949829201373897369, 9.500078657251188829, -0.2878427395703713754 ) ) ;
#102725=VERTEX_POINT ( 'NONE', #24778 ) ;
#102727=CARTESIAN_POINT ( 'NONE',  ( 105.8083603837962414, 7.949999999999997513, 2.130196079827431088 ) ) ;
#102745=CARTESIAN_POINT ( 'NONE',  ( 92.16709685856477563, -3.055000000000000160, -5.291415217122921177 ) ) ;
#102762=CARTESIAN_POINT ( 'NONE',  ( 102.7458603837962272, 3.974999999999996980, 6.884901960086287964 ) ) ;
#102770=CARTESIAN_POINT ( 'NONE',  ( 81.66709685856477563, -3.055000000000000160, -5.291415217122921177 ) ) ;
#102780=CARTESIAN_POINT ( 'NONE',  ( 102.7916666666666714, 3.975000000000003642, -6.884901960086285300 ) ) ;
#102785=CARTESIAN_POINT ( 'NONE',  ( 80.70376352523145158, 6.109999999999998543, 1.122388791418548911E-15 ) ) ;
#102815=DIRECTION ( 'NONE',  ( 0.000000000000000000, 0.000000000000000000, 1.000000000000000000 ) ) ;
#102821=DIRECTION ( 'NONE',  ( 0.000000000000000000, 0.000000000000000000, 1.000000000000000000 ) ) ;
#102832=EDGE_CURVE ( 'NONE', #92449, #55968, #59365, .T. ) ;
#102835=CARTESIAN_POINT ( 'NONE',  ( 118.2712635252314470, 4.472830434245838482, 4.472830434245842035 ) ) ;
#102913=CARTESIAN_POINT ( 'NONE',  ( 90.83333333333332860, -6.884901960086287964, 3.974999999999998312 ) ) ;
#102919=CARTESIAN_POINT ( 'NONE',  ( 14.64180977014269303, 9.473308030796305346, -0.7257954063774550990 ) ) ;
#102925=CARTESIAN_POINT ( 'NONE',  ( 125.6430803969771404, -1.520810258758055200, -7.661534144229997345 ) ) ;
#102936=ORIENTED_EDGE ( 'NONE', *, *, #55548, .T. ) ;
#102938=CARTESIAN_POINT ( 'NONE',  ( 112.5837635252314470, -6.110000000000001208, -3.741295971395164515E-16 ) ) ;
#102945=FACE_OUTER_BOUND ( 'NONE', #61449, .T. ) ;
#102948=CARTESIAN_POINT ( 'NONE',  ( 106.9537635252314516, -6.109999999999998543, -3.741295971395162543E-16 ) ) ;
#102991=CARTESIAN_POINT ( 'NONE',  ( 37.09959685856476597, -6.109999999999997655, -1.637169565754160283 ) ) ;
#103025=CARTESIAN_POINT ( 'NONE',  ( 99.51626352523145158, -4.472830434245839371, 4.472830434245839371 ) ) ;
#103058=CARTESIAN_POINT ( 'NONE',  ( 52.18749999999999289, -5.819803920172573974, 5.819803920172573086 ) ) ;
#103072=CARTESIAN_POINT ( 'NONE',  ( 27.93336038379622011, 2.130196079827431532, -7.949999999999996625 ) ) ;
#103077=CARTESIAN_POINT ( 'NONE',  ( 120.0000000000000000, 0.000000000000000000, -7.950000000000000178 ) ) ;
#103089=CARTESIAN_POINT ( 'NONE',  ( 115.6462635252314328, -4.472830434245840259, 4.472830434245839371 ) ) ;
#103099=CARTESIAN_POINT ( 'NONE',  ( 49.95419371712955581, 6.884901960086283523, 3.975000000000002753 ) ) ;
#103102=ORIENTED_EDGE ( 'NONE', *, *, #42566, .T. ) ;
#103103=CARTESIAN_POINT ( 'NONE',  ( 34.24999999999998579, -9.735942053221458872E-16, 7.950000000000000178 ) ) ;
#103109=FACE_OUTER_BOUND ( 'NONE', #71576, .T. ) ;
#103112=CARTESIAN_POINT ( 'NONE',  ( 26.83376352523143993, 6.110000000000001208, 1.122388791418549305E-15 ) ) ;
#103128=CARTESIAN_POINT ( 'NONE',  ( 47.16209685856477307, -5.291415217122919401, 3.054999999999997939 ) ) ;
#103130=CARTESIAN_POINT ( 'NONE',  ( 123.7916666666666714, 3.975000000000003642, -6.884901960086285300 ) ) ;
#103155=CARTESIAN_POINT ( 'NONE',  ( 69.76626352523143737, 4.472830434245838482, -4.472830434245837594 ) ) ;
#103178=CARTESIAN_POINT ( 'NONE',  ( 29.29166666666666075, 3.975000000000003642, -6.884901960086285300 ) ) ;
#103181=CARTESIAN_POINT ( 'NONE',  ( 42.95419371712954870, 6.884901960086283523, 3.975000000000002753 ) ) ;
#103186=CARTESIAN_POINT ( 'NONE',  ( 119.3708603837962272, 6.884901960086289741, -3.974999999999993427 ) ) ;
#103205=FACE_OUTER_BOUND ( 'NONE', #70906, .T. ) ;
#103225=CARTESIAN_POINT ( 'NONE',  ( 50.66209685856478018, -5.291415217122919401, 3.054999999999998384 ) ) ;
#103248=CARTESIAN_POINT ( 'NONE',  ( 72.55836038379624142, -7.949999999999997513, -2.130196079827425759 ) ) ;
#103253=CARTESIAN_POINT ( 'NONE',  ( 61.52083333333332149, 7.949999999999999289, 2.130196079827431532 ) ) ;
#103261=CARTESIAN_POINT ( 'NONE',  ( 54.54209685856477563, 5.291415217122923842, -3.054999999999996163 ) ) ;
#103306=CARTESIAN_POINT ( 'NONE',  ( 91.05793019189812298, 6.110000000000000320, -1.637169565754156064 ) ) ;
#103330=CARTESIAN_POINT ( 'NONE',  ( 42.72959685856476142, -6.110000000000000320, -1.637169565754161393 ) ) ;
#103349=CARTESIAN_POINT ( 'NONE',  ( 127.0787635252314516, -7.482591942790327058E-16, 6.109999999999999432 ) ) ;
#103379=CARTESIAN_POINT ( 'NONE',  ( 8.372076165025809757, 8.651961987691654699, 3.925355617310125833 ) ) ;
#103406=CARTESIAN_POINT ( 'NONE',  ( 103.6208603837962272, -6.884901960086286188, 3.974999999999997424 ) ) ;
#103421=CARTESIAN_POINT ( 'NONE',  ( 97.41709685856478984, 3.054999999999998828, 5.291415217122922066 ) ) ;
#103448=CARTESIAN_POINT ( 'NONE',  ( 81.81293019189810423, -1.637169565754159617, -6.110000000000001208 ) ) ;
#103457=CARTESIAN_POINT ( 'NONE',  ( 102.9375000000000000, 5.819803920172574863, -5.819803920172573086 ) ) ;
#103459=CARTESIAN_POINT ( 'NONE',  ( 74.14126352523146579, 4.472830434245836706, 4.472830434245840259 ) ) ;
#103466=CARTESIAN_POINT ( 'NONE',  ( 64.14583333333332860, 2.130196079827431976, -7.949999999999998401 ) ) ;
#103483=CARTESIAN_POINT ( 'NONE',  ( 69.64169371712954160, -2.130196079827424871, -7.949999999999998401 ) ) ;
#103501=CARTESIAN_POINT ( 'NONE',  ( 71.45876352523143282, 0.000000000000000000, -6.110000000000001208 ) ) ;
#103506=CARTESIAN_POINT ( 'NONE',  ( 117.6879301918981042, 6.110000000000002984, -1.637169565754156730 ) ) ;
#103575=CARTESIAN_POINT ( 'NONE',  ( 128.7041937171295842, -6.884901960086285300, -3.975000000000000089 ) ) ;
#103592=CARTESIAN_POINT ( 'NONE',  ( 88.35416666666665719, -2.130196079827425315, -7.950000000000001066 ) ) ;
#103612=ORIENTED_EDGE ( 'NONE', *, *, #122637, .T. ) ;
#103614=CARTESIAN_POINT ( 'NONE',  ( 110.1045968585647756, 1.637169565754164946, -6.109999999999999432 ) ) ;
#103624=CARTESIAN_POINT ( 'NONE',  ( 101.1204301918981230, 3.055000000000001936, -5.291415217122916737 ) ) ;
#103665=CARTESIAN_POINT ( 'NONE',  ( 35.49543019189811588, 5.291415217122916737, 3.055000000000001936 ) ) ;
#103670=EDGE_CURVE ( 'NONE', #120796, #9583, #63183, .T. ) ;
#103700=CARTESIAN_POINT ( 'NONE',  ( 97.32876352523145158, 0.000000000000000000, -6.109999999999999432 ) ) ;
#103748=CARTESIAN_POINT ( 'NONE',  ( 28.22502705046288440, 5.819803920172573974, -5.819803920172573086 ) ) ;
#103753=CARTESIAN_POINT ( 'NONE',  ( 121.1666666666666714, 6.884901960086285300, 3.975000000000003642 ) ) ;
#103761=( BOUNDED_CURVE ( )  B_SPLINE_CURVE ( 2, ( #138616, #39308, #58966, #71953, #83530, #116845, #127742, #49494, #113997, #26282, #82121, #116124, #14685 ),
 .UNSPECIFIED., .F., .T. ) 
 B_SPLINE_CURVE_WITH_KNOTS ( ( 3, 2, 2, 2, 2, 2, 3 ),
 ( 0.5999999999999999778, 0.6027777777777777457, 0.6055555555555555136, 0.6083333333333332815, 0.6111111111111111605, 0.6138888888888889284, 0.6166666666666666963 ),
 .UNSPECIFIED. ) 
 CURVE ( )  GEOMETRIC_REPRESENTATION_ITEM ( )  RATIONAL_B_SPLINE_CURVE ( ( 1.000000000000000000, 0.9659258262890683122, 1.000000000000000000, 0.9659258262890683122, 1.000000000000000000, 0.9659258262890683122, 1.000000000000000000, 0.9659258262890683122, 1.000000000000000000, 0.9659258262890683122, 1.000000000000000000, 0.9659258262890683122, 1.000000000000000000 ) ) 
 REPRESENTATION_ITEM ( '' )  );
#103766=CARTESIAN_POINT ( 'NONE',  ( 108.7920968585647756, -5.291415217122921177, 3.054999999999999272 ) ) ;
#103771=CARTESIAN_POINT ( 'NONE',  ( 82.62086038379624142, -6.884901960086286188, 3.974999999999997424 ) ) ;
#103775=CARTESIAN_POINT ( 'NONE',  ( 34.49586038379622011, -3.974999999999998312, -6.884901960086286188 ) ) ;
#103781=CARTESIAN_POINT ( 'NONE',  ( 33.81249999999999289, 5.819803920172571310, 5.819803920172575751 ) ) ;
#103792=CARTESIAN_POINT ( 'NONE',  ( 28.29209685856476497, -5.291415217122921177, 3.054999999999999272 ) ) ;
#103802=CARTESIAN_POINT ( 'NONE',  ( 0.000000000000000000, 0.000000000000000000, 0.000000000000000000 ) ) ;
#103806=CARTESIAN_POINT ( 'NONE',  ( 51.53709685856478018, -3.054999999999998828, -5.291415217122919401 ) ) ;
#103837=CARTESIAN_POINT ( 'NONE',  ( 66.41209685856478018, 5.291415217122921177, -3.054999999999994831 ) ) ;
#103850=CARTESIAN_POINT ( 'NONE',  ( 0.000000000000000000, 9.735942053221458872E-16, -7.950000000000000178 ) ) ;
#103865=CARTESIAN_POINT ( 'NONE',  ( 29.72916666666665009, 7.950000000000001954, -2.130196079827421762 ) ) ;
#103886=CARTESIAN_POINT ( 'NONE',  ( 107.7500000000000000, -9.735942053221458872E-16, 7.950000000000000178 ) ) ;
#103910=CARTESIAN_POINT ( 'NONE',  ( 43.53752705046289151, -9.735942053221456900E-16, 7.949999999999998401 ) ) ;
#103916=CARTESIAN_POINT ( 'NONE',  ( 45.26626352523144448, 4.472830434245839371, -4.472830434245839371 ) ) ;
#103927=FACE_OUTER_BOUND ( 'NONE', #132771, .T. ) ;
#103928=LINE ( 'NONE', #4577, #97520 ) ;
#103942=CARTESIAN_POINT ( 'NONE',  ( 65.26669371712957002, -7.949999999999999289, 2.130196079827424427 ) ) ;
#103943=DIRECTION ( 'NONE',  ( -1.000000000000000000, -0.000000000000000000, -0.000000000000000000 ) ) ;
#103946=CARTESIAN_POINT ( 'NONE',  ( 62.68749999999999289, -5.819803920172573086, 5.819803920172572198 ) ) ;
#103954=CARTESIAN_POINT ( 'NONE',  ( 33.08333333333332860, 6.884901960086290629, -3.974999999999994316 ) ) ;
#103958=CARTESIAN_POINT ( 'NONE',  ( 55.12543019189811133, 5.291415217122919401, 3.055000000000002824 ) ) ;
#103982=CARTESIAN_POINT ( 'NONE',  ( 150.3000000000000114, 0.000000000000000000, 0.000000000000000000 ) ) ;
#103991=EDGE_LOOP ( 'NONE', ( #67450, #13640, #84597, #120125 ) ) ;
#104005=CARTESIAN_POINT ( 'NONE',  ( 98.05793019189812298, 6.110000000000000320, -1.637169565754156064 ) ) ;
#104035=CARTESIAN_POINT ( 'NONE',  ( 40.97959685856476852, 6.109999999999999432, 1.637169565754164280 ) ) ;
#104074=CARTESIAN_POINT ( 'NONE',  ( 96.81250000000000000, 5.819803920172571310, 5.819803920172576639 ) ) ;
#104087=CARTESIAN_POINT ( 'NONE',  ( 72.97459685856478018, 1.637169565754164280, -6.109999999999997655 ) ) ;
#104095=CARTESIAN_POINT ( 'NONE',  ( 83.24999999999998579, -9.735942053221458872E-16, 7.950000000000000178 ) ) ;
#104109=CARTESIAN_POINT ( 'NONE',  ( 93.70419371712957002, -6.884901960086285300, -3.975000000000000089 ) ) ;
#104122=CARTESIAN_POINT ( 'NONE',  ( 87.06293019189807580, 1.637169565754157174, 6.110000000000002984 ) ) ;
#104124=VECTOR ( 'NONE', #55354, 1000.000000000000000 ) ;
#104146=CARTESIAN_POINT ( 'NONE',  ( 80.20876352523143282, -7.482591942790329030E-16, 6.110000000000001208 ) ) ;
#104159=CARTESIAN_POINT ( 'NONE',  ( 75.89126352523143737, -4.472830434245839371, -4.472830434245839371 ) ) ;
#104205=CARTESIAN_POINT ( 'NONE',  ( 74.22959685856477563, -6.110000000000000320, -1.637169565754161393 ) ) ;
#104212=CARTESIAN_POINT ( 'NONE',  ( 106.4587635252314328, 0.000000000000000000, -6.110000000000001208 ) ) ;
#104248=CARTESIAN_POINT ( 'NONE',  ( 12.52748590975845566, -8.712603770609980813, -3.790722776764650526 ) ) ;
#104283=CARTESIAN_POINT ( 'NONE',  ( 126.6625270504629128, 7.949999999999998401, 1.460391307983218338E-15 ) ) ;
#104299=CARTESIAN_POINT ( 'NONE',  ( 92.87500000000000000, 7.950000000000000178, 1.460391307983218535E-15 ) ) ;
#104311=CARTESIAN_POINT ( 'NONE',  ( 126.0567959807173679, 4.951256667972520731, -5.496178947977369944 ) ) ;
#104325=CARTESIAN_POINT ( 'NONE',  ( 115.5004301918981042, -3.055000000000002380, 5.291415217122920289 ) ) ;
#104337=CARTESIAN_POINT ( 'NONE',  ( 108.4120968585647944, 5.291415217122921177, -3.054999999999994831 ) ) ;
#104366=VECTOR ( 'NONE', #133902, 1000.000000000000000 ) ;
#104395=ORIENTED_EDGE ( 'NONE', *, *, #18443, .T. ) ;
#104396=CARTESIAN_POINT ( 'NONE',  ( 34.62043019189811588, 3.055000000000001936, -5.291415217122916737 ) ) ;
#104432=CARTESIAN_POINT ( 'NONE',  ( 103.1620968585647802, -5.291415217122919401, 3.054999999999998384 ) ) ;
#104479=CARTESIAN_POINT ( 'NONE',  ( 28.95419371712955225, 6.884901960086283523, 3.975000000000002753 ) ) ;
#104481=ORIENTED_EDGE ( 'NONE', *, *, #74417, .F. ) ;
#104485=CARTESIAN_POINT ( 'NONE',  ( 120.1458333333333286, 2.130196079827431976, -7.949999999999999289 ) ) ;
#104499=CARTESIAN_POINT ( 'NONE',  ( 116.9587635252314470, 0.000000000000000000, -6.110000000000001208 ) ) ;
#104511=CARTESIAN_POINT ( 'NONE',  ( 34.78752705046288440, 0.000000000000000000, -7.949999999999998401 ) ) ;
#104516=CARTESIAN_POINT ( 'NONE',  ( 40.08333333333332860, 6.884901960086290629, -3.974999999999994316 ) ) ;
#104529=CARTESIAN_POINT ( 'NONE',  ( 28.14626352523143638, -4.472830434245840259, 4.472830434245839371 ) ) ;
#104540=CARTESIAN_POINT ( 'NONE',  ( 52.79209685856476852, -5.291415217122921177, 3.054999999999999272 ) ) ;
#104541=ORIENTED_EDGE ( 'NONE', *, *, #122732, .T. ) ;
#104549=CARTESIAN_POINT ( 'NONE',  ( 50.37043019189811588, -3.055000000000001492, 5.291415217122917625 ) ) ;
#104551=CARTESIAN_POINT ( 'NONE',  ( 124.3750000000000000, 7.950000000000000178, 1.460391307983218535E-15 ) ) ;
#104574=CARTESIAN_POINT ( 'NONE',  ( 48.25000000000000000, -9.735942053221458872E-16, 7.950000000000000178 ) ) ;
#104584=CARTESIAN_POINT ( 'NONE',  ( 63.34959685856478018, 6.109999999999996767, 1.637169565754163836 ) ) ;
#104598=EDGE_LOOP ( 'NONE', ( #105043, #131596, #69432, #125497 ) ) ;
#104630=CARTESIAN_POINT ( 'NONE',  ( 125.5000000000000000, -3.441786896390352624, 7.166352137582667758 ) ) ;
#104635=( BOUNDED_CURVE ( )  B_SPLINE_CURVE ( 2, ( #113121, #126846, #68948, #126164, #113844, #13791, #58086, #26835, #25394, #80530, #93531, #124725, #102287 ),
 .UNSPECIFIED., .F., .T. ) 
 B_SPLINE_CURVE_WITH_KNOTS ( ( 3, 2, 2, 2, 2, 2, 3 ),
 ( 0.6166666666666666963, 0.6194444444444444642, 0.6222222222222222321, 0.6250000000000000000, 0.6277777777777777679, 0.6305555555555555358, 0.6333333333333333037 ),
 .UNSPECIFIED. ) 
 CURVE ( )  GEOMETRIC_REPRESENTATION_ITEM ( )  RATIONAL_B_SPLINE_CURVE ( ( 1.000000000000000000, 0.9659258262890683122, 1.000000000000000000, 0.9659258262890683122, 1.000000000000000000, 0.9659258262890683122, 1.000000000000000000, 0.9659258262890683122, 1.000000000000000000, 0.9659258262890683122, 1.000000000000000000, 0.9659258262890683122, 1.000000000000000000 ) ) 
 REPRESENTATION_ITEM ( '' )  );
#104654=CARTESIAN_POINT ( 'NONE',  ( 45.12043019189810877, 3.055000000000002380, -5.291415217122917625 ) ) ;
#104681=CARTESIAN_POINT ( 'NONE',  ( 62.64169371712956291, -2.130196079827424871, -7.949999999999999289 ) ) ;
#104686=CARTESIAN_POINT ( 'NONE',  ( 61.66666666666666430, 6.884901960086285300, 3.975000000000003642 ) ) ;
#104697=CARTESIAN_POINT ( 'NONE',  ( 53.22959685856475431, -6.110000000000000320, -1.637169565754161393 ) ) ;
#104752=CARTESIAN_POINT ( 'NONE',  ( 95.43293019189810877, 1.637169565754156508, 6.110000000000000320 ) ) ;
#104779=CARTESIAN_POINT ( 'NONE',  ( 49.58376352523144703, -6.110000000000001208, -3.741295971395164515E-16 ) ) ;
#104789=FACE_OUTER_BOUND ( 'NONE', #121646, .T. ) ;
#104823=CARTESIAN_POINT ( 'NONE',  ( 95.60002705046287019, 5.819803920172570422, 5.819803920172575751 ) ) ;
#104827=CARTESIAN_POINT ( 'NONE',  ( 78.07876352523145158, -7.482591942790327058E-16, 6.109999999999999432 ) ) ;
#104833=EDGE_CURVE ( 'NONE', #74280, #75139, #25170, .T. ) ;
#104852=CARTESIAN_POINT ( 'NONE',  ( 90.35002705046287019, -5.819803920172572198, -5.819803920172572198 ) ) ;
#104854=CARTESIAN_POINT ( 'NONE',  ( 72.75000000000000000, -9.735942053221458872E-16, 7.950000000000000178 ) ) ;
#104866=TOROIDAL_SURFACE ( 'NONE', #7568, 8.000000000000001776, 1.500000000000000000 ) ;
#104868=CARTESIAN_POINT ( 'NONE',  ( 45.28752705046289151, 0.000000000000000000, -7.949999999999998401 ) ) ;
#104871=CARTESIAN_POINT ( 'NONE',  ( 85.45876352523143282, 0.000000000000000000, -6.110000000000001208 ) ) ;
#104880=CARTESIAN_POINT ( 'NONE',  ( 117.9125270504628986, -7.949999999999998401, -4.867971026610728450E-16 ) ) ;
#104887=CARTESIAN_POINT ( 'NONE',  ( 59.47916666666666430, -7.950000000000000178, 2.130196079827424427 ) ) ;
#104891=CARTESIAN_POINT ( 'NONE',  ( 72.33376352523143282, 6.110000000000001208, 1.122388791418549305E-15 ) ) ;
#104906=CARTESIAN_POINT ( 'NONE',  ( 33.76669371712954870, -7.949999999999998401, 2.130196079827423983 ) ) ;
#104930=FACE_OUTER_BOUND ( 'NONE', #135227, .T. ) ;
#104946=CARTESIAN_POINT ( 'NONE',  ( 69.70876352523144703, -7.482591942790329030E-16, 6.110000000000001208 ) ) ;
#104950=CARTESIAN_POINT ( 'NONE',  ( 106.8962635252314328, 4.472830434245840259, -4.472830434245838482 ) ) ;
#104998=CARTESIAN_POINT ( 'NONE',  ( 72.75000000000000000, -9.735942053221458872E-16, 7.950000000000000178 ) ) ;
#105013=CARTESIAN_POINT ( 'NONE',  ( 123.1625270504628986, 7.949999999999998401, 1.460391307983218338E-15 ) ) ;
#105032=( BOUNDED_CURVE ( )  B_SPLINE_CURVE ( 2, ( #61974, #125796, #38075, #138087, #6808, #15543, #93152, #116330, #105437, #70721, #27890, #82999, #38775 ),
 .UNSPECIFIED., .F., .F. ) 
 B_SPLINE_CURVE_WITH_KNOTS ( ( 3, 2, 2, 2, 2, 2, 3 ),
 ( 0.6333333333333333037, 0.6361111111111110716, 0.6388888888888888395, 0.6416666666666667185, 0.6444444444444444864, 0.6472222222222222543, 0.6500000000000000222 ),
 .UNSPECIFIED. ) 
 CURVE ( )  GEOMETRIC_REPRESENTATION_ITEM ( )  RATIONAL_B_SPLINE_CURVE ( ( 1.000000000000000000, 0.9659258262890683122, 1.000000000000000000, 0.9659258262890683122, 1.000000000000000000, 0.9659258262890683122, 1.000000000000000000, 0.9659258262890683122, 1.000000000000000000, 0.9659258262890683122, 1.000000000000000000, 0.9659258262890683122, 1.000000000000000000 ) ) 
 REPRESENTATION_ITEM ( '' )  );
#105034=CARTESIAN_POINT ( 'NONE',  ( 84.12500000000000000, -7.950000000000000178, -4.867971026610729436E-16 ) ) ;
#105043=ORIENTED_EDGE ( 'NONE', *, *, #24180, .T. ) ;
#105048=CARTESIAN_POINT ( 'NONE',  ( 126.9298449394060668, 2.838896997467642791, 5.891538070402098981 ) ) ;
#105058=EDGE_CURVE ( 'NONE', #32075, #19121, #86228, .T. ) ;
#105062=CARTESIAN_POINT ( 'NONE',  ( 110.3962635252314328, 4.472830434245840259, -4.472830434245839371 ) ) ;
#105068=CARTESIAN_POINT ( 'NONE',  ( 76.10416666666667140, 2.130196079827422206, 7.950000000000001954 ) ) ;
#105071=CARTESIAN_POINT ( 'NONE',  ( 106.5162635252314658, -4.472830434245839371, 4.472830434245839371 ) ) ;
#105096=CARTESIAN_POINT ( 'NONE',  ( 110.5995968585647802, -6.109999999999997655, -1.637169565754160283 ) ) ;
#105123=CARTESIAN_POINT ( 'NONE',  ( 41.47459685856478018, 1.637169565754164280, -6.109999999999996767 ) ) ;
#105157=CARTESIAN_POINT ( 'NONE',  ( 103.4537635252314516, -6.109999999999999432, -3.741295971395163529E-16 ) ) ;
#105206=CARTESIAN_POINT ( 'NONE',  ( 114.3124999999999858, 5.819803920172571310, 5.819803920172575751 ) ) ;
#105216=EDGE_CURVE ( 'NONE', #40381, #136489, #58546, .T. ) ;
#105219=CARTESIAN_POINT ( 'NONE',  ( 114.3337635252314470, 6.110000000000001208, 1.122388791418549305E-15 ) ) ;
#105221=EDGE_CURVE ( 'NONE', #133915, #76474, #73325, .T. ) ;
#105225=CARTESIAN_POINT ( 'NONE',  ( 83.64169371712955581, -2.130196079827424871, -7.949999999999998401 ) ) ;
#105230=CARTESIAN_POINT ( 'NONE',  ( 39.89169371712955581, 2.130196079827421762, 7.950000000000001066 ) ) ;
#105238=CARTESIAN_POINT ( 'NONE',  ( 40.66666666666665719, 6.884901960086285300, 3.975000000000003642 ) ) ;
#105248=CARTESIAN_POINT ( 'NONE',  ( 25.66709685856477563, -3.055000000000000160, -5.291415217122921177 ) ) ;
#105258=CARTESIAN_POINT ( 'NONE',  ( 51.33376352523143282, 6.110000000000001208, 1.122388791418549305E-15 ) ) ;
#105267=CARTESIAN_POINT ( 'NONE',  ( 52.55793019189811588, 6.110000000000000320, -1.637169565754156064 ) ) ;
#105276=CARTESIAN_POINT ( 'NONE',  ( 60.45419371712955581, 6.884901960086283523, 3.975000000000002753 ) ) ;
#105278=CARTESIAN_POINT ( 'NONE',  ( 44.12086038379622721, -6.884901960086286188, 3.974999999999997424 ) ) ;
#105293=CARTESIAN_POINT ( 'NONE',  ( 66.70376352523143737, 6.109999999999998543, 1.122388791418548911E-15 ) ) ;
#105316=CARTESIAN_POINT ( 'NONE',  ( 30.16666666666666075, 6.884901960086285300, 3.975000000000003642 ) ) ;
#105317=ORIENTED_EDGE ( 'NONE', *, *, #115701, .F. ) ;
#105335=CARTESIAN_POINT ( 'NONE',  ( 107.8958333333333286, -2.130196079827407996, 7.950000000000009059 ) ) ;
#105337=ORIENTED_EDGE ( 'NONE', *, *, #110521, .F. ) ;
#105363=CARTESIAN_POINT ( 'NONE',  ( 51.24543019189811588, -5.291415217122919401, -3.055000000000000604 ) ) ;
#105387=CARTESIAN_POINT ( 'NONE',  ( 66.72502705046289861, 5.819803920172573086, -5.819803920172572198 ) ) ;
#105392=CARTESIAN_POINT ( 'NONE',  ( 64.58333333333332860, 6.884901960086290629, -3.974999999999994316 ) ) ;
#105399=CARTESIAN_POINT ( 'NONE',  ( 32.49999999999998579, 0.000000000000000000, -7.950000000000000178 ) ) ;
#105402=CARTESIAN_POINT ( 'NONE',  ( 58.33376352523143993, 6.110000000000001208, 1.122388791418549305E-15 ) ) ;
#105426=CARTESIAN_POINT ( 'NONE',  ( 72.85002705046289861, -5.819803920172573086, -5.819803920172573086 ) ) ;
#105430=DIRECTION ( 'NONE',  ( -1.000000000000000000, -0.000000000000000000, -0.000000000000000000 ) ) ;
#105437=CARTESIAN_POINT ( 'NONE',  ( 61.62086038379622721, -6.884901960086286188, 3.974999999999997424 ) ) ;
#105447=CARTESIAN_POINT ( 'NONE',  ( 96.45376352523145158, -6.109999999999998543, -3.741295971395162543E-16 ) ) ;
#105473=CARTESIAN_POINT ( 'NONE',  ( 45.06293019189811133, 1.637169565754157174, 6.110000000000002984 ) ) ;
#105505=CARTESIAN_POINT ( 'NONE',  ( 65.89583333333332860, -2.130196079827427091, 7.949999999999998401 ) ) ;
#105513=CARTESIAN_POINT ( 'NONE',  ( 97.25000000000000000, -9.735942053221458872E-16, 7.950000000000000178 ) ) ;
#105515=CARTESIAN_POINT ( 'NONE',  ( 0.000000000000000000, 9.735942053221458872E-16, -7.950000000000000178 ) ) ;
#105521=CARTESIAN_POINT ( 'NONE',  ( 0.000000000000000000, 1.071565949253934124E-15, 8.000000000000001776 ) ) ;
#105527=CARTESIAN_POINT ( 'NONE',  ( 75.01626352523142316, -4.472830434245839371, 4.472830434245839371 ) ) ;
#105528=CARTESIAN_POINT ( 'NONE',  ( 81.20833333333332860, -3.974999999999999201, -6.884901960086287964 ) ) ;
#105537=ORIENTED_EDGE ( 'NONE', *, *, #28303, .T. ) ;
#105548=CARTESIAN_POINT ( 'NONE',  ( 92.10002705046289861, 5.819803920172570422, 5.819803920172574863 ) ) ;
#105549=CARTESIAN_POINT ( 'NONE',  ( 71.00000000000000000, 0.000000000000000000, -7.950000000000000178 ) ) ;
#105563=CARTESIAN_POINT ( 'NONE',  ( 88.81293019189809002, -1.637169565754159617, -6.110000000000001208 ) ) ;
#105582=CARTESIAN_POINT ( 'NONE',  ( 77.43793019189810423, -6.110000000000001208, 1.637169565754158951 ) ) ;
#105597=VERTEX_POINT ( 'NONE', #20182 ) ;
#105619=CARTESIAN_POINT ( 'NONE',  ( 0.000000000000000000, 0.000000000000000000, 0.000000000000000000 ) ) ;
#105635=CARTESIAN_POINT ( 'NONE',  ( 68.97959685856477563, 6.109999999999999432, 1.637169565754164280 ) ) ;
#105644=CARTESIAN_POINT ( 'NONE',  ( 106.6045968585647614, 1.637169565754164946, -6.109999999999999432 ) ) ;
#105653=CARTESIAN_POINT ( 'NONE',  ( 77.80836038379622721, 7.949999999999996625, 2.130196079827431088 ) ) ;
#105707=CARTESIAN_POINT ( 'NONE',  ( 121.2666937171295700, -7.949999999999999289, 2.130196079827424427 ) ) ;
#105720=ORIENTED_EDGE ( 'NONE', *, *, #42734, .T. ) ;
#105722=CARTESIAN_POINT ( 'NONE',  ( 78.43750000000000000, 5.819803920172573974, -5.819803920172572198 ) ) ;
#105746=CARTESIAN_POINT ( 'NONE',  ( 103.1045968585647756, 1.637169565754164946, -6.109999999999999432 ) ) ;
#105756=CARTESIAN_POINT ( 'NONE',  ( 91.34959685856478018, 6.109999999999996767, 1.637169565754163836 ) ) ;
#105782=CARTESIAN_POINT ( 'NONE',  ( 115.4120968585647944, 5.291415217122921177, -3.054999999999994831 ) ) ;
#105794=CARTESIAN_POINT ( 'NONE',  ( 36.87499999999999289, 7.950000000000000178, 1.460391307983218535E-15 ) ) ;
#105846=CARTESIAN_POINT ( 'NONE',  ( 106.0787635252314516, -7.482591942790327058E-16, 6.109999999999999432 ) ) ;
#105865=EDGE_LOOP ( 'NONE', ( #24675, #36729, #97988, #2116 ) ) ;
#105892=CARTESIAN_POINT ( 'NONE',  ( 113.8750000000000000, 7.950000000000000178, 1.460391307983218535E-15 ) ) ;
#105907=CARTESIAN_POINT ( 'NONE',  ( 107.1879301918980900, 6.110000000000002984, -1.637169565754156730 ) ) ;
#105919=CARTESIAN_POINT ( 'NONE',  ( 41.49586038379622721, -3.974999999999998312, -6.884901960086286188 ) ) ;
#105925=CARTESIAN_POINT ( 'NONE',  ( 126.4379301918981042, -6.110000000000001208, 1.637169565754158951 ) ) ;
#105934=CARTESIAN_POINT ( 'NONE',  ( 27.12543019189810067, 5.291415217122919401, 3.055000000000002824 ) ) ;
#105945=CARTESIAN_POINT ( 'NONE',  ( 55.85459685856475431, -1.637169565754161615, 6.110000000000000320 ) ) ;
#105948=EDGE_CURVE ( 'NONE', #134670, #69673, #92767, .T. ) ;
#105953=CARTESIAN_POINT ( 'NONE',  ( 45.55793019189811588, 6.110000000000000320, -1.637169565754156064 ) ) ;
#105976=CYLINDRICAL_SURFACE ( 'NONE', #123546, 6.350000000000004086 ) ;
#105979=CARTESIAN_POINT ( 'NONE',  ( 55.03709685856478018, -3.054999999999998828, -5.291415217122919401 ) ) ;
#106007=ORIENTED_EDGE ( 'NONE', *, *, #52818, .T. ) ;
#106037=DIRECTION ( 'NONE',  ( 0.000000000000000000, 0.000000000000000000, 1.000000000000000000 ) ) ;
#106055=CARTESIAN_POINT ( 'NONE',  ( 49.49543019189811588, 5.291415217122917625, 3.055000000000002380 ) ) ;
#106068=EDGE_CURVE ( 'NONE', #78734, #5013, #26952, .T. ) ;
#106076=CARTESIAN_POINT ( 'NONE',  ( 61.47502705046287730, -5.819803920172572198, 5.819803920172572198 ) ) ;
#106081=CARTESIAN_POINT ( 'NONE',  ( 54.08333333333332860, 6.884901960086290629, -3.974999999999994316 ) ) ;
#106089=CARTESIAN_POINT ( 'NONE',  ( 54.25043019189811133, 3.055000000000002824, -5.291415217122919401 ) ) ;
#106117=EDGE_CURVE ( 'NONE', #75310, #30975, #98661, .T. ) ;
#106146=CARTESIAN_POINT ( 'NONE',  ( 94.41209685856478018, 5.291415217122921177, -3.054999999999994831 ) ) ;
#106175=CARTESIAN_POINT ( 'NONE',  ( 48.70876352523144703, -7.482591942790329030E-16, 6.110000000000001208 ) ) ;
#106211=CYLINDRICAL_SURFACE ( 'NONE', #114230, 7.950000000000000178 ) ;
#106216=CARTESIAN_POINT ( 'NONE',  ( 96.66666666666667140, 6.884901960086285300, 3.975000000000003642 ) ) ;
#106228=CARTESIAN_POINT ( 'NONE',  ( 74.87043019189812298, -3.055000000000001936, 5.291415217122918513 ) ) ;
#106232=DIRECTION ( 'NONE',  ( 0.000000000000000000, 0.000000000000000000, 1.000000000000000000 ) ) ;
#106251=CARTESIAN_POINT ( 'NONE',  ( 98.07919371712955581, 3.975000000000002753, -6.884901960086283523 ) ) ;
#106264=CARTESIAN_POINT ( 'NONE',  ( 83.85459685856478984, -1.637169565754161615, 6.110000000000000320 ) ) ;
#106282=CARTESIAN_POINT ( 'NONE',  ( 75.83376352523144703, 6.110000000000001208, 1.122388791418549305E-15 ) ) ;
#106294=CARTESIAN_POINT ( 'NONE',  ( 34.78752705046288440, 0.000000000000000000, -7.949999999999998401 ) ) ;
#106343=CARTESIAN_POINT ( 'NONE',  ( 77.14626352523143282, -4.472830434245840259, 4.472830434245838482 ) ) ;
#106348=CARTESIAN_POINT ( 'NONE',  ( 110.6879301918981184, 6.110000000000002984, -1.637169565754156730 ) ) ;
#106405=CARTESIAN_POINT ( 'NONE',  ( 123.4541937171295700, 6.884901960086283523, 3.975000000000002753 ) ) ;
#106421=CARTESIAN_POINT ( 'NONE',  ( 87.47916666666665719, -7.950000000000001066, 2.130196079827424427 ) ) ;
#106425=CARTESIAN_POINT ( 'NONE',  ( 91.66252705046288440, 7.949999999999998401, 1.460391307983218338E-15 ) ) ;
#106452=CARTESIAN_POINT ( 'NONE',  ( 104.1254301918981184, 5.291415217122919401, 3.055000000000002824 ) ) ;
#106462=CARTESIAN_POINT ( 'NONE',  ( 93.97459685856478018, 1.637169565754164058, -6.109999999999996767 ) ) ;
#106484=ORIENTED_EDGE ( 'NONE', *, *, #16296, .T. ) ;
#106487=EDGE_CURVE ( 'NONE', #69673, #77789, #38178, .T. ) ;
#106518=CARTESIAN_POINT ( 'NONE',  ( 32.57876352523145158, -7.482591942790325086E-16, 6.109999999999998543 ) ) ;
#106555=CARTESIAN_POINT ( 'NONE',  ( 95.28709685856479439, 3.054999999999997939, 5.291415217122920289 ) ) ;
#106559=ORIENTED_EDGE ( 'NONE', *, *, #31435, .F. ) ;
#106600=CARTESIAN_POINT ( 'NONE',  ( 109.6458333333333286, 2.130196079827431976, -7.949999999999999289 ) ) ;
#106618=CARTESIAN_POINT ( 'NONE',  ( 99.02126352523144703, -4.472830434245839371, -4.472830434245840259 ) ) ;
#106628=CARTESIAN_POINT ( 'NONE',  ( 30.55836038379621655, -7.949999999999997513, -2.130196079827425759 ) ) ;
#106635=CARTESIAN_POINT ( 'NONE',  ( 24.77083333333332504, -7.949999999999999289, -2.130196079827426203 ) ) ;
#106641=DIRECTION ( 'NONE',  ( -1.000000000000000000, -0.000000000000000000, -0.000000000000000000 ) ) ;
#106650=CARTESIAN_POINT ( 'NONE',  ( 127.0787635252314516, -7.482591942790325086E-16, 6.109999999999998543 ) ) ;
#106661=VERTEX_POINT ( 'NONE', #76261 ) ;
#106662=CARTESIAN_POINT ( 'NONE',  ( 48.70876352523144703, -7.482591942790329030E-16, 6.110000000000001208 ) ) ;
#106670=CARTESIAN_POINT ( 'NONE',  ( 38.55793019189810877, 6.110000000000000320, -1.637169565754156064 ) ) ;
#106671=ORIENTED_EDGE ( 'NONE', *, *, #59774, .F. ) ;
#106695=CARTESIAN_POINT ( 'NONE',  ( 54.89126352523145158, -4.472830434245838482, -4.472830434245838482 ) ) ;
#106712=EDGE_LOOP ( 'NONE', ( #76069, #137584, #1888, #70380 ) ) ;
#106726=CARTESIAN_POINT ( 'NONE',  ( 55.35002705046288440, -5.819803920172573086, -5.819803920172573086 ) ) ;
#106785=CARTESIAN_POINT ( 'NONE',  ( 39.72459685856478018, -1.637169565754161171, 6.109999999999998543 ) ) ;
#106806=CARTESIAN_POINT ( 'NONE',  ( 103.9125270504628844, -7.949999999999998401, -4.867971026610728450E-16 ) ) ;
#106807=CARTESIAN_POINT ( 'NONE',  ( 64.39169371712955581, 2.130196079827421762, 7.950000000000001066 ) ) ;
#106812=CARTESIAN_POINT ( 'NONE',  ( 58.89583333333332149, -2.130196079827427091, 7.949999999999999289 ) ) ;
#106824=CARTESIAN_POINT ( 'NONE',  ( 45.64626352523142572, -4.472830434245840259, 4.472830434245839371 ) ) ;
#106836=CARTESIAN_POINT ( 'NONE',  ( 0.000000000000000000, 9.735942053221458872E-16, -7.950000000000000178 ) ) ;
#106852=CARTESIAN_POINT ( 'NONE',  ( 88.60002705046289861, 5.819803920172570422, 5.819803920172575751 ) ) ;
#106853=CARTESIAN_POINT ( 'NONE',  ( 76.76626352523142316, 4.472830434245839371, -4.472830434245838482 ) ) ;
#106883=CARTESIAN_POINT ( 'NONE',  ( 89.16209685856478018, -5.291415217122919401, 3.054999999999997939 ) ) ;
#106909=CARTESIAN_POINT ( 'NONE',  ( 31.64626352523143638, -4.472830434245840259, 4.472830434245838482 ) ) ;
#106961=CARTESIAN_POINT ( 'NONE',  ( 75.74543019189810877, -5.291415217122919401, -3.055000000000000604 ) ) ;
#106968=CARTESIAN_POINT ( 'NONE',  ( 65.75000000000000000, -9.735942053221458872E-16, 7.950000000000000178 ) ) ;
#106988=CARTESIAN_POINT ( 'NONE',  ( 98.37086038379622721, 6.884901960086289741, -3.974999999999993427 ) ) ;
#107005=CARTESIAN_POINT ( 'NONE',  ( 83.56293019189811844, 1.637169565754157174, 6.110000000000002984 ) ) ;
#107024=CARTESIAN_POINT ( 'NONE',  ( 75.54209685856477563, 5.291415217122923842, -3.054999999999996163 ) ) ;
#107057=CARTESIAN_POINT ( 'NONE',  ( 53.89169371712955581, 2.130196079827421762, 7.950000000000000178 ) ) ;
#107084=CARTESIAN_POINT ( 'NONE',  ( 64.60459685856477563, 1.637169565754164946, -6.109999999999999432 ) ) ;
#107089=CARTESIAN_POINT ( 'NONE',  ( 111.2712635252314470, 4.472830434245838482, 4.472830434245842035 ) ) ;
#107134=CARTESIAN_POINT ( 'NONE',  ( 26.10459685856476852, 1.637169565754164946, -6.109999999999999432 ) ) ;
#107153=CARTESIAN_POINT ( 'NONE',  ( 93.55836038379622721, -7.949999999999996625, -2.130196079827426203 ) ) ;
#107154=CARTESIAN_POINT ( 'NONE',  ( 120.1000270504628986, 5.819803920172570422, 5.819803920172574863 ) ) ;
#107176=CARTESIAN_POINT ( 'NONE',  ( 29.68336038379622366, -2.130196079827426203, 7.949999999999996625 ) ) ;
#107187=CARTESIAN_POINT ( 'NONE',  ( 40.95833333333333570, 3.974999999999997424, 6.884901960086288852 ) ) ;
#107197=CARTESIAN_POINT ( 'NONE',  ( 97.41709685856478984, 3.054999999999998828, 5.291415217122922066 ) ) ;
#107208=CARTESIAN_POINT ( 'NONE',  ( 92.95376352523145158, -6.109999999999998543, -3.741295971395162543E-16 ) ) ;
#107239=AXIS2_PLACEMENT_3D ( 'NONE', #103802, #60362, #72692 ) ;
#107254=CARTESIAN_POINT ( 'NONE',  ( 29.95376352523145158, -6.109999999999998543, -3.741295971395162543E-16 ) ) ;
#107293=CARTESIAN_POINT ( 'NONE',  ( 96.74543019189810877, -5.291415217122919401, -3.055000000000000604 ) ) ;
#107311=CARTESIAN_POINT ( 'NONE',  ( 69.78752705046289861, 0.000000000000000000, -7.949999999999998401 ) ) ;
#107332=CARTESIAN_POINT ( 'NONE',  ( 30.89583333333332860, -2.130196079827427091, 7.949999999999998401 ) ) ;
#107334=CARTESIAN_POINT ( 'NONE',  ( 48.25000000000000000, -9.735942053221458872E-16, 7.950000000000000178 ) ) ;
#107335=EDGE_CURVE ( 'NONE', #120211, #133905, #121550, .T. ) ;
#107347=CARTESIAN_POINT ( 'NONE',  ( 113.4374999999999716, 5.819803920172573974, -5.819803920172572198 ) ) ;
#107360=CARTESIAN_POINT ( 'NONE',  ( 103.2504301918981184, 3.055000000000002824, -5.291415217122919401 ) ) ;
#107374=CARTESIAN_POINT ( 'NONE',  ( 30.31249999999999645, 5.819803920172571310, 5.819803920172575751 ) ) ;
#107378=CYLINDRICAL_SURFACE ( 'NONE', #61828, 7.950000000000000178 ) ;
#107383=CARTESIAN_POINT ( 'NONE',  ( 127.2245968585647660, -1.637169565754160949, 6.109999999999997655 ) ) ;
#107395=CARTESIAN_POINT ( 'NONE',  ( 50.16709685856476852, -3.055000000000000160, -5.291415217122921177 ) ) ;
#107404=CARTESIAN_POINT ( 'NONE',  ( 40.30793019189810877, -6.109999999999998543, 1.637169565754158063 ) ) ;
#107433=CARTESIAN_POINT ( 'NONE',  ( 61.01626352523143737, -4.472830434245838482, 4.472830434245838482 ) ) ;
#107448=ORIENTED_EDGE ( 'NONE', *, *, #135821, .T. ) ;
#107451=ORIENTED_EDGE ( 'NONE', *, *, #122414, .T. ) ;
#107468=CARTESIAN_POINT ( 'NONE',  ( 117.3079301918980946, -6.109999999999999432, 1.637169565754158507 ) ) ;
#107475=CARTESIAN_POINT ( 'NONE',  ( 67.45419371712955581, 6.884901960086283523, 3.975000000000002753 ) ) ;
#107478=CARTESIAN_POINT ( 'NONE',  ( 76.05836038379622721, -7.949999999999996625, -2.130196079827426203 ) ) ;
#107488=DIRECTION ( 'NONE',  ( 0.000000000000000000, 0.000000000000000000, 1.000000000000000000 ) ) ;
#107494=EDGE_LOOP ( 'NONE', ( #130454, #123355 ) ) ;
#107510=CARTESIAN_POINT ( 'NONE',  ( 40.16209685856478018, -5.291415217122919401, 3.054999999999998384 ) ) ;
#107534=CARTESIAN_POINT ( 'NONE',  ( 103.4750270504628844, -5.819803920172573086, 5.819803920172573086 ) ) ;
#107535=CARTESIAN_POINT ( 'NONE',  ( 53.89169371712955581, 2.130196079827421762, 7.950000000000001066 ) ) ;
#107539=CARTESIAN_POINT ( 'NONE',  ( 51.16666666666666430, 6.884901960086285300, 3.975000000000003642 ) ) ;
#107547=CARTESIAN_POINT ( 'NONE',  ( 48.41709685856476852, 3.054999999999998828, 5.291415217122922066 ) ) ;
#107570=CARTESIAN_POINT ( 'NONE',  ( 66.84959685856479439, 6.109999999999996767, 1.637169565754163836 ) ) ;
#107603=CARTESIAN_POINT ( 'NONE',  ( 84.64126352523145158, 4.472830434245835818, 4.472830434245840259 ) ) ;
#107624=CARTESIAN_POINT ( 'NONE',  ( 39.22959685856476142, -6.110000000000000320, -1.637169565754161393 ) ) ;
#107625=VERTEX_POINT ( 'NONE', #59195 ) ;
#107626=CARTESIAN_POINT ( 'NONE',  ( 45.62500000000000000, -7.950000000000000178, -4.867971026610729436E-16 ) ) ;
#107662=ADVANCED_FACE ( 'NONE', ( #91096 ), #91915, .T. ) ;
#107676=CARTESIAN_POINT ( 'NONE',  ( 61.59959685856478018, -6.109999999999998543, -1.637169565754160727 ) ) ;
#107701=CARTESIAN_POINT ( 'NONE',  ( 85.10002705046289861, 5.819803920172570422, 5.819803920172574863 ) ) ;
#107715=CARTESIAN_POINT ( 'NONE',  ( 75.10459685856474721, 1.637169565754164946, -6.109999999999999432 ) ) ;
#107732=CARTESIAN_POINT ( 'NONE',  ( 73.93793019189809002, -6.110000000000001208, 1.637169565754158951 ) ) ;
#107741=ORIENTED_EDGE ( 'NONE', *, *, #16007, .F. ) ;
#107745=CARTESIAN_POINT ( 'NONE',  ( 33.18336038379622721, -2.130196079827426203, 7.949999999999996625 ) ) ;
#107782=CARTESIAN_POINT ( 'NONE',  ( 60.37543019189810423, -5.291415217122920289, -3.055000000000001492 ) ) ;
#107790=CARTESIAN_POINT ( 'NONE',  ( 98.00043019189810423, -3.055000000000002380, 5.291415217122920289 ) ) ;
#107812=EDGE_CURVE ( 'NONE', #49576, #46218, #7256, .T. ) ;
#107820=ORIENTED_EDGE ( 'NONE', *, *, #109794, .T. ) ;
#107822=ORIENTED_EDGE ( 'NONE', *, *, #142907, .F. ) ;
#107829=DIRECTION ( 'NONE',  ( -1.000000000000000000, -0.000000000000000000, -0.000000000000000000 ) ) ;
#107830=CARTESIAN_POINT ( 'NONE',  ( 32.81293019189809002, -1.637169565754159617, -6.110000000000001208 ) ) ;
#107835=EDGE_CURVE ( 'NONE', #2581, #142459, #131737, .T. ) ;
#107850=CARTESIAN_POINT ( 'NONE',  ( 124.6208603837962272, -6.884901960086286188, 3.974999999999997424 ) ) ;
#107876=CARTESIAN_POINT ( 'NONE',  ( 40.37499999999999289, 7.950000000000000178, 1.460391307983218535E-15 ) ) ;
#107886=CARTESIAN_POINT ( 'NONE',  ( 102.8129301918981042, -1.637169565754159617, -6.110000000000001208 ) ) ;
#107891=CARTESIAN_POINT ( 'NONE',  ( 84.66252705046289861, 7.949999999999998401, 1.460391307983218338E-15 ) ) ;
#107894=FACE_BOUND ( 'NONE', #44061, .T. ) ;
#107895=CARTESIAN_POINT ( 'NONE',  ( 97.18293019189810877, -1.637169565754158951, -6.109999999999998543 ) ) ;
#107923=CARTESIAN_POINT ( 'NONE',  ( 56.27083333333332860, -7.949999999999998401, -2.130196079827426203 ) ) ;
#107942=CARTESIAN_POINT ( 'NONE',  ( 30.97459685856477662, 1.637169565754164280, -6.109999999999996767 ) ) ;
#107945=CARTESIAN_POINT ( 'NONE',  ( 125.1254301918981184, 5.291415217122919401, 3.055000000000002824 ) ) ;
#107955=ORIENTED_EDGE ( 'NONE', *, *, #17735, .F. ) ;
#107979=CARTESIAN_POINT ( 'NONE',  ( 96.45376352523145158, -6.109999999999999432, -3.741295971395163529E-16 ) ) ;
#108020=CARTESIAN_POINT ( 'NONE',  ( 47.66666666666666430, 6.884901960086285300, 3.975000000000003642 ) ) ;
#108031=CARTESIAN_POINT ( 'NONE',  ( 107.4583333333333428, 3.974999999999997424, 6.884901960086288852 ) ) ;
#108044=CARTESIAN_POINT ( 'NONE',  ( 102.6670968585647756, -3.055000000000000160, -5.291415217122921177 ) ) ;
#108052=CARTESIAN_POINT ( 'NONE',  ( 28.95419371712955225, 6.884901960086283523, 3.975000000000002753 ) ) ;
#108057=CARTESIAN_POINT ( 'NONE',  ( 27.24999999999999645, -9.735942053221458872E-16, 7.950000000000000178 ) ) ;
#108065=CARTESIAN_POINT ( 'NONE',  ( 125.7662635252314658, 4.472830434245839371, -4.472830434245838482 ) ) ;
#108076=CARTESIAN_POINT ( 'NONE',  ( 44.91709685856476142, 3.054999999999998828, 5.291415217122922066 ) ) ;
#108088=CARTESIAN_POINT ( 'NONE',  ( 38.99543019189812298, 5.291415217122916737, 3.055000000000001936 ) ) ;
#108117=CARTESIAN_POINT ( 'NONE',  ( 54.59959685856476597, -6.109999999999997655, -1.637169565754160283 ) ) ;
#108125=CIRCLE ( 'NONE', #135900, 6.350000000000001421 ) ;
#108149=CARTESIAN_POINT ( 'NONE',  ( 121.5370968585647802, -3.054999999999999272, -5.291415217122919401 ) ) ;
#108156=CARTESIAN_POINT ( 'NONE',  ( 67.01669371712957002, 7.950000000000000178, -2.130196079827421318 ) ) ;
#108158=CARTESIAN_POINT ( 'NONE',  ( 76.49586038379621300, -3.974999999999998312, -6.884901960086286188 ) ) ;
#108190=CARTESIAN_POINT ( 'NONE',  ( 126.6275873549815003, -6.299348860240304937, -2.637261474849121878 ) ) ;
#108191=CARTESIAN_POINT ( 'NONE',  ( 37.97459685856477307, 1.637169565754164280, -6.109999999999997655 ) ) ;
#108214=CARTESIAN_POINT ( 'NONE',  ( 53.01669371712955581, 7.950000000000001066, -2.130196079827421318 ) ) ;
#108219=CARTESIAN_POINT ( 'NONE',  ( 52.04166666666666430, -3.975000000000002753, 6.884901960086286188 ) ) ;
#108225=CARTESIAN_POINT ( 'NONE',  ( 49.14626352523143282, -4.472830434245840259, 4.472830434245839371 ) ) ;
#108231=LINE ( 'NONE', #89382, #135258 ) ;
#108232=CARTESIAN_POINT ( 'NONE',  ( 80.57919371712955581, 3.975000000000002753, -6.884901960086283523 ) ) ;
#108241=CARTESIAN_POINT ( 'NONE',  ( 84.87543019189810423, -5.291415217122920289, -3.055000000000001492 ) ) ;
#108249=CARTESIAN_POINT ( 'NONE',  ( 64.22459685856478018, -1.637169565754160949, 6.109999999999997655 ) ) ;
#108281=CARTESIAN_POINT ( 'NONE',  ( 88.43293019189809456, 1.637169565754156508, 6.110000000000000320 ) ) ;
#108287=LINE ( 'NONE', #6825, #2776 ) ;
#108297=ORIENTED_EDGE ( 'NONE', *, *, #32853, .T. ) ;
#108308=CARTESIAN_POINT ( 'NONE',  ( 31.35459685856476497, -1.637169565754161615, 6.110000000000000320 ) ) ;
#108354=CARTESIAN_POINT ( 'NONE',  ( 65.53709685856478018, -3.054999999999999272, -5.291415217122919401 ) ) ;
#108382=CARTESIAN_POINT ( 'NONE',  ( 80.14169371712957002, -2.130196079827424871, -7.949999999999999289 ) ) ;
#108394=CARTESIAN_POINT ( 'NONE',  ( 72.91709685856477563, 3.054999999999998828, 5.291415217122922066 ) ) ;
#108417=CARTESIAN_POINT ( 'NONE',  ( 67.08376352523143282, -6.110000000000001208, -3.741295971395164515E-16 ) ) ;
#108429=EDGE_CURVE ( 'NONE', #98838, #34604, #17808, .T. ) ;
#108441=CARTESIAN_POINT ( 'NONE',  ( 128.3052689125804875, -5.499261314031185677, -3.175000000000000711 ) ) ;
#108449=CARTESIAN_POINT ( 'NONE',  ( 109.7245968585647660, -1.637169565754160949, 6.109999999999997655 ) ) ;
#108475=CARTESIAN_POINT ( 'NONE',  ( 60.95876352523143993, 0.000000000000000000, -6.110000000000001208 ) ) ;
#108483=CARTESIAN_POINT ( 'NONE',  ( 96.83376352523144703, 6.110000000000001208, 1.122388791418549305E-15 ) ) ;
#108491=CARTESIAN_POINT ( 'NONE',  ( 78.24586038379621300, 3.974999999999996980, 6.884901960086287964 ) ) ;
#108498=CARTESIAN_POINT ( 'NONE',  ( 126.3495968585647802, 6.109999999999996767, 1.637169565754163836 ) ) ;
#108529=CARTESIAN_POINT ( 'NONE',  ( 29.75043019189810423, 3.055000000000002824, -5.291415217122919401 ) ) ;
#108538=CARTESIAN_POINT ( 'NONE',  ( 41.24999999999999289, -9.735942053221458872E-16, 7.950000000000000178 ) ) ;
#108549=CARTESIAN_POINT ( 'NONE',  ( 116.8916937171295558, 2.130196079827421762, 7.950000000000001066 ) ) ;
#108557=CARTESIAN_POINT ( 'NONE',  ( 0.000000000000000000, 0.000000000000000000, 0.000000000000000000 ) ) ;
#108575=CARTESIAN_POINT ( 'NONE',  ( 93.45833333333334281, 3.974999999999997424, 6.884901960086288852 ) ) ;
#108579=CARTESIAN_POINT ( 'NONE',  ( 39.49999999999999289, 0.000000000000000000, -7.950000000000000178 ) ) ;
#108589=CARTESIAN_POINT ( 'NONE',  ( 92.89626352523143282, 4.472830434245840259, -4.472830434245839371 ) ) ;
#108602=CARTESIAN_POINT ( 'NONE',  ( 93.68293019189812298, -1.637169565754158951, -6.109999999999998543 ) ) ;
#108642=VERTEX_POINT ( 'NONE', #79979 ) ;
#108653=CARTESIAN_POINT ( 'NONE',  ( 27.47459685856478018, 1.637169565754164280, -6.109999999999996767 ) ) ;
#108688=CARTESIAN_POINT ( 'NONE',  ( 91.93293019189812298, 1.637169565754156730, 6.110000000000001208 ) ) ;
#108743=CARTESIAN_POINT ( 'NONE',  ( 102.5000000000000142, 0.000000000000000000, -7.950000000000000178 ) ) ;
#108753=CARTESIAN_POINT ( 'NONE',  ( 89.03752705046288440, -9.735942053221456900E-16, 7.949999999999998401 ) ) ;
#108761=CARTESIAN_POINT ( 'NONE',  ( 31.57919371712955581, 3.975000000000002753, -6.884901960086283523 ) ) ;
#108766=CARTESIAN_POINT ( 'NONE',  ( 28.85416666666666075, -2.130196079827425315, -7.950000000000001066 ) ) ;
#108778=CARTESIAN_POINT ( 'NONE',  ( 120.0787635252314516, -7.482591942790325086E-16, 6.109999999999998543 ) ) ;
#108786=PRESENTATION_STYLE_ASSIGNMENT (( #118980 ) ) ;
#108790=CARTESIAN_POINT ( 'NONE',  ( 46.81293019189811133, -1.637169565754159617, -6.110000000000001208 ) ) ;
#108800=CARTESIAN_POINT ( 'NONE',  ( 35.20376352523143737, 6.109999999999998543, 1.122388791418548911E-15 ) ) ;
#108833=CARTESIAN_POINT ( 'NONE',  ( 53.14126352523145158, 4.472830434245835818, 4.472830434245840259 ) ) ;
#108865=CARTESIAN_POINT ( 'NONE',  ( 123.5787635252314516, -7.482591942790327058E-16, 6.109999999999999432 ) ) ;
#108911=CARTESIAN_POINT ( 'NONE',  ( 33.74543019189811588, -5.291415217122919401, -3.055000000000000604 ) ) ;
#108928=CYLINDRICAL_SURFACE ( 'NONE', #16220, 7.950000000000000178 ) ;
#108936=CARTESIAN_POINT ( 'NONE',  ( 79.60416666666667140, 2.130196079827498146, 7.949999999999958433 ) ) ;
#108941=CARTESIAN_POINT ( 'NONE',  ( 58.55836038379621300, -7.949999999999997513, -2.130196079827425759 ) ) ;
#108946=CARTESIAN_POINT ( 'NONE',  ( 57.43750000000000711, 5.819803920172573974, -5.819803920172572198 ) ) ;
#108955=EDGE_CURVE ( 'NONE', #142079, #16751, #62310, .T. ) ;
#108957=CARTESIAN_POINT ( 'NONE',  ( 49.72959685856476852, -6.110000000000000320, -1.637169565754161393 ) ) ;
#108965=CARTESIAN_POINT ( 'NONE',  ( 80.72502705046288440, 5.819803920172573974, -5.819803920172573086 ) ) ;
#108973=CARTESIAN_POINT ( 'NONE',  ( 80.50043019189810423, -3.055000000000002380, 5.291415217122920289 ) ) ;
#108982=CARTESIAN_POINT ( 'NONE',  ( 67.28709685856478018, 3.054999999999997495, 5.291415217122919401 ) ) ;
#109011=DIRECTION ( 'NONE',  ( 1.000000000000000000, 0.000000000000000000, 0.000000000000000000 ) ) ;
#109012=ORIENTED_EDGE ( 'NONE', *, *, #133203, .F. ) ;
#109018=CARTESIAN_POINT ( 'NONE',  ( 82.45376352523145158, -6.109999999999998543, -3.741295971395162543E-16 ) ) ;
#109024=ORIENTED_EDGE ( 'NONE', *, *, #140874, .F. ) ;
#109025=CARTESIAN_POINT ( 'NONE',  ( 20.65000000000000213, 1.163414459189985485E-15, -9.500000000000000000 ) ) ;
#109045=CARTESIAN_POINT ( 'NONE',  ( 38.20876352523143282, -7.482591942790329030E-16, 6.110000000000001208 ) ) ;
#109102=CARTESIAN_POINT ( 'NONE',  ( 70.20376352523143737, 6.109999999999999432, 1.122388791418549108E-15 ) ) ;
#109114=CIRCLE ( 'NONE', #141630, 7.950000000000000178 ) ;
#109119=ORIENTED_EDGE ( 'NONE', *, *, #97777, .F. ) ;
#109135=CARTESIAN_POINT ( 'NONE',  ( 85.24586038379622721, 3.974999999999996980, 6.884901960086287964 ) ) ;
#109139=CARTESIAN_POINT ( 'NONE',  ( 82.52083333333331439, 7.949999999999999289, 2.130196079827431532 ) ) ;
#109151=CARTESIAN_POINT ( 'NONE',  ( 71.89626352523144703, 4.472830434245840259, -4.472830434245839371 ) ) ;
#109172=CARTESIAN_POINT ( 'NONE',  ( 61.10459685856476852, 1.637169565754164946, -6.109999999999999432 ) ) ;
#109195=CARTESIAN_POINT ( 'NONE',  ( 61.66666666666666430, 6.884901960086285300, 3.975000000000003642 ) ) ;
#109196=CIRCLE ( 'NONE', #23512, 6.350000000000008527 ) ;
#109203=CARTESIAN_POINT ( 'NONE',  ( 111.6204301918981088, 3.055000000000001936, -5.291415217122916737 ) ) ;
#109232=CARTESIAN_POINT ( 'NONE',  ( 66.06293019189810423, 1.637169565754157174, 6.110000000000002984 ) ) ;
#109236=CARTESIAN_POINT ( 'NONE',  ( 96.25043019189810423, 3.055000000000002824, -5.291415217122919401 ) ) ;
#109253=CARTESIAN_POINT ( 'NONE',  ( 121.9745968585647802, 1.637169565754164280, -6.109999999999996767 ) ) ;
#109265=EDGE_CURVE ( 'NONE', #139877, #73811, #41412, .T. ) ;
#109273=EDGE_CURVE ( 'NONE', #73811, #139877, #5193, .T. ) ;
#109284=CARTESIAN_POINT ( 'NONE',  ( 34.56293019189810423, 1.637169565754157174, 6.110000000000002984 ) ) ;
#109291=( BOUNDED_CURVE ( )  B_SPLINE_CURVE ( 2, ( #21648, #43401, #97771, #10732, #41981, #86191, #99166, #130421, #142018, #31108, #120196, #20907, #143413 ),
 .UNSPECIFIED., .F., .T. ) 
 B_SPLINE_CURVE_WITH_KNOTS ( ( 3, 2, 2, 2, 2, 2, 3 ),
 ( 0.09999999999999995004, 0.1027777777777777179, 0.1055555555555555136, 0.1083333333333332954, 0.1111111111111110633, 0.1138888888888888590, 0.1166666666666666408 ),
 .UNSPECIFIED. ) 
 CURVE ( )  GEOMETRIC_REPRESENTATION_ITEM ( )  RATIONAL_B_SPLINE_CURVE ( ( 1.000000000000000666, 0.9659258262890676461, 1.000000000000000000, 0.9659258262890683122, 1.000000000000000000, 0.9659258262890683122, 1.000000000000000000, 0.9659258262890683122, 1.000000000000000000, 0.9659258262890683122, 1.000000000000000000, 0.9659258262890686453, 0.9999999999999996669 ) ) 
 REPRESENTATION_ITEM ( '' )  );
#109292=ADVANCED_FACE ( 'NONE', ( #37676 ), #58751, .T. ) ;
#109305=CARTESIAN_POINT ( 'NONE',  ( 111.3500270504628986, -5.819803920172572198, -5.819803920172572198 ) ) ;
#109348=CARTESIAN_POINT ( 'NONE',  ( 91.87543019189811844, -5.291415217122920289, -3.055000000000001492 ) ) ;
#109357=CARTESIAN_POINT ( 'NONE',  ( 81.87043019189812298, -3.055000000000001492, 5.291415217122917625 ) ) ;
#109397=CARTESIAN_POINT ( 'NONE',  ( 116.3083603837962130, 7.949999999999996625, 2.130196079827431088 ) ) ;
#109408=CARTESIAN_POINT ( 'NONE',  ( 124.9795968585647756, 6.109999999999999432, 1.637169565754164280 ) ) ;
#109435=EDGE_CURVE ( 'NONE', #91210, #38530, #3801, .T. ) ;
#109439=CARTESIAN_POINT ( 'NONE',  ( 91.20376352523145158, 6.109999999999999432, 1.122388791418549108E-15 ) ) ;
#109460=DIRECTION ( 'NONE',  ( 0.000000000000000000, 0.000000000000000000, 1.000000000000000000 ) ) ;
#109478=VECTOR ( 'NONE', #140657, 1000.000000000000000 ) ;
#109495=CARTESIAN_POINT ( 'NONE',  ( 101.1874999999999858, -5.819803920172573086, 5.819803920172572198 ) ) ;
#109501=CARTESIAN_POINT ( 'NONE',  ( 89.37500000000000000, 7.950000000000000178, 1.460391307983218535E-15 ) ) ;
#109515=CARTESIAN_POINT ( 'NONE',  ( 28.07919371712955225, 3.975000000000002753, -6.884901960086283523 ) ) ;
#109520=CARTESIAN_POINT ( 'NONE',  ( 118.1254301918981184, 5.291415217122919401, 3.055000000000002824 ) ) ;
#109531=CARTESIAN_POINT ( 'NONE',  ( 127.9537635252314658, -6.109999999999998543, -3.741295971395162543E-16 ) ) ;
#109539=CARTESIAN_POINT ( 'NONE',  ( 42.29209685856477563, -5.291415217122921177, 3.054999999999999272 ) ) ;
#109545=CARTESIAN_POINT ( 'NONE',  ( 38.12043019189811588, 3.055000000000001936, -5.291415217122916737 ) ) ;
#109574=CARTESIAN_POINT ( 'NONE',  ( 44.24543019189810877, -5.291415217122918513, -3.055000000000000160 ) ) ;
#109609=CARTESIAN_POINT ( 'NONE',  ( 123.8704301918981230, -3.055000000000001936, 5.291415217122918513 ) ) ;
#109653=CARTESIAN_POINT ( 'NONE',  ( 36.66209685856478018, -5.291415217122919401, 3.054999999999998384 ) ) ;
#109679=CARTESIAN_POINT ( 'NONE',  ( 64.53752705046289861, -9.735942053221456900E-16, 7.949999999999998401 ) ) ;
#109683=CARTESIAN_POINT ( 'NONE',  ( 54.18336038379622011, -2.130196079827426203, 7.949999999999997513 ) ) ;
#109690=CARTESIAN_POINT ( 'NONE',  ( 44.45833333333332149, 3.974999999999997424, 6.884901960086288852 ) ) ;
#109695=( BOUNDED_CURVE ( )  B_SPLINE_CURVE ( 2, ( #105513, #6177, #128715, #104074, #106216, #71489, #50453, #29391, #5481, #70792, #92495, #93228, #138898 ),
 .UNSPECIFIED., .F., .F. ) 
 B_SPLINE_CURVE_WITH_KNOTS ( ( 3, 2, 2, 2, 2, 2, 3 ),
 ( 0.2833333333333333259, 0.2861111111111110938, 0.2888888888888888618, 0.2916666666666666852, 0.2944444444444444531, 0.2972222222222222210, 0.2999999999999999889 ),
 .UNSPECIFIED. ) 
 CURVE ( )  GEOMETRIC_REPRESENTATION_ITEM ( )  RATIONAL_B_SPLINE_CURVE ( ( 1.000000000000000000, 0.9659258262890683122, 1.000000000000000000, 0.9659258262890683122, 1.000000000000000000, 0.9659258262890683122, 1.000000000000000000, 0.9659258262890683122, 1.000000000000000000, 0.9659258262890683122, 1.000000000000000000, 0.9659258262890683122, 1.000000000000000000 ) ) 
 REPRESENTATION_ITEM ( '' )  );
#109697=CARTESIAN_POINT ( 'NONE',  ( 43.89626352523143282, 4.472830434245840259, -4.472830434245839371 ) ) ;
#109711=CARTESIAN_POINT ( 'NONE',  ( 81.08376352523144703, -6.110000000000001208, -3.741295971395164515E-16 ) ) ;
#109720=CARTESIAN_POINT ( 'NONE',  ( 66.55793019189812298, 6.110000000000000320, -1.637169565754156064 ) ) ;
#109739=CARTESIAN_POINT ( 'NONE',  ( 41.49586038379622721, -3.974999999999998312, -6.884901960086286188 ) ) ;
#109749=CARTESIAN_POINT ( 'NONE',  ( 85.66209685856478018, -5.291415217122919401, 3.054999999999997939 ) ) ;
#109769=CARTESIAN_POINT ( 'NONE',  ( 123.1625270504628986, 7.949999999999998401, 1.460391307983218338E-15 ) ) ;
#109775=CARTESIAN_POINT ( 'NONE',  ( 33.83376352523143282, 6.110000000000001208, 1.122388791418549305E-15 ) ) ;
#109780=CIRCLE ( 'NONE', #58940, 1.499999999999999556 ) ;
#109794=EDGE_CURVE ( 'NONE', #96695, #83079, #15439, .T. ) ;
#109813=CARTESIAN_POINT ( 'NONE',  ( 96.76669371712955581, -7.949999999999998401, 2.130196079827423983 ) ) ;
#109830=CARTESIAN_POINT ( 'NONE',  ( 63.34959685856478018, 6.109999999999997655, 1.637169565754163836 ) ) ;
#109834=CARTESIAN_POINT ( 'NONE',  ( 83.54166666666667140, -3.975000000000002753, 6.884901960086286188 ) ) ;
#109836=CARTESIAN_POINT ( 'NONE',  ( 153.6500000000000057, 0.000000000000000000, 0.000000000000000000 ) ) ;
#109854=CARTESIAN_POINT ( 'NONE',  ( 83.20419371712955581, -6.884901960086285300, -3.975000000000000089 ) ) ;
#109859=CARTESIAN_POINT ( 'NONE',  ( 84.27083333333332860, -7.949999999999999289, -2.130196079827426203 ) ) ;
#109870=CARTESIAN_POINT ( 'NONE',  ( 77.43793019189810423, -6.110000000000001208, 1.637169565754158951 ) ) ;
#109888=CARTESIAN_POINT ( 'NONE',  ( 63.14626352523143282, -4.472830434245840259, 4.472830434245839371 ) ) ;
#109918=CARTESIAN_POINT ( 'NONE',  ( 116.2870968585647802, 3.054999999999997495, 5.291415217122919401 ) ) ;
#109930=CARTESIAN_POINT ( 'NONE',  ( 57.53752705046289151, -9.735942053221456900E-16, 7.949999999999998401 ) ) ;
#109933=ADVANCED_FACE ( 'NONE', ( #103109 ), #114677, .T. ) ;
#109939=EDGE_LOOP ( 'NONE', ( #89227, #71260, #128604, #93910 ) ) ;
#109941=CARTESIAN_POINT ( 'NONE',  ( 63.87543019189810423, -5.291415217122920289, -3.055000000000001492 ) ) ;
#109947=CARTESIAN_POINT ( 'NONE',  ( 100.3337635252314328, 6.110000000000001208, 1.122388791418549305E-15 ) ) ;
#109964=CARTESIAN_POINT ( 'NONE',  ( 123.1412635252314374, 4.472830434245835818, 4.472830434245840259 ) ) ;
#109990=CARTESIAN_POINT ( 'NONE',  ( 31.06293019189809712, 1.637169565754157174, 6.110000000000002984 ) ) ;
#110009=CARTESIAN_POINT ( 'NONE',  ( 114.7041937171295558, -6.884901960086285300, -3.975000000000000089 ) ) ;
#110023=ORIENTED_EDGE ( 'NONE', *, *, #131079, .T. ) ;
#110045=CARTESIAN_POINT ( 'NONE',  ( 90.56293019189811844, 1.637169565754157174, 6.110000000000002984 ) ) ;
#110046=ORIENTED_EDGE ( 'NONE', *, *, #41029, .F. ) ;
#110049=CARTESIAN_POINT ( 'NONE',  ( 84.07919371712955581, 3.975000000000002753, -6.884901960086283523 ) ) ;
#110050=EDGE_LOOP ( 'NONE', ( #9852, #100167, #106484, #50745 ) ) ;
#110052=CARTESIAN_POINT ( 'NONE',  ( 84.78709685856478018, 3.054999999999997495, 5.291415217122919401 ) ) ;
#110086=CARTESIAN_POINT ( 'NONE',  ( 56.12499999999999289, -7.950000000000000178, -4.867971026610729436E-16 ) ) ;
#110097=ORIENTED_EDGE ( 'NONE', *, *, #129731, .T. ) ;
#110106=CARTESIAN_POINT ( 'NONE',  ( 124.6879301918981042, 6.110000000000002984, -1.637169565754156730 ) ) ;
#110121=( BOUNDED_CURVE ( )  B_SPLINE_CURVE ( 2, ( #69606, #1430, #79790, #57306, #24634, #34821, #34110, #68888, #25343, #23181, #58025, #102225, #79066, #80474, #124667, #131734, #8468, #108498, #120093, #54897, #52719, #99064, #142613, #10633, #77381, #96910, #78077, #141917, #110649, #11329, #143308, #55609, #41869, #54207, #33172, #53446, #121549, #131023, #122252, #109964, #133177, #33861, #22924, #99803, #44012, #88230, #43299, #109253, #98393, #32424, #22224, #20808, #476, #9934, #132485, #87511, #86088, #66486, #9180, #130318, #76659, #120835, #44769, #64332, #88960, #21539, #141156, #97662, #67189, #65064, #65804, #31007, #42607, #75230, #75921, #119392, #20085, #86806, #31701, #65755, #99027, #128298, #9885, #54850, #119344, #64282, #109918, #130984, #17373, #43261, #61630, #120785, #105782, #139185, #83359, #43963, #86760, #39143, #97602, #75879, #72527, #10581, #84099, #138453, #28976, #127571, #16656, #143261, #88183, #6446, #141864, #50727, #120040, #115949, #27522, #71781, #9126, #87470, #109203, #75188, #20039, #50025, #54159, #94214, #60938, #105096, #28266, #39878, #65016, #94916, #131685, #108449, #53398, #5759, #42558, #21497, #98346, #31658, #116688, #20760, #142569, #32372, #76614, #12733, #33124, #57003, #121497, #25037, #67896, #89591, #11286, #133822, #3284, #132435, #23622, #124371, #99752, #69290, #419, #133132, #45415, #113473, #1818, #102634, #111333, #34505, #112773, #14167, #78730, #112079, #58455, #90300, #122204, #2560, #22873, #80180, #67142, #100490, #44721, #47571, #46121, #135277, #134553, #79493, #68586, #1135, #12019, #78028, #56306, #24338, #33809, #122947, #35961, #101899, #55560, #101178, #66437, #77338, #57711, #22175, #35250, #46868, #13432, #123685, #91056, #110606, #88913, #116345, #48967, #25761, #114198, #104005, #38092, #91732, #70034, #81603, #93873, #82309, #137398, #126490, #27907, #26487, #105447, #71426, #135955, #48232, #59840, #138103, #36634, #104752, #127958, #17717, #27183, #125076, #15558, #4665, #106146, #94575, #59157, #83014, #114880, #115581, #17040, #136660, #61309, #70735, #61994, #49696, #72897, #6821, #6108, #93167, #138829, #16282, #38793, #60579, #14883, #50387, #92426, #103306, #5416, #127208, #39524, #3958, #83754, #72175, #80881, #37368, #28646, #117049, #125812, #119190, #106883, #65579, #118477, #75015, #85851, #108281, #131515, #64113, #21321, #76429, #42381, #63435, #29325, #95299, #32199, #19175, #52508, #20584, #120598, #73567, #31487, #51824, #8260, #140250, #109749, #7562, #53976, #8953, #141680, #117736, #51107, #107603, #18420, #96694, #96010, #40246, #87294, #139563, #40936, #19873, #74283, #97424, #84460, #128652, #62701, #30787, #109018, #130823, #140941, #85140, #129350, #75710, #30035, #41632, #130088, #53215, #86594, #119879, #64834, #9709, #98172, #142403, #43088, #238, #43789, #57541, #88738, #24178, #133657, #88002, #44539, #77845, #101007, #132970, #56849, #968, #12568, #79318, #54678, #80025, #33649, #112610, #13268, #1661, #101730, #132251, #56127, #35077, #55390, #23448, #123520, #98858, #32942, #45948, #135114, #24877, #2380, #111907, #90133, #45253, #111151, #100315, #34337, #121332, #11841, #110440, #143095, #46701, #124199, #77162, #122032, #22016, #66265, #68431, #90883, #22702, #99564, #35801, #11114, #78566, #66974, #89424, #134378, #122762, #67718, #69126, #10420, #37188, #70579, #71993, #15396, #38623, #82853, #103155, #3118, #16870, #48080, #127037, #93000, #113304, #69859, #81441, #16110, #13982, #126335, #5948, #39353, #59678, #47409, #83572, #3794, #116176, #61144, #60398, #105293, #91575, #103837, #137945, #14723, #27735, #92262, #127786, #71265, #94411, #28472, #58285, #114031, #125642, #5247, #4488, #114724, #48793, #137227, #50221, #26322, #138660, #37926, #104584, #82157, #135793, #102471, #59000, #36478, #27019, #80717, #115417, #124913, #25583, #49531, #136491, #93716, #19707, #40771, #107433, #140762, #128492, #87118, #140091, #96525, #8096, #129905, #9519, #85670, #42919, #51649, #29862, #53040, #97994, #19002, #53797, #84974, #74105, #42205, #142235, #50933, #97237, #73402, #118296, #18249, #131334, #29163, #75536, #30616, #63948, #8780, #129176, #95844, #141502, #62530, #86421, #72732, #74844, #63266, #130648, #105979, #106695, #52338, #108117, #41455, #119021, #31317, #119706, #20404, #116885, #17557, #7389, #64652, #108833, #61821, #6649, #95123, #117566, #139395, #40082, #84296, #100844, #76249, #10250, #78389, #13099, #46520, #34896, #133487, #67533, #22535, #132799, #121856, #55939, #1498, #123338, #111729, #100142, #43603, #110268, #87825, #134200, #132065, #90703, #76990, #66795, #45784, #32755, #79133, #33482, #32018, #121156, #122581, #55, #110974, #24006, #142921, #68264, #21852, #66097, #88565, #112440, #57369, #101544, #2198, #120410, #23257, #44352, #54511, #21137, #65397, #99384, #77684, #89948, #109574, #98692, #10943, #11655, #55208, #792, #89259, #45086, #34172, #12395, #56679, #13801, #115975, #47927, #102298, #136317, #91412, #124032, #27542, #105123, #124736, #25403, #68960, #35627, #60215, #38451, #69677, #36312, #82674, #79858, #15229, #135625, #58096, #71096, #2945, #24704, #47241, #37006, #58829, #92091, #113130, #113854, #137043, #125462, #115238, #80540, #81257, #14550, #50047, #102991, #137773, #92812, #81987, #15925, #3627, #26145, #70415, #114560, #26844, #59508, #103665, #5781, #4306, #48609, #37750, #126173, #104396, #134938, #5058, #49356, #93541, #126856, #71810, #16678, #60964, #28290, #118851, #51474, #72552, #116716, #106518, #95667, #17394, #52859, #139922, #19539, #63785, #84122, #127600, #141316, #28999, #107942, #73928, #94241, #50751, #62358, #140596, #138479, #107254, #130468, #20233, #8614, #39164, #64478, #128324, #97054, #42030, #41284, #86245, #61651, #40599, #31155, #139209, #75367, #73232, #108653, #52168, #119535, #9334, #83385, #94941, #129721, #18071 ),
 .UNSPECIFIED., .F., .T. ) 
 B_SPLINE_CURVE_WITH_KNOTS ( ( 3, 2, 2, 2, 2, 2, 2, 2, 2, 2, 2, 2, 2, 2, 2, 2, 2, 2, 2, 2, 2, 2, 2, 2, 2, 2, 2, 2, 2, 2, 2, 2, 2, 2, 2, 2, 2, 2, 2, 2, 2, 2, 2, 2, 2, 2, 2, 2, 2, 2, 2, 2, 2, 2, 2, 2, 2, 2, 2, 2, 2, 2, 2, 2, 2, 2, 2, 2, 2, 2, 2, 2, 2, 2, 2, 2, 2, 2, 2, 2, 2, 2, 2, 2, 2, 2, 2, 2, 2, 2, 2, 2, 2, 2, 2, 2, 2, 2, 2, 2, 2, 2, 2, 2, 2, 2, 2, 2, 2, 2, 2, 2, 2, 2, 2, 2, 2, 2, 2, 2, 2, 2, 2, 2, 2, 2, 2, 2, 2, 2, 2, 2, 2, 2, 2, 2, 2, 2, 2, 2, 2, 2, 2, 2, 2, 2, 2, 2, 2, 2, 2, 2, 2, 2, 2, 2, 2, 2, 2, 2, 2, 2, 2, 2, 2, 2, 2, 2, 2, 2, 2, 2, 2, 2, 2, 2, 2, 2, 2, 2, 2, 2, 2, 2, 2, 2, 2, 2, 2, 2, 2, 2, 2, 2, 2, 2, 2, 2, 2, 2, 2, 2, 2, 2, 2, 2, 2, 2, 2, 2, 2, 2, 2, 2, 2, 2, 2, 2, 2, 2, 2, 2, 2, 2, 2, 2, 2, 2, 2, 2, 2, 2, 2, 2, 2, 2, 2, 2, 2, 2, 2, 2, 2, 2, 2, 2, 2, 2, 2, 2, 2, 2, 2, 2, 2, 2, 2, 2, 2, 2, 2, 2, 2, 2, 2, 2, 2, 2, 2, 2, 2, 2, 2, 2, 2, 2, 2, 2, 2, 2, 2, 2, 2, 2, 2, 2, 2, 2, 2, 2, 2, 2, 2, 2, 2, 2, 2, 2, 2, 2, 2, 2, 2, 2, 2, 2, 2, 2, 2, 2, 2, 2, 2, 2, 2, 2, 2, 2, 2, 2, 2, 2, 2, 2, 2, 2, 2, 2, 2, 2, 2, 2, 2, 2, 2, 2, 2, 2, 2, 2, 2, 2, 2, 2, 2, 2, 2, 2, 2, 2, 2, 3 ),
 ( 0.000000000000000000, 0.002777777777777777884, 0.005555555555555555768, 0.008333333333333333218, 0.01111111111111111154, 0.01388888888888888812, 0.01666666666666666644, 0.01944444444444444475, 0.02222222222222222307, 0.02500000000000000139, 0.02777777777777777624, 0.03055555555555555455, 0.03333333333333333287, 0.03611111111111110772, 0.03888888888888888951, 0.04166666666666666435, 0.04444444444444444614, 0.04722222222222222099, 0.05000000000000000278, 0.05277777777777777762, 0.05555555555555555247, 0.05833333333333333426, 0.06111111111111110911, 0.06388888888888888395, 0.06666666666666666574, 0.06944444444444444753, 0.07222222222222221544, 0.07499999999999999722, 0.07777777777777777901, 0.08055555555555556080, 0.08333333333333332871, 0.08611111111111111049, 0.08888888888888889228, 0.09166666666666666019, 0.09444444444444444198, 0.09722222222222222376, 0.1000000000000000056, 0.1027777777777777735, 0.1055555555555555552, 0.1083333333333333370, 0.1111111111111111049, 0.1138888888888888867, 0.1166666666666666685, 0.1194444444444444503, 0.1222222222222222182, 0.1250000000000000000, 0.1277777777777777679, 0.1305555555555555636, 0.1333333333333333315, 0.1361111111111110994, 0.1388888888888888951, 0.1416666666666666630, 0.1444444444444444309, 0.1472222222222222265, 0.1499999999999999944, 0.1527777777777777901, 0.1555555555555555580, 0.1583333333333333259, 0.1611111111111111216, 0.1638888888888888895, 0.1666666666666666574, 0.1694444444444444531, 0.1722222222222222210, 0.1750000000000000167, 0.1777777777777777846, 0.1805555555555555525, 0.1833333333333333204, 0.1861111111111111160, 0.1888888888888888840, 0.1916666666666666796, 0.1944444444444444475, 0.1972222222222222154, 0.2000000000000000111, 0.2027777777777777790, 0.2055555555555555469, 0.2083333333333333426, 0.2111111111111111105, 0.2138888888888888784, 0.2166666666666666741, 0.2194444444444444420, 0.2222222222222222099, 0.2249999999999999778, 0.2277777777777777735, 0.2305555555555555691, 0.2333333333333333370, 0.2361111111111111049, 0.2388888888888889006, 0.2416666666666666685, 0.2444444444444444364, 0.2472222222222222321, 0.2500000000000000000, 0.2527777777777777679, 0.2555555555555555358, 0.2583333333333333592, 0.2611111111111111271, 0.2638888888888888951, 0.2666666666666666630, 0.2694444444444444309, 0.2722222222222221988, 0.2750000000000000222, 0.2777777777777777901, 0.2805555555555555580, 0.2833333333333333259, 0.2861111111111110938, 0.2888888888888888618, 0.2916666666666666852, 0.2944444444444444531, 0.2972222222222222210, 0.2999999999999999889, 0.3027777777777777568, 0.3055555555555555802, 0.3083333333333333481, 0.3111111111111111160, 0.3138888888888888840, 0.3166666666666666519, 0.3194444444444444198, 0.3222222222222222432, 0.3250000000000000111, 0.3277777777777777790, 0.3305555555555555469, 0.3333333333333333148, 0.3361111111111111382, 0.3388888888888889062, 0.3416666666666666741, 0.3444444444444444420, 0.3472222222222222099, 0.3500000000000000333, 0.3527777777777778012, 0.3555555555555555691, 0.3583333333333333370, 0.3611111111111111049, 0.3638888888888888729, 0.3666666666666666408, 0.3694444444444444642, 0.3722222222222222321, 0.3750000000000000000, 0.3777777777777777679, 0.3805555555555555358, 0.3833333333333333592, 0.3861111111111111271, 0.3888888888888888951, 0.3916666666666666630, 0.3944444444444444309, 0.3972222222222221988, 0.4000000000000000222, 0.4027777777777777901, 0.4055555555555555580, 0.4083333333333333259, 0.4111111111111110938, 0.4138888888888888618, 0.4166666666666666852, 0.4194444444444444531, 0.4222222222222222210, 0.4249999999999999889, 0.4277777777777777568, 0.4305555555555555802, 0.4333333333333333481, 0.4361111111111111160, 0.4388888888888888840, 0.4416666666666666519, 0.4444444444444444198, 0.4472222222222222432, 0.4499999999999999556, 0.4527777777777777790, 0.4555555555555555469, 0.4583333333333333148, 0.4611111111111111382, 0.4638888888888889062, 0.4666666666666666741, 0.4694444444444444420, 0.4722222222222222099, 0.4749999999999999778, 0.4777777777777778012, 0.4805555555555555691, 0.4833333333333333370, 0.4861111111111111049, 0.4888888888888888729, 0.4916666666666666408, 0.4944444444444444642, 0.4972222222222222321, 0.5000000000000000000, 0.5027777777777777679, 0.5055555555555555358, 0.5083333333333333037, 0.5111111111111110716, 0.5138888888888888395, 0.5166666666666667185, 0.5194444444444444864, 0.5222222222222222543, 0.5250000000000000222, 0.5277777777777777901, 0.5305555555555555580, 0.5333333333333333259, 0.5361111111111110938, 0.5388888888888888618, 0.5416666666666666297, 0.5444444444444443976, 0.5472222222222222765, 0.5500000000000000444, 0.5527777777777778123, 0.5555555555555555802, 0.5583333333333333481, 0.5611111111111111160, 0.5638888888888888840, 0.5666666666666666519, 0.5694444444444444198, 0.5722222222222221877, 0.5749999999999999556, 0.5777777777777777235, 0.5805555555555556024, 0.5833333333333333703, 0.5861111111111112493, 0.5888888888888889062, 0.5916666666666666741, 0.5944444444444444420, 0.5972222222222222099, 0.5999999999999999778, 0.6027777777777777457, 0.6055555555555555136, 0.6083333333333332815, 0.6111111111111111605, 0.6138888888888889284, 0.6166666666666666963, 0.6194444444444444642, 0.6222222222222222321, 0.6250000000000000000, 0.6277777777777777679, 0.6305555555555555358, 0.6333333333333333037, 0.6361111111111110716, 0.6388888888888888395, 0.6416666666666667185, 0.6444444444444444864, 0.6472222222222222543, 0.6500000000000000222, 0.6527777777777777901, 0.6555555555555555580, 0.6583333333333333259, 0.6611111111111110938, 0.6638888888888888618, 0.6666666666666666297, 0.6694444444444443976, 0.6722222222222222765, 0.6750000000000000444, 0.6777777777777778123, 0.6805555555555555802, 0.6833333333333333481, 0.6861111111111111160, 0.6888888888888888840, 0.6916666666666666519, 0.6944444444444444198, 0.6972222222222221877, 0.7000000000000000666, 0.7027777777777777235, 0.7055555555555556024, 0.7083333333333333703, 0.7111111111111111382, 0.7138888888888889062, 0.7166666666666666741, 0.7194444444444444420, 0.7222222222222222099, 0.7249999999999999778, 0.7277777777777777457, 0.7305555555555555136, 0.7333333333333332815, 0.7361111111111111605, 0.7388888888888889284, 0.7416666666666666963, 0.7444444444444444642, 0.7472222222222222321, 0.7500000000000000000, 0.7527777777777777679, 0.7555555555555555358, 0.7583333333333333037, 0.7611111111111110716, 0.7638888888888888395, 0.7666666666666667185, 0.7694444444444444864, 0.7722222222222222543, 0.7750000000000000222, 0.7777777777777777901, 0.7805555555555555580, 0.7833333333333333259, 0.7861111111111110938, 0.7888888888888888618, 0.7916666666666666297, 0.7944444444444443976, 0.7972222222222222765, 0.8000000000000000444, 0.8027777777777778123, 0.8055555555555555802, 0.8083333333333333481, 0.8111111111111111160, 0.8138888888888888840, 0.8166666666666666519, 0.8194444444444444198, 0.8222222222222221877, 0.8249999999999999556, 0.8277777777777777235, 0.8305555555555556024, 0.8333333333333333703, 0.8361111111111111382, 0.8388888888888889062, 0.8416666666666666741, 0.8444444444444444420, 0.8472222222222222099, 0.8499999999999999778, 0.8527777777777777457, 0.8555555555555555136, 0.8583333333333332815, 0.8611111111111111605, 0.8638888888888889284, 0.8666666666666666963, 0.8694444444444444642, 0.8722222222222222321, 0.8750000000000000000, 0.8777777777777777679, 0.8805555555555555358, 0.8833333333333333037, 0.8861111111111110716, 0.8888888888888888395, 0.8916666666666667185, 0.8944444444444444864, 0.8972222222222222543, 0.8999999999999999112, 0.9027777777777777901, 0.9055555555555555580, 0.9083333333333333259, 0.9111111111111110938, 0.9138888888888888618, 0.9166666666666666297, 0.9194444444444443976, 0.9222222222222222765, 0.9250000000000000444, 0.9277777777777778123, 0.9305555555555555802, 0.9333333333333333481, 0.9361111111111111160, 0.9388888888888888840, 0.9416666666666666519, 0.9444444444444444198, 0.9472222222222221877, 0.9499999999999999556, 0.9527777777777777235, 0.9555555555555556024, 0.9583333333333333703, 0.9611111111111111382, 0.9638888888888889062, 0.9666666666666666741, 0.9694444444444444420, 0.9722222222222222099, 0.9749999999999999778 ),
 .UNSPECIFIED. ) 
 CURVE ( )  GEOMETRIC_REPRESENTATION_ITEM ( )  RATIONAL_B_SPLINE_CURVE ( ( 1.000000000000000000, 0.9659258262890683122, 1.000000000000000000, 0.9659258262890683122, 1.000000000000000000, 0.9659258262890683122, 1.000000000000000000, 0.9659258262890683122, 1.000000000000000000, 0.9659258262890683122, 1.000000000000000000, 0.9659258262890683122, 1.000000000000000000, 0.9659258262890683122, 1.000000000000000000, 0.9659258262890683122, 1.000000000000000000, 0.9659258262890683122, 1.000000000000000000, 0.9659258262890683122, 1.000000000000000000, 0.9659258262890683122, 1.000000000000000000, 0.9659258262890683122, 1.000000000000000000, 0.9659258262890683122, 1.000000000000000000, 0.9659258262890683122, 1.000000000000000000, 0.9659258262890683122, 1.000000000000000000, 0.9659258262890683122, 1.000000000000000000, 0.9659258262890683122, 1.000000000000000000, 0.9659258262890683122, 1.000000000000000000, 0.9659258262890683122, 1.000000000000000000, 0.9659258262890683122, 1.000000000000000000, 0.9659258262890683122, 1.000000000000000000, 0.9659258262890683122, 1.000000000000000000, 0.9659258262890683122, 1.000000000000000000, 0.9659258262890683122, 1.000000000000000000, 0.9659258262890683122, 1.000000000000000000, 0.9659258262890683122, 1.000000000000000000, 0.9659258262890683122, 1.000000000000000000, 0.9659258262890683122, 1.000000000000000000, 0.9659258262890683122, 1.000000000000000000, 0.9659258262890683122, 1.000000000000000000, 0.9659258262890683122, 1.000000000000000000, 0.9659258262890683122, 1.000000000000000000, 0.9659258262890683122, 1.000000000000000000, 0.9659258262890683122, 1.000000000000000000, 0.9659258262890683122, 1.000000000000000000, 0.9659258262890683122, 1.000000000000000000, 0.9659258262890683122, 1.000000000000000000, 0.9659258262890683122, 1.000000000000000000, 0.9659258262890683122, 1.000000000000000000, 0.9659258262890683122, 1.000000000000000000, 0.9659258262890683122, 1.000000000000000000, 0.9659258262890683122, 1.000000000000000000, 0.9659258262890683122, 1.000000000000000000, 0.9659258262890683122, 1.000000000000000000, 0.9659258262890683122, 1.000000000000000000, 0.9659258262890683122, 1.000000000000000000, 0.9659258262890683122, 1.000000000000000000, 0.9659258262890683122, 1.000000000000000000, 0.9659258262890683122, 1.000000000000000000, 0.9659258262890683122, 1.000000000000000000, 0.9659258262890683122, 1.000000000000000000, 0.9659258262890683122, 1.000000000000000000, 0.9659258262890683122, 1.000000000000000000, 0.9659258262890683122, 1.000000000000000000, 0.9659258262890683122, 1.000000000000000000, 0.9659258262890683122, 1.000000000000000000, 0.9659258262890683122, 1.000000000000000000, 0.9659258262890683122, 1.000000000000000000, 0.9659258262890683122, 1.000000000000000000, 0.9659258262890683122, 1.000000000000000000, 0.9659258262890683122, 1.000000000000000000, 0.9659258262890683122, 1.000000000000000000, 0.9659258262890683122, 1.000000000000000000, 0.9659258262890683122, 1.000000000000000000, 0.9659258262890683122, 1.000000000000000000, 0.9659258262890683122, 1.000000000000000000, 0.9659258262890683122, 1.000000000000000000, 0.9659258262890683122, 1.000000000000000000, 0.9659258262890683122, 1.000000000000000000, 0.9659258262890683122, 1.000000000000000000, 0.9659258262890683122, 1.000000000000000000, 0.9659258262890683122, 1.000000000000000000, 0.9659258262890683122, 1.000000000000000000, 0.9659258262890683122, 1.000000000000000000, 0.9659258262890683122, 1.000000000000000000, 0.9659258262890683122, 1.000000000000000000, 0.9659258262890683122, 1.000000000000000000, 0.9659258262890683122, 1.000000000000000000, 0.9659258262890683122, 1.000000000000000000, 0.9659258262890683122, 1.000000000000000000, 0.9659258262890683122, 1.000000000000000000, 0.9659258262890683122, 1.000000000000000000, 0.9659258262890683122, 1.000000000000000000, 0.9659258262890683122, 1.000000000000000000, 0.9659258262890683122, 1.000000000000000000, 0.9659258262890683122, 1.000000000000000000, 0.9659258262890683122, 1.000000000000000000, 0.9659258262890683122, 1.000000000000000000, 0.9659258262890683122, 1.000000000000000000, 0.9659258262890683122, 1.000000000000000000, 0.9659258262890683122, 1.000000000000000000, 0.9659258262890683122, 1.000000000000000000, 0.9659258262890683122, 1.000000000000000000, 0.9659258262890683122, 1.000000000000000000, 0.9659258262890683122, 1.000000000000000000, 0.9659258262890683122, 1.000000000000000000, 0.9659258262890683122, 1.000000000000000000, 0.9659258262890683122, 1.000000000000000000, 0.9659258262890683122, 1.000000000000000000, 0.9659258262890683122, 1.000000000000000000, 0.9659258262890683122, 1.000000000000000000, 0.9659258262890683122, 1.000000000000000000, 0.9659258262890683122, 1.000000000000000000, 0.9659258262890683122, 1.000000000000000000, 0.9659258262890683122, 1.000000000000000000, 0.9659258262890683122, 1.000000000000000000, 0.9659258262890683122, 1.000000000000000000, 0.9659258262890683122, 1.000000000000000000, 0.9659258262890683122, 1.000000000000000000, 0.9659258262890683122, 1.000000000000000000, 0.9659258262890683122, 1.000000000000000000, 0.9659258262890683122, 1.000000000000000000, 0.9659258262890683122, 1.000000000000000000, 0.9659258262890683122, 1.000000000000000000, 0.9659258262890683122, 1.000000000000000000, 0.9659258262890683122, 1.000000000000000000, 0.9659258262890683122, 1.000000000000000000, 0.9659258262890683122, 1.000000000000000000, 0.9659258262890683122, 1.000000000000000000, 0.9659258262890683122, 1.000000000000000000, 0.9659258262890683122, 1.000000000000000000, 0.9659258262890683122, 1.000000000000000000, 0.9659258262890683122, 1.000000000000000000, 0.9659258262890683122, 1.000000000000000000, 0.9659258262890683122, 1.000000000000000000, 0.9659258262890683122, 1.000000000000000000, 0.9659258262890683122, 1.000000000000000000, 0.9659258262890683122, 1.000000000000000000, 0.9659258262890683122, 1.000000000000000000, 0.9659258262890683122, 1.000000000000000000, 0.9659258262890683122, 1.000000000000000000, 0.9659258262890683122, 1.000000000000000000, 0.9659258262890683122, 1.000000000000000000, 0.9659258262890683122, 1.000000000000000000, 0.9659258262890683122, 1.000000000000000000, 0.9659258262890683122, 1.000000000000000000, 0.9659258262890683122, 1.000000000000000000, 0.9659258262890683122, 1.000000000000000000, 0.9659258262890683122, 1.000000000000000000, 0.9659258262890683122, 1.000000000000000000, 0.9659258262890683122, 1.000000000000000000, 0.9659258262890683122, 1.000000000000000000, 0.9659258262890683122, 1.000000000000000000, 0.9659258262890683122, 1.000000000000000000, 0.9659258262890683122, 1.000000000000000000, 0.9659258262890683122, 1.000000000000000000, 0.9659258262890683122, 1.000000000000000000, 0.9659258262890683122, 1.000000000000000000, 0.9659258262890683122, 1.000000000000000000, 0.9659258262890683122, 1.000000000000000000, 0.9659258262890683122, 1.000000000000000000, 0.9659258262890683122, 1.000000000000000000, 0.9659258262890683122, 1.000000000000000000, 0.9659258262890683122, 1.000000000000000000, 0.9659258262890683122, 1.000000000000000000, 0.9659258262890683122, 1.000000000000000000, 0.9659258262890683122, 1.000000000000000000, 0.9659258262890683122, 1.000000000000000000, 0.9659258262890683122, 1.000000000000000000, 0.9659258262890683122, 1.000000000000000000, 0.9659258262890683122, 1.000000000000000000, 0.9659258262890683122, 1.000000000000000000, 0.9659258262890683122, 1.000000000000000000, 0.9659258262890683122, 1.000000000000000000, 0.9659258262890683122, 1.000000000000000000, 0.9659258262890683122, 1.000000000000000000, 0.9659258262890683122, 1.000000000000000000, 0.9659258262890683122, 1.000000000000000000, 0.9659258262890683122, 1.000000000000000000, 0.9659258262890683122, 1.000000000000000000, 0.9659258262890683122, 1.000000000000000000, 0.9659258262890683122, 1.000000000000000000, 0.9659258262890683122, 1.000000000000000000, 0.9659258262890683122, 1.000000000000000000, 0.9659258262890683122, 1.000000000000000000, 0.9659258262890683122, 1.000000000000000000, 0.9659258262890683122, 1.000000000000000000, 0.9659258262890683122, 1.000000000000000000, 0.9659258262890683122, 1.000000000000000000, 0.9659258262890683122, 1.000000000000000000, 0.9659258262890683122, 1.000000000000000000, 0.9659258262890683122, 1.000000000000000000, 0.9659258262890683122, 1.000000000000000000, 0.9659258262890683122, 1.000000000000000000, 0.9659258262890683122, 1.000000000000000000, 0.9659258262890683122, 1.000000000000000000, 0.9659258262890683122, 1.000000000000000000, 0.9659258262890683122, 1.000000000000000000, 0.9659258262890683122, 1.000000000000000000, 0.9659258262890683122, 1.000000000000000000, 0.9659258262890683122, 1.000000000000000000, 0.9659258262890683122, 1.000000000000000000, 0.9659258262890683122, 1.000000000000000000, 0.9659258262890683122, 1.000000000000000000, 0.9659258262890683122, 1.000000000000000000, 0.9659258262890683122, 1.000000000000000000, 0.9659258262890683122, 1.000000000000000000, 0.9659258262890683122, 1.000000000000000000, 0.9659258262890683122, 1.000000000000000000, 0.9659258262890683122, 1.000000000000000000, 0.9659258262890683122, 1.000000000000000000, 0.9659258262890683122, 1.000000000000000000, 0.9659258262890683122, 1.000000000000000000, 0.9659258262890683122, 1.000000000000000000, 0.9659258262890683122, 1.000000000000000000, 0.9659258262890683122, 1.000000000000000000, 0.9659258262890683122, 1.000000000000000000, 0.9659258262890683122, 1.000000000000000000, 0.9659258262890683122, 1.000000000000000000, 0.9659258262890683122, 1.000000000000000000, 0.9659258262890683122, 1.000000000000000000, 0.9659258262890683122, 1.000000000000000000, 0.9659258262890683122, 1.000000000000000000, 0.9659258262890683122, 1.000000000000000000, 0.9659258262890683122, 1.000000000000000000, 0.9659258262890683122, 1.000000000000000000, 0.9659258262890683122, 1.000000000000000000, 0.9659258262890683122, 1.000000000000000000, 0.9659258262890683122, 1.000000000000000000, 0.9659258262890683122, 1.000000000000000000, 0.9659258262890683122, 1.000000000000000000, 0.9659258262890683122, 1.000000000000000000, 0.9659258262890683122, 1.000000000000000000, 0.9659258262890683122, 1.000000000000000000, 0.9659258262890683122, 1.000000000000000000, 0.9659258262890683122, 1.000000000000000000, 0.9659258262890683122, 1.000000000000000000, 0.9659258262890683122, 1.000000000000000000, 0.9659258262890683122, 1.000000000000000000, 0.9659258262890683122, 1.000000000000000000, 0.9659258262890683122, 1.000000000000000000, 0.9659258262890683122, 1.000000000000000000, 0.9659258262890683122, 1.000000000000000000, 0.9659258262890683122, 1.000000000000000000, 0.9659258262890683122, 1.000000000000000000, 0.9659258262890683122, 1.000000000000000000, 0.9659258262890683122, 1.000000000000000000, 0.9659258262890683122, 1.000000000000000000, 0.9659258262890683122, 1.000000000000000000, 0.9659258262890683122, 1.000000000000000000, 0.9659258262890683122, 1.000000000000000000, 0.9659258262890683122, 1.000000000000000000, 0.9659258262890683122, 1.000000000000000000, 0.9659258262890683122, 1.000000000000000000, 0.9659258262890683122, 1.000000000000000000, 0.9659258262890683122, 1.000000000000000000, 0.9659258262890683122, 1.000000000000000000, 0.9659258262890683122, 1.000000000000000000, 0.9659258262890683122, 1.000000000000000000, 0.9659258262890683122, 1.000000000000000000, 0.9659258262890683122, 1.000000000000000000, 0.9659258262890683122, 1.000000000000000000, 0.9659258262890683122, 1.000000000000000000, 0.9659258262890683122, 1.000000000000000000, 0.9659258262890683122, 1.000000000000000000, 0.9659258262890683122, 1.000000000000000000, 0.9659258262890683122, 1.000000000000000000, 0.9659258262890683122, 1.000000000000000000, 0.9659258262890683122, 1.000000000000000000, 0.9659258262890683122, 1.000000000000000000, 0.9659258262890683122, 1.000000000000000000, 0.9659258262890683122, 1.000000000000000000, 0.9659258262890683122, 1.000000000000000000, 0.9659258262890683122, 1.000000000000000000, 0.9659258262890683122, 1.000000000000000000, 0.9659258262890683122, 1.000000000000000000, 0.9659258262890683122, 1.000000000000000000, 0.9659258262890683122, 1.000000000000000000, 0.9659258262890683122, 1.000000000000000000, 0.9659258262890683122, 1.000000000000000000, 0.9659258262890683122, 1.000000000000000000, 0.9659258262890683122, 1.000000000000000000, 0.9659258262890683122, 1.000000000000000000, 0.9659258262890683122, 1.000000000000000000, 0.9659258262890683122, 1.000000000000000000, 0.9659258262890683122, 1.000000000000000000, 0.9659258262890683122, 1.000000000000000000, 0.9659258262890683122, 1.000000000000000000, 0.9659258262890683122, 1.000000000000000000, 0.9659258262890683122, 1.000000000000000000, 0.9659258262890683122, 1.000000000000000000, 0.9659258262890683122, 1.000000000000000000, 0.9659258262890683122, 1.000000000000000000, 0.9659258262890683122, 1.000000000000000000, 0.9659258262890683122, 1.000000000000000000, 0.9659258262890683122, 1.000000000000000000, 0.9659258262890683122, 1.000000000000000000, 0.9659258262890683122, 1.000000000000000000, 0.9659258262890683122, 1.000000000000000000, 0.9659258262890683122, 1.000000000000000000, 0.9659258262890683122, 1.000000000000000000, 0.9659258262890683122, 1.000000000000000000, 0.9659258262890683122, 1.000000000000000000, 0.9659258262890683122, 1.000000000000000000, 0.9659258262890683122, 1.000000000000000000, 0.9659258262890683122, 1.000000000000000000, 0.9659258262890683122, 1.000000000000000000, 0.9659258262890683122, 1.000000000000000000, 0.9659258262890683122, 1.000000000000000000, 0.9659258262890683122, 1.000000000000000000, 0.9659258262890683122, 1.000000000000000000, 0.9659258262890683122, 1.000000000000000000, 0.9659258262890683122, 1.000000000000000000, 0.9659258262890683122, 1.000000000000000000, 0.9659258262890683122, 1.000000000000000000, 0.9659258262890683122, 1.000000000000000000, 0.9659258262890683122, 1.000000000000000000, 0.9659258262890683122, 1.000000000000000000, 0.9659258262890683122, 1.000000000000000000, 0.9659258262890683122, 1.000000000000000000, 0.9659258262890683122, 1.000000000000000000, 0.9659258262890683122, 1.000000000000000000, 0.9659258262890683122, 1.000000000000000000, 0.9659258262890683122, 1.000000000000000000, 0.9659258262890683122, 1.000000000000000000, 0.9659258262890683122, 1.000000000000000000, 0.9659258262890683122, 1.000000000000000000, 0.9659258262890683122, 1.000000000000000000, 0.9659258262890683122, 1.000000000000000000, 0.9659258262890683122, 1.000000000000000000, 0.9659258262890683122, 1.000000000000000000, 0.9659258262890683122, 1.000000000000000000, 0.9659258262890683122, 1.000000000000000000, 0.9659258262890683122, 1.000000000000000000, 0.9659258262890683122, 1.000000000000000000, 0.9659258262890683122, 1.000000000000000000, 0.9659258262890683122, 1.000000000000000000, 0.9659258262890683122, 1.000000000000000000, 0.9659258262890683122, 1.000000000000000000, 0.9659258262890683122, 1.000000000000000000, 0.9659258262890683122, 1.000000000000000000, 0.9659258262890683122, 1.000000000000000000, 0.9659258262890683122, 1.000000000000000000, 0.9659258262890683122, 1.000000000000000000, 0.9659258262890683122, 1.000000000000000000, 0.9659258262890683122, 1.000000000000000000, 0.9659258262890683122, 1.000000000000000000, 0.9659258262890683122, 1.000000000000000000, 0.9659258262890683122, 1.000000000000000000, 0.9659258262890683122, 1.000000000000000000, 0.9659258262890683122, 1.000000000000000000, 0.9659258262890683122, 1.000000000000000000, 0.9659258262890683122, 1.000000000000000000, 0.9659258262890683122, 1.000000000000000000, 0.9659258262890683122, 1.000000000000000000, 0.9659258262890683122, 1.000000000000000000, 0.9659258262890683122, 1.000000000000000000, 0.9659258262890683122, 1.000000000000000000, 0.9659258262890683122, 1.000000000000000000, 0.9659258262890683122, 1.000000000000000000, 0.9659258262890683122, 1.000000000000000000 ) ) 
 REPRESENTATION_ITEM ( '' )  );
#110135=CARTESIAN_POINT ( 'NONE',  ( 82.45376352523145158, -6.109999999999999432, -3.741295971395163529E-16 ) ) ;
#110136=CARTESIAN_POINT ( 'NONE',  ( 5.979043268340604733, -9.486524475911640053, -0.5800208356449471081 ) ) ;
#110188=CARTESIAN_POINT ( 'NONE',  ( 98.41666666666667140, -6.884901960086287076, -3.975000000000000977 ) ) ;
#110211=CARTESIAN_POINT ( 'NONE',  ( 121.6254301918981184, 5.291415217122919401, 3.055000000000002824 ) ) ;
#110219=CARTESIAN_POINT ( 'NONE',  ( 117.0162635252314374, -4.472830434245839371, 4.472830434245839371 ) ) ;
#110225=CARTESIAN_POINT ( 'NONE',  ( 39.81293019189809712, -1.637169565754159617, -6.110000000000001208 ) ) ;
#110233=CARTESIAN_POINT ( 'NONE',  ( 29.51626352523143737, -4.472830434245839371, 4.472830434245839371 ) ) ;
#110268=CARTESIAN_POINT ( 'NONE',  ( 49.34959685856478728, 6.109999999999996767, 1.637169565754163836 ) ) ;
#110301=CARTESIAN_POINT ( 'NONE',  ( 123.4329301918981088, 1.637169565754156730, 6.110000000000001208 ) ) ;
#110308=CARTESIAN_POINT ( 'NONE',  ( 67.89169371712955581, 2.130196079827421762, 7.950000000000000178 ) ) ;
#110343=CARTESIAN_POINT ( 'NONE',  ( 27.91209685856478728, 5.291415217122922066, -3.054999999999995275 ) ) ;
#110360=CARTESIAN_POINT ( 'NONE',  ( 119.0004301918981184, -3.055000000000002380, 5.291415217122920289 ) ) ;
#110372=CARTESIAN_POINT ( 'NONE',  ( 61.18336038379622011, -2.130196079827426203, 7.949999999999997513 ) ) ;
#110378=CARTESIAN_POINT ( 'NONE',  ( 46.20833333333332149, -3.974999999999999201, -6.884901960086287964 ) ) ;
#110387=CARTESIAN_POINT ( 'NONE',  ( 34.12543019189810423, 5.291415217122919401, 3.055000000000002824 ) ) ;
#110400=CARTESIAN_POINT ( 'NONE',  ( 82.97959685856476142, 6.109999999999999432, 1.637169565754164280 ) ) ;
#110401=CARTESIAN_POINT ( 'NONE',  ( 127.1386022459138019, -7.776507174585692163E-16, 6.349999999999999645 ) ) ;
#110410=CARTESIAN_POINT ( 'NONE',  ( 68.30793019189809456, -6.109999999999998543, 1.637169565754158063 ) ) ;
#110440=CARTESIAN_POINT ( 'NONE',  ( 73.84959685856479439, 6.109999999999996767, 1.637169565754163836 ) ) ;
#110446=CARTESIAN_POINT ( 'NONE',  ( 123.5000000000000000, 0.000000000000000000, -7.950000000000000178 ) ) ;
#110462=CARTESIAN_POINT ( 'NONE',  ( 30.04209685856476497, 5.291415217122923842, -3.054999999999996163 ) ) ;
#110481=CARTESIAN_POINT ( 'NONE',  ( 30.75000000000000000, -9.735942053221458872E-16, 7.950000000000000178 ) ) ;
#110500=CARTESIAN_POINT ( 'NONE',  ( 25.89892480454907542, 0.000000000000000000, -6.350000000000003197 ) ) ;
#110510=CARTESIAN_POINT ( 'NONE',  ( 112.7083333333333286, -3.974999999999999201, -6.884901960086287964 ) ) ;
#110513=CARTESIAN_POINT ( 'NONE',  ( 53.35416666666665719, -2.130196079827501698, -7.949999999999956657 ) ) ;
#110515=CARTESIAN_POINT ( 'NONE',  ( 68.16209685856478018, -5.291415217122919401, 3.054999999999998384 ) ) ;
#110521=EDGE_CURVE ( 'NONE', #142459, #95449, #58536, .T. ) ;
#110540=CARTESIAN_POINT ( 'NONE',  ( 81.89169371712955581, 2.130196079827421762, 7.950000000000001066 ) ) ;
#110543=ORIENTED_EDGE ( 'NONE', *, *, #73633, .T. ) ;
#110545=CARTESIAN_POINT ( 'NONE',  ( 69.68750000000000000, -5.819803920172573086, 5.819803920172572198 ) ) ;
#110555=CARTESIAN_POINT ( 'NONE',  ( 77.72959685856477563, -6.110000000000000320, -1.637169565754161393 ) ) ;
#110569=CARTESIAN_POINT ( 'NONE',  ( 76.83333333333334281, -6.884901960086287964, 3.974999999999998312 ) ) ;
#110575=CARTESIAN_POINT ( 'NONE',  ( 62.12543019189810423, 5.291415217122919401, 3.055000000000002824 ) ) ;
#110582=CARTESIAN_POINT ( 'NONE',  ( 124.6208603837962272, -6.884901960086286188, 3.974999999999997424 ) ) ;
#110606=CARTESIAN_POINT ( 'NONE',  ( 98.93293019189810877, 1.637169565754156508, 6.110000000000000320 ) ) ;
#110624=CARTESIAN_POINT ( 'NONE',  ( 87.91666666666667140, -6.884901960086287076, -3.975000000000000977 ) ) ;
#110629=CARTESIAN_POINT ( 'NONE',  ( 56.58376352523143993, -6.110000000000001208, -3.741295971395164515E-16 ) ) ;
#110636=CARTESIAN_POINT ( 'NONE',  ( 91.58376352523144703, -6.110000000000001208, -3.741295971395164515E-16 ) ) ;
#110645=CARTESIAN_POINT ( 'NONE',  ( 0.000000000000000000, 9.735942053221458872E-16, -7.950000000000000178 ) ) ;
#110649=CARTESIAN_POINT ( 'NONE',  ( 124.7454301918981230, -5.291415217122918513, -3.055000000000000160 ) ) ;
#110670=CARTESIAN_POINT ( 'NONE',  ( 57.43750000000000000, 5.819803920172574863, -5.819803920172573086 ) ) ;
#110699=CARTESIAN_POINT ( 'NONE',  ( 114.5583603837962414, -7.949999999999997513, -2.130196079827425759 ) ) ;
#110708=DIRECTION ( 'NONE',  ( -1.000000000000000000, -0.000000000000000000, -0.000000000000000000 ) ) ;
#110712=ORIENTED_EDGE ( 'NONE', *, *, #3980, .F. ) ;
#110716=CARTESIAN_POINT ( 'NONE',  ( 103.9795968585647756, 6.109999999999999432, 1.637169565754164280 ) ) ;
#110738=CARTESIAN_POINT ( 'NONE',  ( 92.75043019189810423, 3.055000000000002824, -5.291415217122919401 ) ) ;
#110750=CARTESIAN_POINT ( 'NONE',  ( 89.45376352523146579, -6.109999999999998543, -3.741295971395162543E-16 ) ) ;
#110795=DIRECTION ( 'NONE',  ( -1.000000000000000000, -0.000000000000000000, -0.000000000000000000 ) ) ;
#110805=CARTESIAN_POINT ( 'NONE',  ( 125.2712635252314328, 4.472830434245838482, 4.472830434245842035 ) ) ;
#110820=ORIENTED_EDGE ( 'NONE', *, *, #88539, .F. ) ;
#110831=CARTESIAN_POINT ( 'NONE',  ( 80.41209685856479439, 5.291415217122922066, -3.054999999999995275 ) ) ;
#110846=CYLINDRICAL_SURFACE ( 'NONE', #63066, 6.350000000000004086 ) ;
#110887=CARTESIAN_POINT ( 'NONE',  ( 100.3124999999999858, 5.819803920172571310, 5.819803920172575751 ) ) ;
#110911=CARTESIAN_POINT ( 'NONE',  ( 86.41252705046289861, -7.949999999999998401, -4.867971026610728450E-16 ) ) ;
#110915=CARTESIAN_POINT ( 'NONE',  ( 117.5420968585647756, 5.291415217122923842, -3.054999999999996163 ) ) ;
#110924=CARTESIAN_POINT ( 'NONE',  ( 112.7870968585647802, 3.054999999999997495, 5.291415217122919401 ) ) ;
#110934=CARTESIAN_POINT ( 'NONE',  ( 35.14626352523143993, -4.472830434245840259, 4.472830434245839371 ) ) ;
#110943=DIRECTION ( 'NONE',  ( -1.000000000000000000, -0.000000000000000000, -0.000000000000000000 ) ) ;
#110974=CARTESIAN_POINT ( 'NONE',  ( 47.16209685856477307, -5.291415217122919401, 3.054999999999997939 ) ) ;
#111014=CARTESIAN_POINT ( 'NONE',  ( 109.8704301918981230, -3.055000000000001936, 5.291415217122918513 ) ) ;
#111035=DIRECTION ( 'NONE',  ( -1.000000000000000000, -0.000000000000000000, -0.000000000000000000 ) ) ;
#111051=CARTESIAN_POINT ( 'NONE',  ( 127.8291937171295558, -3.975000000000001865, 6.884901960086284411 ) ) ;
#111055=CARTESIAN_POINT ( 'NONE',  ( 127.0000000000000000, 0.000000000000000000, -7.950000000000000178 ) ) ;
#111056=EDGE_CURVE ( 'NONE', #7898, #75827, #63171, .T. ) ;
#111071=CARTESIAN_POINT ( 'NONE',  ( 122.5004301918981184, -3.055000000000002380, 5.291415217122920289 ) ) ;
#111074=CARTESIAN_POINT ( 'NONE',  ( 44.75000000000000000, -9.735942053221458872E-16, 7.950000000000000178 ) ) ;
#111082=CARTESIAN_POINT ( 'NONE',  ( 47.76669371712954870, -7.949999999999999289, 2.130196079827424427 ) ) ;
#111087=CARTESIAN_POINT ( 'NONE',  ( 44.89583333333332149, -2.130196079827427091, 7.949999999999999289 ) ) ;
#111095=CARTESIAN_POINT ( 'NONE',  ( 37.18793019189810423, 6.110000000000002984, -1.637169565754156730 ) ) ;
#111106=ORIENTED_EDGE ( 'NONE', *, *, #105221, .T. ) ;
#111110=CARTESIAN_POINT ( 'NONE',  ( 86.47959685856477563, 6.109999999999999432, 1.637169565754164280 ) ) ;
#111121=CARTESIAN_POINT ( 'NONE',  ( 58.82876352523144448, 0.000000000000000000, -6.109999999999998543 ) ) ;
#111129=FILL_AREA_STYLE ('',( #33627 ) ) ;
#111142=DIRECTION ( 'NONE',  ( -1.000000000000000000, -0.000000000000000000, -0.000000000000000000 ) ) ;
#111151=CARTESIAN_POINT ( 'NONE',  ( 74.57876352523145158, -7.482591942790325086E-16, 6.109999999999998543 ) ) ;
#111182=CARTESIAN_POINT ( 'NONE',  ( 29.60459685856477208, 1.637169565754164946, -6.109999999999999432 ) ) ;
#111231=CARTESIAN_POINT ( 'NONE',  ( 111.2500000000000000, -9.735942053221458872E-16, 7.950000000000000178 ) ) ;
#111236=EDGE_CURVE ( 'NONE', #135809, #5049, #13142, .T. ) ;
#111237=CARTESIAN_POINT ( 'NONE',  ( 60.43293019189810877, 1.637169565754156730, 6.110000000000001208 ) ) ;
#111238=DIRECTION ( 'NONE',  ( -1.000000000000000000, -0.000000000000000000, -0.000000000000000000 ) ) ;
#111251=DIRECTION ( 'NONE',  ( -1.000000000000000000, -0.000000000000000000, -0.000000000000000000 ) ) ;
#111262=CARTESIAN_POINT ( 'NONE',  ( 72.41252705046288440, -7.949999999999998401, -4.867971026610728450E-16 ) ) ;
#111266=CARTESIAN_POINT ( 'NONE',  ( 68.95833333333332860, 3.974999999999997424, 6.884901960086288852 ) ) ;
#111278=CARTESIAN_POINT ( 'NONE',  ( 63.00043019189810423, -3.055000000000002380, 5.291415217122920289 ) ) ;
#111299=CARTESIAN_POINT ( 'NONE',  ( 61.97959685856476852, 6.109999999999999432, 1.637169565754164280 ) ) ;
#111333=CARTESIAN_POINT ( 'NONE',  ( 104.9120968585647802, 5.291415217122921177, -3.054999999999994831 ) ) ;
#111359=CARTESIAN_POINT ( 'NONE',  ( 55.85459685856476142, -1.637169565754161615, 6.110000000000000320 ) ) ;
#111364=CARTESIAN_POINT ( 'NONE',  ( 88.52126352523143282, -4.472830434245838482, -4.472830434245840259 ) ) ;
#111373=( BOUNDED_CURVE ( )  B_SPLINE_CURVE ( 2, ( #49918, #138338, #18664, #32228, #76463, #130851, #56876, #12599, #23481, #9739, #43816, #99594, #111941 ),
 .UNSPECIFIED., .F., .F. ) 
 B_SPLINE_CURVE_WITH_KNOTS ( ( 3, 2, 2, 2, 2, 2, 3 ),
 ( 0.3666666666666666408, 0.3694444444444444642, 0.3722222222222222321, 0.3750000000000000000, 0.3777777777777777679, 0.3805555555555555358, 0.3833333333333333592 ),
 .UNSPECIFIED. ) 
 CURVE ( )  GEOMETRIC_REPRESENTATION_ITEM ( )  RATIONAL_B_SPLINE_CURVE ( ( 1.000000000000000000, 0.9659258262890683122, 1.000000000000000000, 0.9659258262890683122, 1.000000000000000000, 0.9659258262890683122, 1.000000000000000000, 0.9659258262890683122, 1.000000000000000000, 0.9659258262890683122, 1.000000000000000000, 0.9659258262890683122, 1.000000000000000000 ) ) 
 REPRESENTATION_ITEM ( '' )  );
#111410=CARTESIAN_POINT ( 'NONE',  ( 6.401278309935243271, 9.300261028980425948, -1.956595482711489531 ) ) ;
#111426=CARTESIAN_POINT ( 'NONE',  ( 41.39583333333331439, -2.130196079827427091, 7.949999999999998401 ) ) ;
#111440=EDGE_CURVE ( 'NONE', #69673, #63944, #38415, .T. ) ;
#111441=CARTESIAN_POINT ( 'NONE',  ( 115.4333603837961988, 2.130196079827431532, -7.949999999999997513 ) ) ;
#111458=CARTESIAN_POINT ( 'NONE',  ( 89.83376352523143282, 6.110000000000001208, 1.122388791418549305E-15 ) ) ;
#111485=CARTESIAN_POINT ( 'NONE',  ( 88.37543019189811844, -5.291415217122920289, -3.055000000000001492 ) ) ;
#111498=CARTESIAN_POINT ( 'NONE',  ( 87.12043019189812298, 3.055000000000001936, -5.291415217122916737 ) ) ;
#111513=DIRECTION ( 'NONE',  ( 0.000000000000000000, 0.000000000000000000, -1.000000000000000000 ) ) ;
#111528=DIRECTION ( 'NONE',  ( -1.000000000000000000, -0.000000000000000000, -0.000000000000000000 ) ) ;
#111548=CARTESIAN_POINT ( 'NONE',  ( 116.3754301918981042, -5.291415217122920289, -3.055000000000001492 ) ) ;
#111549=CARTESIAN_POINT ( 'NONE',  ( 0.000000000000000000, 0.000000000000000000, 0.000000000000000000 ) ) ;
#111570=PLANE ( 'NONE',  #74612 ) ;
#111583=CARTESIAN_POINT ( 'NONE',  ( 83.76626352523145158, 4.472830434245839371, -4.472830434245839371 ) ) ;
#111643=CARTESIAN_POINT ( 'NONE',  ( 105.8541666666666430, -2.130196079827425315, -7.950000000000001066 ) ) ;
#111663=CARTESIAN_POINT ( 'NONE',  ( 27.00000000000000000, 5.807595119381032234, 2.946028100216067092 ) ) ;
#111672=CARTESIAN_POINT ( 'NONE',  ( 124.5420968585647756, 5.291415217122923842, -3.054999999999996163 ) ) ;
#111675=CARTESIAN_POINT ( 'NONE',  ( 100.0208333333333286, 7.949999999999998401, 2.130196079827431532 ) ) ;
#111680=CARTESIAN_POINT ( 'NONE',  ( 116.2870968585647802, 3.054999999999997495, 5.291415217122919401 ) ) ;
#111689=CARTESIAN_POINT ( 'NONE',  ( 40.97959685856477563, 6.109999999999999432, 1.637169565754164280 ) ) ;
#111693=CARTESIAN_POINT ( 'NONE',  ( 30.97459685856477662, 1.637169565754164058, -6.109999999999996767 ) ) ;
#111703=VECTOR ( 'NONE', #88556, 1000.000000000000000 ) ;
#111728=ADVANCED_FACE ( 'NONE', ( #43409 ), #65184, .T. ) ;
#111729=CARTESIAN_POINT ( 'NONE',  ( 49.78709685856478018, 3.054999999999997495, 5.291415217122919401 ) ) ;
#111736=DIRECTION ( 'NONE',  ( -1.000000000000000000, -0.000000000000000000, -0.000000000000000000 ) ) ;
#111752=CARTESIAN_POINT ( 'NONE',  ( 36.10002705046289151, 5.819803920172570422, 5.819803920172575751 ) ) ;
#111764=CARTESIAN_POINT ( 'NONE',  ( 110.1620968585647944, -5.291415217122919401, 3.054999999999998384 ) ) ;
#111806=CARTESIAN_POINT ( 'NONE',  ( 30.97459685856477662, 1.637169565754164280, -6.109999999999997655 ) ) ;
#111826=CARTESIAN_POINT ( 'NONE',  ( 0.000000000000000000, 0.000000000000000000, 0.000000000000000000 ) ) ;
#111829=CARTESIAN_POINT ( 'NONE',  ( 124.3962635252314470, 4.472830434245840259, -4.472830434245839371 ) ) ;
#111840=CARTESIAN_POINT ( 'NONE',  ( 51.55836038379622011, -7.949999999999997513, -2.130196079827425759 ) ) ;
#111846=CARTESIAN_POINT ( 'NONE',  ( 41.39583333333331439, -2.130196079827427091, 7.949999999999999289 ) ) ;
#111854=CARTESIAN_POINT ( 'NONE',  ( 42.14626352523143282, -4.472830434245840259, 4.472830434245839371 ) ) ;
#111876=CARTESIAN_POINT ( 'NONE',  ( 57.22459685856476597, -1.637169565754160949, 6.109999999999997655 ) ) ;
#111905=EDGE_CURVE ( 'NONE', #4663, #113019, #13990, .T. ) ;
#111907=CARTESIAN_POINT ( 'NONE',  ( 75.01626352523142316, -4.472830434245838482, 4.472830434245838482 ) ) ;
#111941=CARTESIAN_POINT ( 'NONE',  ( 89.03752705046288440, -9.735942053221456900E-16, 7.949999999999998401 ) ) ;
#111992=CARTESIAN_POINT ( 'NONE',  ( 52.41209685856478018, 5.291415217122922066, -3.054999999999995275 ) ) ;
#111993=FACE_OUTER_BOUND ( 'NONE', #10375, .T. ) ;
#112015=CARTESIAN_POINT ( 'NONE',  ( 76.64169371712954160, -2.130196079827424871, -7.949999999999999289 ) ) ;
#112020=CARTESIAN_POINT ( 'NONE',  ( 76.97916666666665719, -7.950000000000001066, 2.130196079827424427 ) ) ;
#112030=CARTESIAN_POINT ( 'NONE',  ( 67.52126352523141861, -4.472830434245839371, -4.472830434245840259 ) ) ;
#112035=CARTESIAN_POINT ( 'NONE',  ( 44.60416666666665719, 2.130196079827422206, 7.950000000000001954 ) ) ;
#112046=CARTESIAN_POINT ( 'NONE',  ( 57.02126352523143993, -4.472830434245839371, -4.472830434245840259 ) ) ;
#112063=CARTESIAN_POINT ( 'NONE',  ( 112.0791937171295558, 3.975000000000002753, -6.884901960086283523 ) ) ;
#112071=DIRECTION ( 'NONE',  ( 0.000000000000000000, 0.000000000000000000, 1.000000000000000000 ) ) ;
#112079=CARTESIAN_POINT ( 'NONE',  ( 104.1829301918981088, -1.637169565754158951, -6.109999999999998543 ) ) ;
#112097=CARTESIAN_POINT ( 'NONE',  ( 67.93750000000000000, 5.819803920172574863, -5.819803920172573086 ) ) ;
#112110=CARTESIAN_POINT ( 'NONE',  ( 55.70876352523143282, -7.482591942790329030E-16, 6.110000000000001208 ) ) ;
#112115=CARTESIAN_POINT ( 'NONE',  ( 89.54209685856477563, 5.291415217122923842, -3.054999999999996163 ) ) ;
#112156=CARTESIAN_POINT ( 'NONE',  ( 5.950172325297302223, 9.499920639676602718, 0.2930115638150264101 ) ) ;
#112182=CARTESIAN_POINT ( 'NONE',  ( 101.2875270504628986, 0.000000000000000000, -7.949999999999998401 ) ) ;
#112199=CARTESIAN_POINT ( 'NONE',  ( 93.47959685856474721, 6.109999999999999432, 1.637169565754164280 ) ) ;
#112220=CARTESIAN_POINT ( 'NONE',  ( 79.33376352523144703, 6.110000000000001208, 1.122388791418549305E-15 ) ) ;
#112232=CARTESIAN_POINT ( 'NONE',  ( 83.62043019189812298, 3.055000000000001936, -5.291415217122916737 ) ) ;
#112274=ORIENTED_EDGE ( 'NONE', *, *, #105216, .F. ) ;
#112284=CARTESIAN_POINT ( 'NONE',  ( 114.0420968585647898, 5.291415217122923842, -3.054999999999996163 ) ) ;
#112298=ADVANCED_FACE ( 'NONE', ( #114874 ), #17031, .T. ) ;
#112302=CARTESIAN_POINT ( 'NONE',  ( 107.4125270504628986, -7.949999999999998401, -4.867971026610728450E-16 ) ) ;
#112314=CARTESIAN_POINT ( 'NONE',  ( 80.84959685856478018, 6.109999999999997655, 1.637169565754163836 ) ) ;
#112316=CARTESIAN_POINT ( 'NONE',  ( 98.66252705046289861, 7.949999999999998401, 1.460391307983218338E-15 ) ) ;
#112319=VERTEX_POINT ( 'NONE', #129344 ) ;
#112358=CARTESIAN_POINT ( 'NONE',  ( 92.29166666666665719, 3.975000000000003642, -6.884901960086285300 ) ) ;
#112387=CARTESIAN_POINT ( 'NONE',  ( 122.5004301918981184, -3.055000000000002380, 5.291415217122920289 ) ) ;
#112396=CARTESIAN_POINT ( 'NONE',  ( 114.0995968585647660, -6.109999999999997655, -1.637169565754160283 ) ) ;
#112399=EDGE_CURVE ( 'NONE', #113019, #8484, #43656, .T. ) ;
#112408=CARTESIAN_POINT ( 'NONE',  ( 30.24543019189811233, -5.291415217122918513, -3.055000000000000160 ) ) ;
#112440=CARTESIAN_POINT ( 'NONE',  ( 46.14126352523144448, 4.472830434245835818, 4.472830434245840259 ) ) ;
#112470=EDGE_CURVE ( 'NONE', #33848, #135001, #140782, .T. ) ;
#112475=CARTESIAN_POINT ( 'NONE',  ( 106.2245968585647802, -1.637169565754161171, 6.109999999999998543 ) ) ;
#112529=CARTESIAN_POINT ( 'NONE',  ( 120.4587635252314328, 0.000000000000000000, -6.110000000000001208 ) ) ;
#112533=CARTESIAN_POINT ( 'NONE',  ( 106.2458603837962272, 3.974999999999996980, 6.884901960086287964 ) ) ;
#112540=CARTESIAN_POINT ( 'NONE',  ( 51.12086038379622011, -6.884901960086286188, 3.974999999999997424 ) ) ;
#112547=CARTESIAN_POINT ( 'NONE',  ( 46.06249999999999289, -5.819803920172572198, -5.819803920172573086 ) ) ;
#112556=CARTESIAN_POINT ( 'NONE',  ( 39.81293019189809712, -1.637169565754159617, -6.110000000000001208 ) ) ;
#112574=DIRECTION ( 'NONE',  ( -1.000000000000000000, -0.000000000000000000, -0.000000000000000000 ) ) ;
#112581=CARTESIAN_POINT ( 'NONE',  ( 60.57876352523145158, -7.482591942790325086E-16, 6.109999999999998543 ) ) ;
#112610=CARTESIAN_POINT ( 'NONE',  ( 77.34959685856478018, 6.109999999999996767, 1.637169565754163836 ) ) ;
#112633=CARTESIAN_POINT ( 'NONE',  ( 29.75043019189810423, 3.055000000000002824, -5.291415217122919401 ) ) ;
#112667=CARTESIAN_POINT ( 'NONE',  ( 25.31559147121573972, -5.499261314031187453, -3.175000000000002487 ) ) ;
#112680=CARTESIAN_POINT ( 'NONE',  ( 52.12043019189811588, 3.055000000000002380, -5.291415217122917625 ) ) ;
#112695=DIRECTION ( 'NONE',  ( -1.000000000000000000, -0.000000000000000000, -0.000000000000000000 ) ) ;
#112707=CARTESIAN_POINT ( 'NONE',  ( 72.70419371712955581, -6.884901960086285300, -3.975000000000000089 ) ) ;
#112713=CARTESIAN_POINT ( 'NONE',  ( 70.27083333333334281, -7.949999999999999289, -2.130196079827426203 ) ) ;
#112723=CARTESIAN_POINT ( 'NONE',  ( 70.00043019189810423, -3.055000000000002380, 5.291415217122920289 ) ) ;
#112742=CARTESIAN_POINT ( 'NONE',  ( 56.58376352523143993, -6.110000000000001208, -3.741295971395164515E-16 ) ) ;
#112765=CARTESIAN_POINT ( 'NONE',  ( 36.82919371712956291, -3.975000000000001865, 6.884901960086284411 ) ) ;
#112773=CARTESIAN_POINT ( 'NONE',  ( 104.6204301918981230, 3.055000000000001936, -5.291415217122916737 ) ) ;
#112786=CARTESIAN_POINT ( 'NONE',  ( 27.35002705046288085, -5.819803920172573086, -5.819803920172573086 ) ) ;
#112795=CARTESIAN_POINT ( 'NONE',  ( 50.89626352523143993, 4.472830434245840259, -4.472830434245838482 ) ) ;
#112801=CARTESIAN_POINT ( 'NONE',  ( 94.50043019189810423, -3.055000000000002380, 5.291415217122920289 ) ) ;
#112814=CARTESIAN_POINT ( 'NONE',  ( 126.2037635252314658, 6.109999999999999432, 1.122388791418549108E-15 ) ) ;
#112819=ORIENTED_EDGE ( 'NONE', *, *, #59783, .T. ) ;
#112848=EDGE_CURVE ( 'NONE', #112319, #67893, #138083, .T. ) ;
#112871=CARTESIAN_POINT ( 'NONE',  ( 105.0791937171295700, 3.975000000000002753, -6.884901960086283523 ) ) ;
#112888=ADVANCED_FACE ( 'NONE', ( #125068 ), #67887, .T. ) ;
#112890=CARTESIAN_POINT ( 'NONE',  ( 96.39626352523144703, 4.472830434245840259, -4.472830434245839371 ) ) ;
#112897=EDGE_CURVE ( 'NONE', #121255, #143282, #88122, .T. ) ;
#112915=CARTESIAN_POINT ( 'NONE',  ( 87.50043019189810423, -3.055000000000002380, 5.291415217122920289 ) ) ;
#112925=CARTESIAN_POINT ( 'NONE',  ( 81.28709685856478018, 3.054999999999997495, 5.291415217122919401 ) ) ;
#112975=CARTESIAN_POINT ( 'NONE',  ( 117.9795968585647756, 6.109999999999999432, 1.637169565754164280 ) ) ;
#113019=VERTEX_POINT ( 'NONE', #140076 ) ;
#113039=CARTESIAN_POINT ( 'NONE',  ( 0.000000000000000000, 0.000000000000000000, 0.000000000000000000 ) ) ;
#113045=CARTESIAN_POINT ( 'NONE',  ( 93.45833333333334281, 3.974999999999997424, 6.884901960086288852 ) ) ;
#113052=CARTESIAN_POINT ( 'NONE',  ( 10.91209335768108168, 8.448398485916262857, 4.344958105531096848 ) ) ;
#113077=CARTESIAN_POINT ( 'NONE',  ( 108.3545968585647472, -1.637169565754161615, 6.110000000000000320 ) ) ;
#113086=CARTESIAN_POINT ( 'NONE',  ( 109.8704301918981230, -3.055000000000001492, 5.291415217122917625 ) ) ;
#113102=CARTESIAN_POINT ( 'NONE',  ( 27.47459685856478018, 1.637169565754164058, -6.109999999999996767 ) ) ;
#113113=CARTESIAN_POINT ( 'NONE',  ( 78.53752705046289861, -9.735942053221456900E-16, 7.949999999999998401 ) ) ;
#113121=CARTESIAN_POINT ( 'NONE',  ( 64.53752705046289861, -9.735942053221456900E-16, 7.949999999999998401 ) ) ;
#113130=CARTESIAN_POINT ( 'NONE',  ( 38.41209685856478018, 5.291415217122921177, -3.054999999999994831 ) ) ;
#113165=CARTESIAN_POINT ( 'NONE',  ( 109.1412635252314374, 4.472830434245837594, 4.472830434245841147 ) ) ;
#113216=CARTESIAN_POINT ( 'NONE',  ( 121.4583333333333286, 3.974999999999997424, 6.884901960086288852 ) ) ;
#113228=CARTESIAN_POINT ( 'NONE',  ( 115.2087635252314470, -7.482591942790329030E-16, 6.110000000000001208 ) ) ;
#113238=CARTESIAN_POINT ( 'NONE',  ( 43.53752705046289151, -9.735942053221456900E-16, 7.949999999999998401 ) ) ;
#113243=CARTESIAN_POINT ( 'NONE',  ( 37.74999999999999289, -9.735942053221458872E-16, 7.950000000000000178 ) ) ;
#113251=CARTESIAN_POINT ( 'NONE',  ( 34.70876352523143282, -7.482591942790329030E-16, 6.110000000000001208 ) ) ;
#113277=CARTESIAN_POINT ( 'NONE',  ( 58.09959685856477307, -6.109999999999997655, -1.637169565754160283 ) ) ;
#113285=AXIS2_PLACEMENT_3D ( 'NONE', #59777, #103943, #4590 ) ;
#113303=ORIENTED_EDGE ( 'NONE', *, *, #99454, .T. ) ;
#113304=CARTESIAN_POINT ( 'NONE',  ( 68.89126352523143737, -4.472830434245838482, -4.472830434245838482 ) ) ;
#113311=CARTESIAN_POINT ( 'NONE',  ( 122.0416666666666714, -3.975000000000002753, 6.884901960086286188 ) ) ;
#113331=CARTESIAN_POINT ( 'NONE',  ( 42.37086038379622721, 6.884901960086289741, -3.974999999999993427 ) ) ;
#113379=CARTESIAN_POINT ( 'NONE',  ( 59.70376352523145158, 6.109999999999999432, 1.122388791418549108E-15 ) ) ;
#113385=ORIENTED_EDGE ( 'NONE', *, *, #59533, .T. ) ;
#113399=ORIENTED_EDGE ( 'NONE', *, *, #106068, .T. ) ;
#113408=CARTESIAN_POINT ( 'NONE',  ( 77.51669371712954160, 7.950000000000001066, -2.130196079827421318 ) ) ;
#113412=CARTESIAN_POINT ( 'NONE',  ( 76.39583333333332860, -2.130196079827427091, 7.949999999999999289 ) ) ;
#113422=CARTESIAN_POINT ( 'NONE',  ( 70.58376352523143282, -6.110000000000001208, -3.741295971395164515E-16 ) ) ;
#113441=CARTESIAN_POINT ( 'NONE',  ( 59.50043019189810423, -3.055000000000002380, 5.291415217122920289 ) ) ;
#113446=CARTESIAN_POINT ( 'NONE',  ( 111.3500270504628986, -5.819803920172573086, -5.819803920172573086 ) ) ;
#113447=CARTESIAN_POINT ( 'NONE',  ( 54.52083333333332149, 7.949999999999998401, 2.130196079827431532 ) ) ;
#113473=CARTESIAN_POINT ( 'NONE',  ( 105.3495968585647944, 6.109999999999996767, 1.637169565754163836 ) ) ;
#113479=LINE ( 'NONE', #124377, #101050 ) ;
#113500=CARTESIAN_POINT ( 'NONE',  ( 52.50043019189811133, -3.055000000000002380, 5.291415217122920289 ) ) ;
#113506=CARTESIAN_POINT ( 'NONE',  ( 87.93793019189809002, -6.110000000000001208, 1.637169565754158951 ) ) ;
#113547=CARTESIAN_POINT ( 'NONE',  ( 10.32500000000000107, 8.432637487761466488, 4.375000000000001776 ) ) ;
#113563=EDGE_CURVE ( 'NONE', #64622, #82404, #115505, .T. ) ;
#113567=VERTEX_POINT ( 'NONE', #11471 ) ;
#113576=CARTESIAN_POINT ( 'NONE',  ( 99.68336038379624142, -2.130196079827426203, 7.949999999999997513 ) ) ;
#113594=CARTESIAN_POINT ( 'NONE',  ( 98.58376352523144703, -6.110000000000001208, -3.741295971395164515E-16 ) ) ;
#113614=CYLINDRICAL_SURFACE ( 'NONE', #121092, 7.950000000000000178 ) ;
#113619=CARTESIAN_POINT ( 'NONE',  ( 86.47959685856477563, 6.109999999999999432, 1.637169565754164280 ) ) ;
#113632=CARTESIAN_POINT ( 'NONE',  ( 75.01626352523142316, -4.472830434245839371, 4.472830434245839371 ) ) ;
#113644=CARTESIAN_POINT ( 'NONE',  ( 20.65000000000000213, 9.500000000000000000, 0.000000000000000000 ) ) ;
#113684=ADVANCED_FACE ( 'NONE', ( #78208 ), #122390, .T. ) ;
#113689=CARTESIAN_POINT ( 'NONE',  ( 115.3545968585647614, -1.637169565754161615, 6.110000000000000320 ) ) ;
#113714=EDGE_CURVE ( 'NONE', #82607, #33848, #47746, .T. ) ;
#113776=CARTESIAN_POINT ( 'NONE',  ( 95.64583333333334281, 2.130196079827431976, -7.949999999999999289 ) ) ;
#113785=CARTESIAN_POINT ( 'NONE',  ( 14.25124240572947265, 9.301334755096696938, 1.951233148376585236 ) ) ;
#113791=CARTESIAN_POINT ( 'NONE',  ( 125.9517069660836484, 3.572642044305429643, -6.597326320955100520 ) ) ;
#113804=CARTESIAN_POINT ( 'NONE',  ( 106.6045968585647472, 1.637169565754164946, -6.109999999999999432 ) ) ;
#113813=CARTESIAN_POINT ( 'NONE',  ( 104.1829301918981088, -1.637169565754158951, -6.109999999999998543 ) ) ;
#113844=CARTESIAN_POINT ( 'NONE',  ( 63.95419371712955581, 6.884901960086283523, 3.975000000000002753 ) ) ;
#113854=CARTESIAN_POINT ( 'NONE',  ( 38.26626352523145158, 4.472830434245838482, -4.472830434245837594 ) ) ;
#113877=AXIS2_PLACEMENT_3D ( 'NONE', #57640, #22797, #21423 ) ;
#113895=CARTESIAN_POINT ( 'NONE',  ( 112.0579301918981372, 6.110000000000001208, -1.637169565754156286 ) ) ;
#113901=ORIENTED_EDGE ( 'NONE', *, *, #135782, .F. ) ;
#113943=CARTESIAN_POINT ( 'NONE',  ( 116.0625000000000000, -5.819803920172572198, -5.819803920172573086 ) ) ;
#113956=CARTESIAN_POINT ( 'NONE',  ( 109.6670968585647756, -3.055000000000000160, -5.291415217122921177 ) ) ;
#113968=CARTESIAN_POINT ( 'NONE',  ( 49.07919371712955581, 3.975000000000002753, -6.884901960086283523 ) ) ;
#113973=CARTESIAN_POINT ( 'NONE',  ( 34.54166666666666430, -3.975000000000002753, 6.884901960086286188 ) ) ;
#113986=CARTESIAN_POINT ( 'NONE',  ( 32.95876352523143282, 0.000000000000000000, -6.110000000000001208 ) ) ;
#113990=CARTESIAN_POINT ( 'NONE',  ( 1.500000000000000000, 1.163414459189985682E-15, -9.500000000000001776 ) ) ;
#113991=ORIENTED_EDGE ( 'NONE', *, *, #106117, .T. ) ;
#113997=CARTESIAN_POINT ( 'NONE',  ( 62.83333333333332149, -6.884901960086287964, 3.974999999999998312 ) ) ;
#114001=CARTESIAN_POINT ( 'NONE',  ( 39.16252705046288440, 7.949999999999998401, 1.460391307983218338E-15 ) ) ;
#114005=CARTESIAN_POINT ( 'NONE',  ( 54.16209685856478018, -5.291415217122919401, 3.054999999999997939 ) ) ;
#114031=CARTESIAN_POINT ( 'NONE',  ( 64.95376352523145158, -6.109999999999998543, -3.741295971395162543E-16 ) ) ;
#114035=VECTOR ( 'NONE', #105430, 1000.000000000000000 ) ;
#114051=EDGE_LOOP ( 'NONE', ( #11305, #50953, #18331, #11744 ) ) ;
#114053=EDGE_LOOP ( 'NONE', ( #59643, #108297, #119490, #101601 ) ) ;
#114071=ORIENTED_EDGE ( 'NONE', *, *, #46153, .F. ) ;
#114081=DIRECTION ( 'NONE',  ( -1.000000000000000000, -0.000000000000000000, -0.000000000000000000 ) ) ;
#114098=EDGE_CURVE ( 'NONE', #107625, #75066, #9304, .T. ) ;
#114103=CARTESIAN_POINT ( 'NONE',  ( 65.85002705046288440, -5.819803920172573086, -5.819803920172573086 ) ) ;
#114112=CARTESIAN_POINT ( 'NONE',  ( 60.28709685856478728, 3.054999999999997939, 5.291415217122920289 ) ) ;
#114134=CARTESIAN_POINT ( 'NONE',  ( 75.91252705046288440, -7.949999999999998401, -4.867971026610728450E-16 ) ) ;
#114135=CARTESIAN_POINT ( 'NONE',  ( 0.000000000000000000, 0.000000000000000000, -8.000000000000001776 ) ) ;
#114137=CARTESIAN_POINT ( 'NONE',  ( 66.77083333333332860, -7.949999999999999289, -2.130196079827426203 ) ) ;
#114147=CARTESIAN_POINT ( 'NONE',  ( 69.85459685856476142, -1.637169565754161615, 6.110000000000000320 ) ) ;
#114154=CARTESIAN_POINT ( 'NONE',  ( 44.16666666666665719, 6.884901960086285300, 3.975000000000003642 ) ) ;
#114198=CARTESIAN_POINT ( 'NONE',  ( 98.20376352523145158, 6.109999999999998543, 1.122388791418548911E-15 ) ) ;
#114227=CARTESIAN_POINT ( 'NONE',  ( 48.12543019189810423, 5.291415217122919401, 3.055000000000002824 ) ) ;
#114230=AXIS2_PLACEMENT_3D ( 'NONE', #70787, #93223, #59901 ) ;
#114300=CARTESIAN_POINT ( 'NONE',  ( 104.2041937171295700, -6.884901960086285300, -3.975000000000000089 ) ) ;
#114316=CARTESIAN_POINT ( 'NONE',  ( 91.14626352523144703, -4.472830434245840259, 4.472830434245839371 ) ) ;
#114325=CARTESIAN_POINT ( 'NONE',  ( 100.7500000000000000, -9.735942053221458872E-16, 7.950000000000000178 ) ) ;
#114340=ORIENTED_EDGE ( 'NONE', *, *, #77253, .F. ) ;
#114342=CARTESIAN_POINT ( 'NONE',  ( 82.39626352523143282, 4.472830434245840259, -4.472830434245839371 ) ) ;
#114355=CARTESIAN_POINT ( 'NONE',  ( 77.49543019189810877, 5.291415217122916737, 3.055000000000001936 ) ) ;
#114358=CARTESIAN_POINT ( 'NONE',  ( 34.64169371712954160, -2.130196079827424871, -7.949999999999998401 ) ) ;
#114396=ORIENTED_EDGE ( 'NONE', *, *, #52381, .F. ) ;
#114402=CARTESIAN_POINT ( 'NONE',  ( 50.53752705046289861, -9.735942053221456900E-16, 7.949999999999998401 ) ) ;
#114403=CARTESIAN_POINT ( 'NONE',  ( 115.0629301918981042, 1.637169565754157174, 6.110000000000002984 ) ) ;
#114433=CARTESIAN_POINT ( 'NONE',  ( 10.03498081871643954, -8.432637487761464712, 4.375000000000000888 ) ) ;
#114434=CARTESIAN_POINT ( 'NONE',  ( 14.25160702508294541, -9.301495327579425876, 1.950216952696393280 ) ) ;
#114449=CARTESIAN_POINT ( 'NONE',  ( 0.000000000000000000, 0.000000000000000000, 0.000000000000000000 ) ) ;
#114460=CARTESIAN_POINT ( 'NONE',  ( 32.43293019189810877, 1.637169565754156730, 6.110000000000001208 ) ) ;
#114462=CARTESIAN_POINT ( 'NONE',  ( 47.03752705046289151, -9.735942053221456900E-16, 7.949999999999998401 ) ) ;
#114474=CARTESIAN_POINT ( 'NONE',  ( 88.06249999999998579, -5.819803920172572198, -5.819803920172573086 ) ) ;
#114479=CARTESIAN_POINT ( 'NONE',  ( 13.79752787990784668, 9.118485449599289083, -2.676246828001755507 ) ) ;
#114484=CARTESIAN_POINT ( 'NONE',  ( 126.7260406512308322, 5.298822016825037728, 4.147063925414387953 ) ) ;
#114501=CARTESIAN_POINT ( 'NONE',  ( 114.0420968585647898, 5.291415217122923842, -3.054999999999996163 ) ) ;
#114514=CARTESIAN_POINT ( 'NONE',  ( 108.7037635252314516, 6.109999999999998543, 1.122388791418548911E-15 ) ) ;
#114529=( LENGTH_UNIT ( ) NAMED_UNIT ( * ) SI_UNIT ( .MILLI., .METRE. ) );
#114535=ORIENTED_EDGE ( 'NONE', *, *, #63406, .F. ) ;
#114560=CARTESIAN_POINT ( 'NONE',  ( 35.93293019189810877, 1.637169565754156508, 6.110000000000000320 ) ) ;
#114577=VERTEX_POINT ( 'NONE', #1672 ) ;
#114579=ORIENTED_EDGE ( 'NONE', *, *, #76128, .T. ) ;
#114592=CARTESIAN_POINT ( 'NONE',  ( 101.5579301918981088, 6.110000000000001208, -1.637169565754156286 ) ) ;
#114596=ORIENTED_EDGE ( 'NONE', *, *, #38464, .T. ) ;
#114636=CARTESIAN_POINT ( 'NONE',  ( 125.8183334000146374, -5.871789562033242760, 4.884347503592287865 ) ) ;
#114637=CARTESIAN_POINT ( 'NONE',  ( 29.10002705046288085, 5.819803920172570422, 5.819803920172575751 ) ) ;
#114642=CARTESIAN_POINT ( 'NONE',  ( 121.7500000000000000, -9.735942053221458872E-16, 7.950000000000000178 ) ) ;
#114652=CARTESIAN_POINT ( 'NONE',  ( 112.7295968585647756, -6.110000000000000320, -1.637169565754161393 ) ) ;
#114656=CARTESIAN_POINT ( 'NONE',  ( 105.5166937171295558, 7.950000000000000178, -2.130196079827421318 ) ) ;
#114658=CARTESIAN_POINT ( 'NONE',  ( 83.49586038379622721, -3.974999999999998312, -6.884901960086286188 ) ) ;
#114662=CARTESIAN_POINT ( 'NONE',  ( 39.16252705046288440, 7.949999999999998401, 1.460391307983218338E-15 ) ) ;
#114668=CARTESIAN_POINT ( 'NONE',  ( 34.68749999999999289, -5.819803920172573086, 5.819803920172572198 ) ) ;
#114677=CYLINDRICAL_SURFACE ( 'NONE', #41065, 7.950000000000000178 ) ;
#114680=CARTESIAN_POINT ( 'NONE',  ( 26.54209685856477563, 5.291415217122923842, -3.054999999999996163 ) ) ;
#114697=CARTESIAN_POINT ( 'NONE',  ( 52.41209685856478018, 5.291415217122921177, -3.054999999999994831 ) ) ;
#114706=CARTESIAN_POINT ( 'NONE',  ( 59.43336038379622011, 2.130196079827431532, -7.949999999999996625 ) ) ;
#114724=CARTESIAN_POINT ( 'NONE',  ( 64.37043019189810877, -3.055000000000001492, 5.291415217122917625 ) ) ;
#114735=CARTESIAN_POINT ( 'NONE',  ( 101.1874999999999858, -5.819803920172573974, 5.819803920172573086 ) ) ;
#114746=CARTESIAN_POINT ( 'NONE',  ( 30.31249999999999289, 5.819803920172571310, 5.819803920172576639 ) ) ;
#114748=CARTESIAN_POINT ( 'NONE',  ( 0.000000000000000000, 0.000000000000000000, 4.749999999999997335 ) ) ;
#114749=CARTESIAN_POINT ( 'NONE',  ( 41.93336038379621300, 2.130196079827431532, -7.949999999999996625 ) ) ;
#114754=CARTESIAN_POINT ( 'NONE',  ( 120.3916937171301953, 2.130196079819464128, 7.950000000004595613 ) ) ;
#114771=ORIENTED_EDGE ( 'NONE', *, *, #126459, .T. ) ;
#114785=CARTESIAN_POINT ( 'NONE',  ( 64.53752705046289861, -9.735942053221456900E-16, 7.949999999999998401 ) ) ;
#114793=CARTESIAN_POINT ( 'NONE',  ( 49.64126352523145158, 4.472830434245837594, 4.472830434245841147 ) ) ;
#114814=CARTESIAN_POINT ( 'NONE',  ( 67.45419371712955581, 6.884901960086283523, 3.975000000000002753 ) ) ;
#114817=CYLINDRICAL_SURFACE ( 'NONE', #113285, 7.950000000000000178 ) ;
#114820=CARTESIAN_POINT ( 'NONE',  ( 66.91666666666667140, -6.884901960086287076, -3.975000000000000977 ) ) ;
#114833=CARTESIAN_POINT ( 'NONE',  ( 60.37543019189810423, -5.291415217122920289, -3.055000000000001492 ) ) ;
#114844=CARTESIAN_POINT ( 'NONE',  ( 85.29166666666667140, 3.975000000000003642, -6.884901960086285300 ) ) ;
#114855=CARTESIAN_POINT ( 'NONE',  ( 124.3291937171295700, -3.975000000000001865, 6.884901960086284411 ) ) ;
#114874=FACE_OUTER_BOUND ( 'NONE', #65441, .T. ) ;
#114880=CARTESIAN_POINT ( 'NONE',  ( 93.82876352523145158, 0.000000000000000000, -6.109999999999998543 ) ) ;
#114888=DIRECTION ( 'NONE',  ( -1.000000000000000000, -0.000000000000000000, -0.000000000000000000 ) ) ;
#114904=CARTESIAN_POINT ( 'NONE',  ( 42.29209685856477563, -5.291415217122921177, 3.054999999999999272 ) ) ;
#114950=CARTESIAN_POINT ( 'NONE',  ( 70.93293019189810877, 1.637169565754156730, 6.110000000000001208 ) ) ;
#114953=DIRECTION ( 'NONE',  ( -1.000000000000000000, -0.000000000000000000, -0.000000000000000000 ) ) ;
#114975=CARTESIAN_POINT ( 'NONE',  ( 102.1625270504628844, 7.949999999999998401, 1.460391307983218338E-15 ) ) ;
#114994=CARTESIAN_POINT ( 'NONE',  ( 83.12543019189810423, 5.291415217122919401, 3.055000000000002824 ) ) ;
#115003=CARTESIAN_POINT ( 'NONE',  ( 117.4750270504628844, -5.819803920172573086, 5.819803920172573086 ) ) ;
#115018=CARTESIAN_POINT ( 'NONE',  ( 80.93793019189807580, -6.110000000000001208, 1.637169565754158951 ) ) ;
#115031=CARTESIAN_POINT ( 'NONE',  ( 79.68293019189812298, -1.637169565754158951, -6.109999999999998543 ) ) ;
#115057=CARTESIAN_POINT ( 'NONE',  ( 69.49586038379622721, -3.974999999999998312, -6.884901960086286188 ) ) ;
#115062=CARTESIAN_POINT ( 'NONE',  ( 0.000000000000000000, 7.776507174585690191E-16, -6.349999999999997868 ) ) ;
#115074=CARTESIAN_POINT ( 'NONE',  ( 74.81293019189809002, -1.637169565754159617, -6.110000000000001208 ) ) ;
#115079=CARTESIAN_POINT ( 'NONE',  ( 106.7504301918981184, 3.055000000000002824, -5.291415217122919401 ) ) ;
#115113=CARTESIAN_POINT ( 'NONE',  ( 13.61473099516978991, -9.049659518163096550, -2.897983823904738188 ) ) ;
#115146=CARTESIAN_POINT ( 'NONE',  ( 107.3124999999999858, 5.819803920172571310, 5.819803920172576639 ) ) ;
#115147=CARTESIAN_POINT ( 'NONE',  ( 27.18293019189811588, -1.637169565754159173, -6.109999999999999432 ) ) ;
#115164=CARTESIAN_POINT ( 'NONE',  ( 96.66666666666667140, 6.884901960086285300, 3.975000000000003642 ) ) ;
#115174=CARTESIAN_POINT ( 'NONE',  ( 126.3683832355216055, 7.029815251288743738, -0.9939000555549801774 ) ) ;
#115185=CARTESIAN_POINT ( 'NONE',  ( 115.6462635252314328, -4.472830434245840259, 4.472830434245839371 ) ) ;
#115195=CARTESIAN_POINT ( 'NONE',  ( 100.3912635252314516, -4.472830434245839371, -4.472830434245839371 ) ) ;
#115216=ORIENTED_EDGE ( 'NONE', *, *, #52818, .F. ) ;
#115238=CARTESIAN_POINT ( 'NONE',  ( 37.82876352523144448, 0.000000000000000000, -6.109999999999998543 ) ) ;
#115274=CARTESIAN_POINT ( 'NONE',  ( 104.1829301918981088, -1.637169565754159173, -6.109999999999999432 ) ) ;
#115297=AXIS2_PLACEMENT_3D ( 'NONE', #64829, #109011, #79313 ) ;
#115319=CARTESIAN_POINT ( 'NONE',  ( 26.62809147121574327, 6.350000000000004974, -1.701477371937626826 ) ) ;
#115326=CARTESIAN_POINT ( 'NONE',  ( 118.6874999999999858, -5.819803920172573086, 5.819803920172572198 ) ) ;
#115340=CARTESIAN_POINT ( 'NONE',  ( 108.3545968585647472, -1.637169565754161615, 6.110000000000000320 ) ) ;
#115345=CARTESIAN_POINT ( 'NONE',  ( 83.20419371712955581, -6.884901960086285300, -3.975000000000000089 ) ) ;
#115351=CARTESIAN_POINT ( 'NONE',  ( 37.55836038379622011, -7.949999999999997513, -2.130196079827425759 ) ) ;
#115356=CARTESIAN_POINT ( 'NONE',  ( 37.16666666666666430, 6.884901960086285300, 3.975000000000003642 ) ) ;
#115357=ORIENTED_EDGE ( 'NONE', *, *, #138994, .T. ) ;
#115368=CARTESIAN_POINT ( 'NONE',  ( 26.10459685856476852, 1.637169565754164946, -6.109999999999999432 ) ) ;
#115383=CARTESIAN_POINT ( 'NONE',  ( 53.14126352523144448, 4.472830434245836706, 4.472830434245840259 ) ) ;
#115417=CARTESIAN_POINT ( 'NONE',  ( 62.18293019189812298, -1.637169565754158951, -6.109999999999998543 ) ) ;
#115426=CARTESIAN_POINT ( 'NONE',  ( 101.9166666666666714, -6.884901960086287076, -3.975000000000000977 ) ) ;
#115491=CARTESIAN_POINT ( 'NONE',  ( 44.97459685856478018, 1.637169565754164280, -6.109999999999997655 ) ) ;
#115505=CIRCLE ( 'NONE', #80801, 6.349999999999999645 ) ;
#115518=CARTESIAN_POINT ( 'NONE',  ( 63.22502705046289151, 5.819803920172573086, -5.819803920172572198 ) ) ;
#115522=CARTESIAN_POINT ( 'NONE',  ( 60.64583333333333570, 2.130196079827431976, -7.949999999999999289 ) ) ;
#115530=CARTESIAN_POINT ( 'NONE',  ( 127.1072581378824253, -3.174999999999999378, -5.499261314031185677 ) ) ;
#115534=CARTESIAN_POINT ( 'NONE',  ( 59.64626352523142572, -4.472830434245840259, 4.472830434245839371 ) ) ;
#115581=CARTESIAN_POINT ( 'NONE',  ( 93.68293019189812298, -1.637169565754158951, -6.109999999999998543 ) ) ;
#115608=CARTESIAN_POINT ( 'NONE',  ( 46.52126352523142572, -4.472830434245838482, -4.472830434245840259 ) ) ;
#115629=DIRECTION ( 'NONE',  ( 0.000000000000000000, 0.000000000000000000, 1.000000000000000000 ) ) ;
#115648=CARTESIAN_POINT ( 'NONE',  ( 66.77083333333331439, -7.949999999999998401, -2.130196079827426203 ) ) ;
#115665=CARTESIAN_POINT ( 'NONE',  ( 75.89126352523143737, -4.472830434245839371, -4.472830434245839371 ) ) ;
#115666=CARTESIAN_POINT ( 'NONE',  ( 81.35416666666667140, -2.130196079827501698, -7.949999999999956657 ) ) ;
#115688=CARTESIAN_POINT ( 'NONE',  ( 96.32919371712955581, -3.975000000000001865, 6.884901960086284411 ) ) ;
#115689=CARTESIAN_POINT ( 'NONE',  ( 72.31250000000001421, 5.819803920172571310, 5.819803920172576639 ) ) ;
#115701=EDGE_CURVE ( 'NONE', #71447, #20610, #142730, .T. ) ;
#115702=CARTESIAN_POINT ( 'NONE',  ( 88.08376352523144703, -6.110000000000001208, -3.741295971395164515E-16 ) ) ;
#115713=CARTESIAN_POINT ( 'NONE',  ( 117.7666937171295416, -7.949999999999998401, 2.130196079827423983 ) ) ;
#115725=CARTESIAN_POINT ( 'NONE',  ( 70.29209685856477563, -5.291415217122921177, 3.054999999999999272 ) ) ;
#115747=CARTESIAN_POINT ( 'NONE',  ( 64.72916666666667140, 7.950000000000001954, -2.130196079827421762 ) ) ;
#115781=CARTESIAN_POINT ( 'NONE',  ( 70.43793019189810423, -6.110000000000001208, 1.637169565754158951 ) ) ;
#115789=CARTESIAN_POINT ( 'NONE',  ( 106.1670968585647756, -3.055000000000000160, -5.291415217122921177 ) ) ;
#115806=CARTESIAN_POINT ( 'NONE',  ( 114.8500270504628702, -5.819803920172573086, -5.819803920172573086 ) ) ;
#115814=CARTESIAN_POINT ( 'NONE',  ( 114.4583333333333286, 3.974999999999997424, 6.884901960086288852 ) ) ;
#115822=ORIENTED_EDGE ( 'NONE', *, *, #55548, .F. ) ;
#115860=ORIENTED_EDGE ( 'NONE', *, *, #48765, .T. ) ;
#115867=CARTESIAN_POINT ( 'NONE',  ( 120.9750270504629128, -5.819803920172572198, 5.819803920172572198 ) ) ;
#115882=CARTESIAN_POINT ( 'NONE',  ( 79.60416666666664298, 2.130196079827422206, 7.950000000000001954 ) ) ;
#115907=CARTESIAN_POINT ( 'NONE',  ( 113.4587635252314470, 0.000000000000000000, -6.110000000000001208 ) ) ;
#115917=CARTESIAN_POINT ( 'NONE',  ( 105.0579301918981230, 6.110000000000000320, -1.637169565754156064 ) ) ;
#115949=CARTESIAN_POINT ( 'NONE',  ( 112.3495968585647802, 6.109999999999996767, 1.637169565754163836 ) ) ;
#115975=CARTESIAN_POINT ( 'NONE',  ( 42.49543019189810877, 5.291415217122916737, 3.055000000000001936 ) ) ;
#116015=CARTESIAN_POINT ( 'NONE',  ( 104.6204301918981230, 3.055000000000002380, -5.291415217122917625 ) ) ;
#116075=CARTESIAN_POINT ( 'NONE',  ( 116.7916666666666714, 3.975000000000003642, -6.884901960086285300 ) ) ;
#116087=CARTESIAN_POINT ( 'NONE',  ( 116.0837635252314470, -6.110000000000001208, -3.741295971395164515E-16 ) ) ;
#116096=CARTESIAN_POINT ( 'NONE',  ( 33.47502705046289151, -5.819803920172572198, 5.819803920172572198 ) ) ;
#116101=CARTESIAN_POINT ( 'NONE',  ( 32.93749999999999289, 5.819803920172573974, -5.819803920172572198 ) ) ;
#116112=DIRECTION ( 'NONE',  ( 0.000000000000000000, 0.000000000000000000, 1.000000000000000000 ) ) ;
#116114=CARTESIAN_POINT ( 'NONE',  ( 30.04209685856476497, 5.291415217122923842, -3.054999999999996163 ) ) ;
#116124=CARTESIAN_POINT ( 'NONE',  ( 62.39583333333332149, -2.130196079827427091, 7.949999999999998401 ) ) ;
#116126=CARTESIAN_POINT ( 'NONE',  ( 53.66709685856477563, -3.055000000000000160, -5.291415217122921177 ) ) ;
#116137=CARTESIAN_POINT ( 'NONE',  ( 46.43293019189811588, 1.637169565754156508, 6.110000000000000320 ) ) ;
#116145=VECTOR ( 'NONE', #49761, 1000.000000000000000 ) ;
#116147=VERTEX_POINT ( 'NONE', #67574 ) ;
#116167=MECHANICAL_DESIGN_GEOMETRIC_PRESENTATION_REPRESENTATION('',(#28219),#34853);
#116176=CARTESIAN_POINT ( 'NONE',  ( 67.14126352523145158, 4.472830434245835818, 4.472830434245840259 ) ) ;
#116204=CARTESIAN_POINT ( 'NONE',  ( 30.45833333333332504, 3.974999999999997424, 6.884901960086288852 ) ) ;
#116254=CARTESIAN_POINT ( 'NONE',  ( 42.78709685856478728, 3.054999999999997939, 5.291415217122920289 ) ) ;
#116277=CARTESIAN_POINT ( 'NONE',  ( 67.89169371712955581, 2.130196079827421762, 7.950000000000001066 ) ) ;
#116281=CARTESIAN_POINT ( 'NONE',  ( 68.81250000000000000, 5.819803920172571310, 5.819803920172575751 ) ) ;
#116288=CARTESIAN_POINT ( 'NONE',  ( 53.66709685856477563, -3.055000000000000160, -5.291415217122921177 ) ) ;
#116290=EDGE_CURVE ( 'NONE', #61826, #75931, #40638, .T. ) ;
#116302=CARTESIAN_POINT ( 'NONE',  ( 100.2666937171295700, -7.949999999999998401, 2.130196079827423983 ) ) ;
#116318=CARTESIAN_POINT ( 'NONE',  ( 110.1833603837962130, -2.130196079827426203, 7.949999999999996625 ) ) ;
#116319=CARTESIAN_POINT ( 'NONE',  ( 72.55836038379622721, -7.949999999999996625, -2.130196079827426203 ) ) ;
#116330=CARTESIAN_POINT ( 'NONE',  ( 61.76669371712955581, -7.949999999999998401, 2.130196079827423983 ) ) ;
#116345=CARTESIAN_POINT ( 'NONE',  ( 98.64126352523145158, 4.472830434245835818, 4.472830434245840259 ) ) ;
#116375=CARTESIAN_POINT ( 'NONE',  ( 47.39626352523143282, 4.472830434245840259, -4.472830434245838482 ) ) ;
#116428=CARTESIAN_POINT ( 'NONE',  ( 73.12043019189812298, 3.055000000000002380, -5.291415217122917625 ) ) ;
#116429=EDGE_CURVE ( 'NONE', #139700, #64622, #23543, .T. ) ;
#116451=CARTESIAN_POINT ( 'NONE',  ( 97.78752705046289861, 0.000000000000000000, -7.949999999999998401 ) ) ;
#116454=LINE ( 'NONE', #17145, #35323 ) ;
#116463=CARTESIAN_POINT ( 'NONE',  ( 47.03752705046289151, -9.735942053221456900E-16, 7.949999999999998401 ) ) ;
#116465=CARTESIAN_POINT ( 'NONE',  ( 82.10459685856476142, 1.637169565754164946, -6.109999999999999432 ) ) ;
#116485=CARTESIAN_POINT ( 'NONE',  ( 71.02126352523144703, -4.472830434245839371, -4.472830434245840259 ) ) ;
#116544=CARTESIAN_POINT ( 'NONE',  ( 72.77126352523144703, 4.472830434245838482, 4.472830434245842035 ) ) ;
#116550=CARTESIAN_POINT ( 'NONE',  ( 111.7087635252314470, -7.482591942790329030E-16, 6.110000000000001208 ) ) ;
#116557=CARTESIAN_POINT ( 'NONE',  ( 35.22502705046288440, 5.819803920172573974, -5.819803920172573086 ) ) ;
#116558=CARTESIAN_POINT ( 'NONE',  ( 78.53752705046289861, -9.735942053221456900E-16, 7.949999999999998401 ) ) ;
#116580=CARTESIAN_POINT ( 'NONE',  ( 10.90898527456939426, -8.448166216745459423, 4.345408460216290791 ) ) ;
#116593=TOROIDAL_SURFACE ( 'NONE', #70392, 8.000000000000001776, 1.500000000000000000 ) ;
#116607=CARTESIAN_POINT ( 'NONE',  ( 104.9791666666666714, -7.950000000000000178, 2.130196079827424427 ) ) ;
#116613=CARTESIAN_POINT ( 'NONE',  ( 124.9125270504628986, -7.949999999999998401, -4.867971026610728450E-16 ) ) ;
#116629=CARTESIAN_POINT ( 'NONE',  ( 80.91666666666667140, -6.884901960086287076, -3.975000000000000977 ) ) ;
#116634=CARTESIAN_POINT ( 'NONE',  ( 29.82919371712955581, -3.975000000000001865, 6.884901960086284411 ) ) ;
#116650=CARTESIAN_POINT ( 'NONE',  ( 101.5004301918981042, -3.055000000000002380, 5.291415217122920289 ) ) ;
#116660=AXIS2_PLACEMENT_3D ( 'NONE', #105619, #93349, #92611 ) ;
#116661=CARTESIAN_POINT ( 'NONE',  ( 101.7037635252314374, 6.109999999999998543, 1.122388791418548911E-15 ) ) ;
#116688=CARTESIAN_POINT ( 'NONE',  ( 108.7037635252314516, 6.109999999999998543, 1.122388791418548911E-15 ) ) ;
#116716=CARTESIAN_POINT ( 'NONE',  ( 32.72459685856478018, -1.637169565754160949, 6.109999999999997655 ) ) ;
#116747=CARTESIAN_POINT ( 'NONE',  ( 101.4120968585647802, 5.291415217122922066, -3.054999999999995275 ) ) ;
#116796=CARTESIAN_POINT ( 'NONE',  ( 113.0000000000000000, 0.000000000000000000, -7.950000000000000178 ) ) ;
#116809=CARTESIAN_POINT ( 'NONE',  ( 101.6462635252314186, -4.472830434245840259, 4.472830434245839371 ) ) ;
#116819=CARTESIAN_POINT ( 'NONE',  ( 37.99586038379622011, -3.974999999999998312, -6.884901960086286188 ) ) ;
#116826=CARTESIAN_POINT ( 'NONE',  ( 28.12499999999999645, -7.950000000000000178, -4.867971026610729436E-16 ) ) ;
#116837=CARTESIAN_POINT ( 'NONE',  ( 30.91709685856476497, 3.054999999999998828, 5.291415217122922066 ) ) ;
#116845=CARTESIAN_POINT ( 'NONE',  ( 63.27083333333332860, -7.949999999999998401, -2.130196079827426203 ) ) ;
#116847=CARTESIAN_POINT ( 'NONE',  ( 56.87543019189809712, -5.291415217122920289, -3.055000000000001492 ) ) ;
#116857=CARTESIAN_POINT ( 'NONE',  ( 45.84959685856478018, 6.109999999999996767, 1.637169565754163836 ) ) ;
#116885=CARTESIAN_POINT ( 'NONE',  ( 53.72459685856478018, -1.637169565754160949, 6.109999999999997655 ) ) ;
#116908=CARTESIAN_POINT ( 'NONE',  ( 54.47502705046288440, -5.819803920172573086, 5.819803920172573086 ) ) ;
#116909=CARTESIAN_POINT ( 'NONE',  ( 30.02083333333332860, 7.949999999999998401, 2.130196079827431532 ) ) ;
#116960=CARTESIAN_POINT ( 'NONE',  ( 43.66209685856478728, -5.291415217122919401, 3.054999999999998384 ) ) ;
#116981=CARTESIAN_POINT ( 'NONE',  ( 64.10002705046287019, 5.819803920172570422, 5.819803920172574863 ) ) ;
#116986=CARTESIAN_POINT ( 'NONE',  ( 68.08333333333332860, 6.884901960086290629, -3.974999999999994316 ) ) ;
#116998=CARTESIAN_POINT ( 'NONE',  ( 60.52126352523143282, -4.472830434245839371, -4.472830434245840259 ) ) ;
#117049=CARTESIAN_POINT ( 'NONE',  ( 89.59959685856476597, -6.109999999999997655, -1.637169565754160283 ) ) ;
#117051=CARTESIAN_POINT ( 'NONE',  ( 49.99999999999998579, 0.000000000000000000, -7.950000000000000178 ) ) ;
#117066=CARTESIAN_POINT ( 'NONE',  ( 49.29209685856476852, -5.291415217122921177, 3.054999999999999272 ) ) ;
#117082=CYLINDRICAL_SURFACE ( 'NONE', #101726, 7.950000000000000178 ) ;
#117098=CARTESIAN_POINT ( 'NONE',  ( 66.33333333333332860, -6.884901960086287964, 3.974999999999998312 ) ) ;
#117113=EDGE_CURVE ( 'NONE', #2756, #55557, #18638, .T. ) ;
#117121=CARTESIAN_POINT ( 'NONE',  ( 79.09959685856478018, -6.109999999999998543, -1.637169565754160727 ) ) ;
#117126=DIRECTION ( 'NONE',  ( -1.000000000000000000, -0.000000000000000000, -0.000000000000000000 ) ) ;
#117142=CARTESIAN_POINT ( 'NONE',  ( 90.78752705046288440, 0.000000000000000000, -7.949999999999998401 ) ) ;
#117155=EDGE_LOOP ( 'NONE', ( #87416, #99004, #71248, #139687 ) ) ;
#117156=CARTESIAN_POINT ( 'NONE',  ( 80.79209685856477563, -5.291415217122921177, 3.054999999999999272 ) ) ;
#117173=CARTESIAN_POINT ( 'NONE',  ( 75.68793019189811844, 6.110000000000002984, -1.637169565754156730 ) ) ;
#117196=CARTESIAN_POINT ( 'NONE',  ( 52.43336038379622721, 2.130196079827431532, -7.949999999999996625 ) ) ;
#117225=CARTESIAN_POINT ( 'NONE',  ( 76.12543019189810423, 5.291415217122919401, 3.055000000000002824 ) ) ;
#117230=CARTESIAN_POINT ( 'NONE',  ( 109.9587635252314470, 0.000000000000000000, -6.110000000000001208 ) ) ;
#117263=CARTESIAN_POINT ( 'NONE',  ( 14.24942747710153412, -9.300561119015622324, -1.955118594580004254 ) ) ;
#117300=VECTOR ( 'NONE', #110943, 1000.000000000000000 ) ;
#117303=CARTESIAN_POINT ( 'NONE',  ( 122.1416937171295416, -2.130196079827424871, -7.949999999999999289 ) ) ;
#117317=CARTESIAN_POINT ( 'NONE',  ( 84.99999999999998579, 0.000000000000000000, -7.950000000000000178 ) ) ;
#117321=CARTESIAN_POINT ( 'NONE',  ( 91.95419371712957002, 6.884901960086283523, 3.975000000000002753 ) ) ;
#117340=CARTESIAN_POINT ( 'NONE',  ( 105.5837635252314328, -6.110000000000001208, -3.741295971395164515E-16 ) ) ;
#117349=CARTESIAN_POINT ( 'NONE',  ( 99.22459685856479439, -1.637169565754160949, 6.109999999999997655 ) ) ;
#117374=CARTESIAN_POINT ( 'NONE',  ( 153.6500000000000057, 7.776507174585690191E-16, -6.349999999999997868 ) ) ;
#117433=CARTESIAN_POINT ( 'NONE',  ( 94.41209685856478018, 5.291415217122922066, -3.054999999999995275 ) ) ;
#117475=CARTESIAN_POINT ( 'NONE',  ( 47.22916666666665719, 7.950000000000001954, -2.130196079827421762 ) ) ;
#117485=CARTESIAN_POINT ( 'NONE',  ( 111.3958333333333428, -2.130196079827427091, 7.949999999999999289 ) ) ;
#117499=CARTESIAN_POINT ( 'NONE',  ( 100.1879301918980900, 6.110000000000002984, -1.637169565754156730 ) ) ;
#117509=CARTESIAN_POINT ( 'NONE',  ( 40.03752705046288440, -9.735942053221456900E-16, 7.949999999999998401 ) ) ;
#117515=CARTESIAN_POINT ( 'NONE',  ( 125.7087635252314470, -7.482591942790329030E-16, 6.110000000000001208 ) ) ;
#117524=CARTESIAN_POINT ( 'NONE',  ( 124.5995968585647944, -6.109999999999997655, -1.637169565754160283 ) ) ;
#117534=CARTESIAN_POINT ( 'NONE',  ( 45.93793019189810423, -6.110000000000001208, 1.637169565754158951 ) ) ;
#117542=CARTESIAN_POINT ( 'NONE',  ( 48.62043019189811588, 3.055000000000001936, -5.291415217122916737 ) ) ;
#117564=CARTESIAN_POINT ( 'NONE',  ( 0.000000000000000000, 0.000000000000000000, 0.000000000000000000 ) ) ;
#117566=CARTESIAN_POINT ( 'NONE',  ( 52.55793019189810877, 6.110000000000000320, -1.637169565754156064 ) ) ;
#117642=CARTESIAN_POINT ( 'NONE',  ( 49.78709685856478018, 3.054999999999997939, 5.291415217122920289 ) ) ;
#117654=CARTESIAN_POINT ( 'NONE',  ( 82.52083333333331439, 7.949999999999998401, 2.130196079827431532 ) ) ;
#117665=CARTESIAN_POINT ( 'NONE',  ( 70.07919371712955581, 3.975000000000002753, -6.884901960086283523 ) ) ;
#117671=CARTESIAN_POINT ( 'NONE',  ( 56.12499999999999289, -7.950000000000000178, -4.867971026610729436E-16 ) ) ;
#117677=CARTESIAN_POINT ( 'NONE',  ( 43.31293019189810423, -1.637169565754159617, -6.110000000000001208 ) ) ;
#117703=CARTESIAN_POINT ( 'NONE',  ( 72.09959685856479439, -6.109999999999997655, -1.637169565754160283 ) ) ;
#117710=CARTESIAN_POINT ( 'NONE',  ( 75.03752705046288440, -9.735942053221456900E-16, 7.949999999999998401 ) ) ;
#117736=CARTESIAN_POINT ( 'NONE',  ( 84.93293019189812298, 1.637169565754156508, 6.110000000000000320 ) ) ;
#117759=CARTESIAN_POINT ( 'NONE',  ( 32.81293019189809002, -1.637169565754159617, -6.110000000000001208 ) ) ;
#117815=CARTESIAN_POINT ( 'NONE',  ( 71.51626352523145158, -4.472830434245839371, 4.472830434245839371 ) ) ;
#117821=CARTESIAN_POINT ( 'NONE',  ( 127.4587635252314470, 0.000000000000000000, -6.110000000000001208 ) ) ;
#117841=CARTESIAN_POINT ( 'NONE',  ( 95.30836038379619879, 7.949999999999997513, 2.130196079827431088 ) ) ;
#117853=CARTESIAN_POINT ( 'NONE',  ( 84.43793019189811844, -6.110000000000001208, 1.637169565754158951 ) ) ;
#117858=CARTESIAN_POINT ( 'NONE',  ( 117.6208603837962272, -6.884901960086286188, 3.974999999999997424 ) ) ;
#117867=CARTESIAN_POINT ( 'NONE',  ( 76.85459685856477563, -1.637169565754161615, 6.110000000000000320 ) ) ;
#117918=ORIENTED_EDGE ( 'NONE', *, *, #35510, .T. ) ;
#117928=CARTESIAN_POINT ( 'NONE',  ( 74.37543019189810423, -5.291415217122920289, -3.055000000000001492 ) ) ;
#117935=CARTESIAN_POINT ( 'NONE',  ( 113.1670968585647756, -3.055000000000000160, -5.291415217122921177 ) ) ;
#117977=CARTESIAN_POINT ( 'NONE',  ( 30.47959685856476852, 6.109999999999999432, 1.637169565754164280 ) ) ;
#117998=CARTESIAN_POINT ( 'NONE',  ( 125.4958603837962272, -3.974999999999998312, -6.884901960086286188 ) ) ;
#118013=CARTESIAN_POINT ( 'NONE',  ( 84.56250000000000000, -5.819803920172572198, -5.819803920172573086 ) ) ;
#118020=CARTESIAN_POINT ( 'NONE',  ( 30.55836038379622011, -7.949999999999996625, -2.130196079827426203 ) ) ;
#118041=CARTESIAN_POINT ( 'NONE',  ( 98.43793019189811844, -6.110000000000001208, 1.637169565754158951 ) ) ;
#118049=CARTESIAN_POINT ( 'NONE',  ( 98.49543019189812298, 5.291415217122916737, 3.055000000000001936 ) ) ;
#118055=VECTOR ( 'NONE', #102497, 1000.000000000000000 ) ;
#118071=ORIENTED_EDGE ( 'NONE', *, *, #64663, .T. ) ;
#118122=EDGE_CURVE ( 'NONE', #143282, #63944, #82616, .T. ) ;
#118144=CARTESIAN_POINT ( 'NONE',  ( 88.43293019189809456, 1.637169565754156730, 6.110000000000001208 ) ) ;
#118146=CARTESIAN_POINT ( 'NONE',  ( 0.000000000000000000, 0.000000000000000000, 7.950000000000000178 ) ) ;
#118198=CARTESIAN_POINT ( 'NONE',  ( 106.5833333333333286, 6.884901960086290629, -3.974999999999994316 ) ) ;
#118216=CARTESIAN_POINT ( 'NONE',  ( 102.8129301918981042, -1.637169565754159617, -6.110000000000001208 ) ) ;
#118225=CARTESIAN_POINT ( 'NONE',  ( 33.18336038379622721, -2.130196079827426203, 7.949999999999997513 ) ) ;
#118229=CARTESIAN_POINT ( 'NONE',  ( 31.18749999999998934, -5.819803920172573086, 5.819803920172572198 ) ) ;
#118241=CARTESIAN_POINT ( 'NONE',  ( 121.6829301918980946, -1.637169565754158951, -6.109999999999998543 ) ) ;
#118250=( LENGTH_UNIT ( ) NAMED_UNIT ( * ) SI_UNIT ( .MILLI., .METRE. ) );
#118253=CARTESIAN_POINT ( 'NONE',  ( 41.27126352523144703, 4.472830434245839371, 4.472830434245842035 ) ) ;
#118262=CARTESIAN_POINT ( 'NONE',  ( 41.47459685856477307, 1.637169565754164058, -6.109999999999996767 ) ) ;
#118274=CARTESIAN_POINT ( 'NONE',  ( 80.28752705046289861, 0.000000000000000000, -7.949999999999998401 ) ) ;
#118281=EDGE_CURVE ( 'NONE', #139751, #24590, #127045, .T. ) ;
#118296=CARTESIAN_POINT ( 'NONE',  ( 57.51626352523144448, -4.472830434245838482, 4.472830434245838482 ) ) ;
#118299=CYLINDRICAL_SURFACE ( 'NONE', #18577, 7.950000000000000178 ) ;
#118323=CARTESIAN_POINT ( 'NONE',  ( 54.03752705046288440, -9.735942053221456900E-16, 7.949999999999998401 ) ) ;
#118333=CARTESIAN_POINT ( 'NONE',  ( 121.6829301918980946, -1.637169565754159173, -6.109999999999999432 ) ) ;
#118340=CARTESIAN_POINT ( 'NONE',  ( 67.16252705046288440, 7.949999999999998401, 1.460391307983218338E-15 ) ) ;
#118343=FACE_OUTER_BOUND ( 'NONE', #117155, .T. ) ;
#118376=CARTESIAN_POINT ( 'NONE',  ( 35.34959685856478728, 6.109999999999997655, 1.637169565754163836 ) ) ;
#118400=CARTESIAN_POINT ( 'NONE',  ( 0.000000000000000000, 0.000000000000000000, 0.000000000000000000 ) ) ;
#118402=CARTESIAN_POINT ( 'NONE',  ( 59.43336038379622011, 2.130196079827431532, -7.949999999999997513 ) ) ;
#118406=CARTESIAN_POINT ( 'NONE',  ( 54.52083333333332149, 7.949999999999999289, 2.130196079827431532 ) ) ;
#118413=CARTESIAN_POINT ( 'NONE',  ( 127.3989248045490967, 0.000000000000000000, -6.349999999999997868 ) ) ;
#118416=CARTESIAN_POINT ( 'NONE',  ( 51.04209685856476852, 5.291415217122923842, -3.054999999999996163 ) ) ;
#118425=DIRECTION ( 'NONE',  ( 0.000000000000000000, 0.000000000000000000, 1.000000000000000000 ) ) ;
#118433=CARTESIAN_POINT ( 'NONE',  ( 127.0704994235588572, 0.7945742482428581610, 6.350000000000343370 ) ) ;
#118443=CARTESIAN_POINT ( 'NONE',  ( 70.34959685856478018, 6.109999999999996767, 1.637169565754163836 ) ) ;
#118456=DIRECTION ( 'NONE',  ( -1.000000000000000000, -0.000000000000000000, -0.000000000000000000 ) ) ;
#118477=CARTESIAN_POINT ( 'NONE',  ( 88.87043019189810877, -3.055000000000001492, 5.291415217122917625 ) ) ;
#118488=CYLINDRICAL_SURFACE ( 'NONE', #68150, 7.950000000000000178 ) ;
#118501=CARTESIAN_POINT ( 'NONE',  ( 40.25043019189809712, 3.055000000000002824, -5.291415217122919401 ) ) ;
#118524=CARTESIAN_POINT ( 'NONE',  ( 109.3083603837962130, 7.949999999999996625, 2.130196079827431088 ) ) ;
#118553=CARTESIAN_POINT ( 'NONE',  ( 64.22459685856478018, -1.637169565754161171, 6.109999999999998543 ) ) ;
#118582=CARTESIAN_POINT ( 'NONE',  ( 93.55836038379622721, -7.949999999999997513, -2.130196079827425759 ) ) ;
#118589=DIRECTION ( 'NONE',  ( 0.000000000000000000, 0.000000000000000000, 1.000000000000000000 ) ) ;
#118596=CARTESIAN_POINT ( 'NONE',  ( 78.16709685856476142, -3.055000000000000160, -5.291415217122921177 ) ) ;
#118603=( BOUNDED_CURVE ( )  B_SPLINE_CURVE ( 2, ( #123642, #112035, #134504, #24297, #114154, #80841, #58408, #91689, #77981, #100438, #91008, #25718, #1091 ),
 .UNSPECIFIED., .F., .T. ) 
 B_SPLINE_CURVE_WITH_KNOTS ( ( 3, 2, 2, 2, 2, 2, 3 ),
 ( 0.7833333333333333259, 0.7861111111111110938, 0.7888888888888888618, 0.7916666666666666297, 0.7944444444444443976, 0.7972222222222222765, 0.8000000000000000444 ),
 .UNSPECIFIED. ) 
 CURVE ( )  GEOMETRIC_REPRESENTATION_ITEM ( )  RATIONAL_B_SPLINE_CURVE ( ( 1.000000000000000000, 0.9659258262890683122, 1.000000000000000000, 0.9659258262890683122, 1.000000000000000000, 0.9659258262890683122, 1.000000000000000000, 0.9659258262890683122, 1.000000000000000000, 0.9659258262890683122, 1.000000000000000000, 0.9659258262890683122, 1.000000000000000000 ) ) 
 REPRESENTATION_ITEM ( '' )  );
#118611=CARTESIAN_POINT ( 'NONE',  ( 78.00000000000000000, 0.000000000000000000, -7.950000000000000178 ) ) ;
#118612=CARTESIAN_POINT ( 'NONE',  ( 60.06249999999998579, -5.819803920172573086, -5.819803920172573974 ) ) ;
#118615=CARTESIAN_POINT ( 'NONE',  ( 71.16709685856477563, -3.055000000000000160, -5.291415217122921177 ) ) ;
#118662=ORIENTED_EDGE ( 'NONE', *, *, #112848, .F. ) ;
#118666=CARTESIAN_POINT ( 'NONE',  ( 57.82919371712954870, -3.975000000000001865, 6.884901960086284411 ) ) ;
#118678=CARTESIAN_POINT ( 'NONE',  ( 60.66709685856477563, -3.055000000000000160, -5.291415217122921177 ) ) ;
#118685=CARTESIAN_POINT ( 'NONE',  ( 102.8129301918981042, -1.637169565754159617, -6.110000000000001208 ) ) ;
#118692=CARTESIAN_POINT ( 'NONE',  ( 91.12500000000000000, -7.950000000000000178, -4.867971026610729436E-16 ) ) ;
#118724=CARTESIAN_POINT ( 'NONE',  ( 25.52126352523142927, -4.472830434245839371, -4.472830434245840259 ) ) ;
#118731=CYLINDRICAL_SURFACE ( 'NONE', #133302, 7.950000000000000178 ) ;
#118745=CARTESIAN_POINT ( 'NONE',  ( 125.9333603837962414, 2.130196079827431532, -7.949999999999997513 ) ) ;
#118771=CARTESIAN_POINT ( 'NONE',  ( 93.16666666666667140, 6.884901960086285300, 3.975000000000003642 ) ) ;
#118776=CARTESIAN_POINT ( 'NONE',  ( 40.22916666666666430, 7.950000000000001954, -2.130196079827421762 ) ) ;
#118786=CARTESIAN_POINT ( 'NONE',  ( 105.7295968585647898, -6.110000000000000320, -1.637169565754161393 ) ) ;
#118788=ORIENTED_EDGE ( 'NONE', *, *, #106487, .F. ) ;
#118798=CARTESIAN_POINT ( 'NONE',  ( 92.37043019189810877, -3.055000000000001492, 5.291415217122917625 ) ) ;
#118851=CARTESIAN_POINT ( 'NONE',  ( 33.16209685856478018, -5.291415217122919401, 3.054999999999997939 ) ) ;
#118855=CARTESIAN_POINT ( 'NONE',  ( 125.8545968585647614, -1.637169565754161615, 6.110000000000000320 ) ) ;
#118885=CARTESIAN_POINT ( 'NONE',  ( 89.30793019189809456, -6.109999999999999432, 1.637169565754158507 ) ) ;
#118905=LINE ( 'NONE', #8672, #120366 ) ;
#118935=CARTESIAN_POINT ( 'NONE',  ( 108.6250000000000000, -7.950000000000000178, -4.867971026610729436E-16 ) ) ;
#118948=CARTESIAN_POINT ( 'NONE',  ( 105.2920968585647756, -5.291415217122921177, 3.054999999999999272 ) ) ;
#118961=CARTESIAN_POINT ( 'NONE',  ( 28.56249999999999289, -5.819803920172572198, -5.819803920172573086 ) ) ;
#118972=CARTESIAN_POINT ( 'NONE',  ( 119.7870968585647802, 3.054999999999997495, 5.291415217122919401 ) ) ;
#118979=CARTESIAN_POINT ( 'NONE',  ( 70.37086038379622721, 6.884901960086289741, -3.974999999999993427 ) ) ;
#118980=SURFACE_STYLE_USAGE ( .BOTH. , #40726 ) ;
#118986=CARTESIAN_POINT ( 'NONE',  ( 46.08376352523143993, -6.110000000000001208, -3.741295971395164515E-16 ) ) ;
#118994=CARTESIAN_POINT ( 'NONE',  ( 39.28709685856478018, 3.054999999999997495, 5.291415217122919401 ) ) ;
#119005=ORIENTED_EDGE ( 'NONE', *, *, #46585, .F. ) ;
#119021=CARTESIAN_POINT ( 'NONE',  ( 54.30793019189810877, -6.109999999999998543, 1.637169565754158507 ) ) ;
#119055=CARTESIAN_POINT ( 'NONE',  ( 119.7870968585647802, 3.054999999999997939, 5.291415217122920289 ) ) ;
#119063=CARTESIAN_POINT ( 'NONE',  ( 75.91252705046288440, -7.949999999999998401, -4.867971026610728450E-16 ) ) ;
#119084=DIRECTION ( 'NONE',  ( -1.000000000000000000, -0.000000000000000000, -0.000000000000000000 ) ) ;
#119097=CARTESIAN_POINT ( 'NONE',  ( 126.7587378609811282, -5.618906549250023197, -3.646044159374574711 ) ) ;
#119099=CARTESIAN_POINT ( 'NONE',  ( 35.05793019189811588, 6.110000000000001208, -1.637169565754156286 ) ) ;
#119125=CARTESIAN_POINT ( 'NONE',  ( 57.68336038379621300, -2.130196079827426203, 7.949999999999997513 ) ) ;
#119129=CARTESIAN_POINT ( 'NONE',  ( 51.02083333333332860, 7.949999999999999289, 2.130196079827431532 ) ) ;
#119135=CARTESIAN_POINT ( 'NONE',  ( 44.47959685856476852, 6.109999999999999432, 1.637169565754164280 ) ) ;
#119142=CARTESIAN_POINT ( 'NONE',  ( 81.60002705046291283, 5.819803920172570422, 5.819803920172575751 ) ) ;
#119149=CARTESIAN_POINT ( 'NONE',  ( 79.91709685856476142, 3.054999999999998828, 5.291415217122922066 ) ) ;
#119159=CARTESIAN_POINT ( 'NONE',  ( 65.24543019189810877, -5.291415217122918513, -3.055000000000000160 ) ) ;
#119162=ADVANCED_FACE ( 'NONE', ( #118343 ), #104866, .T. ) ;
#119172=CARTESIAN_POINT ( 'NONE',  ( 0.000000000000000000, 0.000000000000000000, 7.950000000000000178 ) ) ;
#119190=CARTESIAN_POINT ( 'NONE',  ( 89.30793019189810877, -6.109999999999998543, 1.637169565754158507 ) ) ;
#119207=CARTESIAN_POINT ( 'NONE',  ( 123.0166937171295416, 7.950000000000000178, -2.130196079827421318 ) ) ;
#119213=CARTESIAN_POINT ( 'NONE',  ( 34.70876352523143282, -7.482591942790329030E-16, 6.110000000000001208 ) ) ;
#119261=CARTESIAN_POINT ( 'NONE',  ( 63.64126352523144448, 4.472830434245837594, 4.472830434245841147 ) ) ;
#119277=CARTESIAN_POINT ( 'NONE',  ( 106.4374999999999858, 5.819803920172574863, -5.819803920172573086 ) ) ;
#119288=CARTESIAN_POINT ( 'NONE',  ( 88.74586038379622721, 3.974999999999996980, 6.884901960086287964 ) ) ;
#119301=CARTESIAN_POINT ( 'NONE',  ( 73.35459685856476142, -1.637169565754161615, 6.110000000000000320 ) ) ;
#119309=DIRECTION ( 'NONE',  ( -1.000000000000000000, -0.000000000000000000, -0.000000000000000000 ) ) ;
#119314=CARTESIAN_POINT ( 'NONE',  ( 76.25000000000000000, -9.735942053221458872E-16, 7.950000000000000178 ) ) ;
#119319=CARTESIAN_POINT ( 'NONE',  ( 65.47959685856477563, 6.109999999999999432, 1.637169565754164280 ) ) ;
#119322=CARTESIAN_POINT ( 'NONE',  ( 27.00000000000000355, 0.000000000000000000, 7.950000000000000178 ) ) ;
#119339=CARTESIAN_POINT ( 'NONE',  ( 61.95833333333332149, 3.974999999999997424, 6.884901960086288852 ) ) ;
#119344=CARTESIAN_POINT ( 'NONE',  ( 116.5787635252314516, -7.482591942790325086E-16, 6.109999999999998543 ) ) ;
#119345=EDGE_LOOP ( 'NONE', ( #50, #90299, #129546, #24624 ) ) ;
#119369=CARTESIAN_POINT ( 'NONE',  ( 61.10459685856476852, 1.637169565754164946, -6.109999999999999432 ) ) ;
#119376=CARTESIAN_POINT ( 'NONE',  ( 103.9795968585647756, 6.109999999999999432, 1.637169565754164280 ) ) ;
#119386=CARTESIAN_POINT ( 'NONE',  ( 76.78752705046289861, 0.000000000000000000, -7.949999999999998401 ) ) ;
#119392=CARTESIAN_POINT ( 'NONE',  ( 117.8912635252314516, -4.472830434245838482, -4.472830434245838482 ) ) ;
#119394=DIRECTION ( 'NONE',  ( 0.000000000000000000, 0.000000000000000000, 1.000000000000000000 ) ) ;
#119405=CARTESIAN_POINT ( 'NONE',  ( 38.33333333333332860, -6.884901960086287964, 3.974999999999998312 ) ) ;
#119418=CARTESIAN_POINT ( 'NONE',  ( 27.41709685856476142, 3.054999999999998828, 5.291415217122922066 ) ) ;
#119421=ORIENTED_EDGE ( 'NONE', *, *, #112848, .T. ) ;
#119438=CARTESIAN_POINT ( 'NONE',  ( 92.53752705046289861, -9.735942053221456900E-16, 7.949999999999998401 ) ) ;
#119440=CARTESIAN_POINT ( 'NONE',  ( 109.1625270504628986, 7.949999999999998401, 1.460391307983218338E-15 ) ) ;
#119480=CARTESIAN_POINT ( 'NONE',  ( 104.4170968585647756, 3.054999999999998828, 5.291415217122922066 ) ) ;
#119489=CARTESIAN_POINT ( 'NONE',  ( 99.37043019189812298, -3.055000000000001492, 5.291415217122917625 ) ) ;
#119490=ORIENTED_EDGE ( 'NONE', *, *, #91067, .F. ) ;
#119506=ORIENTED_EDGE ( 'NONE', *, *, #112897, .T. ) ;
#119535=CARTESIAN_POINT ( 'NONE',  ( 27.18293019189811588, -1.637169565754158951, -6.109999999999998543 ) ) ;
#119540=CARTESIAN_POINT ( 'NONE',  ( 127.4587635252314470, 0.000000000000000000, -6.110000000000001208 ) ) ;
#119575=CARTESIAN_POINT ( 'NONE',  ( 96.59959685856476597, -6.109999999999998543, -1.637169565754160727 ) ) ;
#119576=CARTESIAN_POINT ( 'NONE',  ( 7.656579674618784637, -8.841847278798848464, 3.478651043998596037 ) ) ;
#119603=LINE ( 'NONE', #20297, #109478 ) ;
#119616=CIRCLE ( 'NONE', #82610, 6.349999999999997868 ) ;
#119624=CARTESIAN_POINT ( 'NONE',  ( 112.1250000000000000, -7.950000000000000178, -4.867971026610729436E-16 ) ) ;
#119625=ORIENTED_EDGE ( 'NONE', *, *, #117113, .T. ) ;
#119636=CARTESIAN_POINT ( 'NONE',  ( 99.16709685856477563, -3.055000000000000160, -5.291415217122921177 ) ) ;
#119643=CARTESIAN_POINT ( 'NONE',  ( 27.64169371712955936, -2.130196079827424871, -7.949999999999999289 ) ) ;
#119649=CARTESIAN_POINT ( 'NONE',  ( 25.93749999999998224, 5.819803920172573974, -5.819803920172572198 ) ) ;
#119658=CARTESIAN_POINT ( 'NONE',  ( 123.2870968585647944, 3.054999999999997495, 5.291415217122919401 ) ) ;
#119667=CARTESIAN_POINT ( 'NONE',  ( 47.68793019189809712, 6.110000000000002984, -1.637169565754156730 ) ) ;
#119671=CARTESIAN_POINT ( 'NONE',  ( 108.2875270504628986, 0.000000000000000000, -7.949999999999998401 ) ) ;
#119674=CARTESIAN_POINT ( 'NONE',  ( 35.64126352523145158, 4.472830434245836706, 4.472830434245840259 ) ) ;
#119683=CARTESIAN_POINT ( 'NONE',  ( 79.41252705046289861, -7.949999999999998401, -4.867971026610728450E-16 ) ) ;
#119706=CARTESIAN_POINT ( 'NONE',  ( 54.01626352523144448, -4.472830434245838482, 4.472830434245838482 ) ) ;
#119743=CARTESIAN_POINT ( 'NONE',  ( 121.9745968585647802, 1.637169565754164280, -6.109999999999997655 ) ) ;
#119751=CARTESIAN_POINT ( 'NONE',  ( 66.72502705046288440, 5.819803920172573974, -5.819803920172573086 ) ) ;
#119788=CARTESIAN_POINT ( 'NONE',  ( 33.30793019189810877, -6.109999999999999432, 1.637169565754158507 ) ) ;
#119804=CARTESIAN_POINT ( 'NONE',  ( 127.4587635252314470, 0.000000000000000000, -6.110000000000001208 ) ) ;
#119814=CARTESIAN_POINT ( 'NONE',  ( 58.26669371712954870, -7.949999999999999289, 2.130196079827424427 ) ) ;
#119819=CARTESIAN_POINT ( 'NONE',  ( 51.89583333333332860, -2.130196079827427091, 7.949999999999999289 ) ) ;
#119828=CARTESIAN_POINT ( 'NONE',  ( 51.77126352523143993, 4.472830434245839371, 4.472830434245842035 ) ) ;
#119841=CARTESIAN_POINT ( 'NONE',  ( 80.79209685856477563, -5.291415217122921177, 3.054999999999999272 ) ) ;
#119848=CARTESIAN_POINT ( 'NONE',  ( 68.16209685856478018, -5.291415217122919401, 3.054999999999997939 ) ) ;
#119879=CARTESIAN_POINT ( 'NONE',  ( 80.84959685856478018, 6.109999999999996767, 1.637169565754163836 ) ) ;
#119888=DIRECTION ( 'NONE',  ( -1.000000000000000000, -0.000000000000000000, -0.000000000000000000 ) ) ;
#119904=CARTESIAN_POINT ( 'NONE',  ( 39.95876352523143282, 0.000000000000000000, -6.110000000000001208 ) ) ;
#119936=CARTESIAN_POINT ( 'NONE',  ( 97.05836038379621300, -7.949999999999996625, -2.130196079827426203 ) ) ;
#119951=CARTESIAN_POINT ( 'NONE',  ( 51.89583333333332860, -2.130196079827351596, 7.950000000000043698 ) ) ;
#119953=CARTESIAN_POINT ( 'NONE',  ( 62.32876352523145158, 0.000000000000000000, -6.109999999999999432 ) ) ;
#119970=CARTESIAN_POINT ( 'NONE',  ( 107.4583333333333428, 3.974999999999997424, 6.884901960086288852 ) ) ;
#119980=CARTESIAN_POINT ( 'NONE',  ( 85.53752705046288440, -9.735942053221456900E-16, 7.949999999999998401 ) ) ;
#119994=CARTESIAN_POINT ( 'NONE',  ( 72.33376352523143282, 6.110000000000001208, 1.122388791418549305E-15 ) ) ;
#119997=AXIS2_PLACEMENT_3D ( 'NONE', #113039, #22448, #134846 ) ;
#120011=( BOUNDED_CURVE ( )  B_SPLINE_CURVE ( 2, ( #45908, #90090, #135759, #69088, #34297, #134337, #114001, #92225, #135076, #35768, #91543, #13945, #102436 ),
 .UNSPECIFIED., .F., .T. ) 
 B_SPLINE_CURVE_WITH_KNOTS ( ( 3, 2, 2, 2, 2, 2, 3 ),
 ( 0.8499999999999999778, 0.8527777777777777457, 0.8555555555555555136, 0.8583333333333332815, 0.8611111111111111605, 0.8638888888888889284, 0.8666666666666666963 ),
 .UNSPECIFIED. ) 
 CURVE ( )  GEOMETRIC_REPRESENTATION_ITEM ( )  RATIONAL_B_SPLINE_CURVE ( ( 1.000000000000000000, 0.9659258262890683122, 1.000000000000000000, 0.9659258262890683122, 1.000000000000000000, 0.9659258262890683122, 1.000000000000000000, 0.9659258262890683122, 1.000000000000000000, 0.9659258262890683122, 1.000000000000000000, 0.9659258262890683122, 1.000000000000000000 ) ) 
 REPRESENTATION_ITEM ( '' )  );
#120014=CARTESIAN_POINT ( 'NONE',  ( 62.27126352523142572, 4.472830434245839371, 4.472830434245842035 ) ) ;
#120040=CARTESIAN_POINT ( 'NONE',  ( 112.4954301918981230, 5.291415217122916737, 3.055000000000001936 ) ) ;
#120051=CARTESIAN_POINT ( 'NONE',  ( 68.47502705046289861, -5.819803920172573086, 5.819803920172573086 ) ) ;
#120069=CARTESIAN_POINT ( 'NONE',  ( 59.35459685856476142, -1.637169565754161615, 6.110000000000000320 ) ) ;
#120076=CARTESIAN_POINT ( 'NONE',  ( 101.6462635252314328, -4.472830434245840259, 4.472830434245838482 ) ) ;
#120084=CARTESIAN_POINT ( 'NONE',  ( 90.54166666666665719, -3.975000000000002753, 6.884901960086286188 ) ) ;
#120093=CARTESIAN_POINT ( 'NONE',  ( 126.2037635252314658, 6.109999999999998543, 1.122388791418548911E-15 ) ) ;
#120106=EDGE_CURVE ( 'NONE', #20563, #98697, #40468, .T. ) ;
#120115=DIRECTION ( 'NONE',  ( -1.000000000000000000, -0.000000000000000000, -0.000000000000000000 ) ) ;
#120121=CARTESIAN_POINT ( 'NONE',  ( 27.27126352523142572, 4.472830434245839371, 4.472830434245842035 ) ) ;
#120125=ORIENTED_EDGE ( 'NONE', *, *, #122414, .F. ) ;
#120131=CARTESIAN_POINT ( 'NONE',  ( 43.00000000000000000, 0.000000000000000000, -7.950000000000000178 ) ) ;
#120141=CARTESIAN_POINT ( 'NONE',  ( 93.70419371712957002, -6.884901960086285300, -3.975000000000000089 ) ) ;
#120142=CARTESIAN_POINT ( 'NONE',  ( 115.5791937171295558, 3.975000000000002753, -6.884901960086283523 ) ) ;
#120174=CARTESIAN_POINT ( 'NONE',  ( 70.27083333333334281, -7.949999999999998401, -2.130196079827426203 ) ) ;
#120182=CARTESIAN_POINT ( 'NONE',  ( 96.83376352523144703, 6.110000000000001208, 1.122388791418549305E-15 ) ) ;
#120193=CARTESIAN_POINT ( 'NONE',  ( 89.16209685856478018, -5.291415217122919401, 3.054999999999997939 ) ) ;
#120196=CARTESIAN_POINT ( 'NONE',  ( 115.0416666666666714, -3.975000000000002753, 6.884901960086286188 ) ) ;
#120202=ORIENTED_EDGE ( 'NONE', *, *, #8080, .T. ) ;
#120211=VERTEX_POINT ( 'NONE', #32318 ) ;
#120242=CARTESIAN_POINT ( 'NONE',  ( 125.7087635252314470, -7.482591942790329030E-16, 6.110000000000001208 ) ) ;
#120271=ORIENTED_EDGE ( 'NONE', *, *, #71564, .T. ) ;
#120277=CARTESIAN_POINT ( 'NONE',  ( 92.51626352523146579, -4.472830434245839371, 4.472830434245839371 ) ) ;
#120278=CARTESIAN_POINT ( 'NONE',  ( 7.028598267277284428, -9.052066293035441191, -2.890594154426020967 ) ) ;
#120326=CARTESIAN_POINT ( 'NONE',  ( 104.9791666666666714, -7.950000000000001066, 2.130196079827424427 ) ) ;
#120331=CARTESIAN_POINT ( 'NONE',  ( 89.66666666666667140, 6.884901960086285300, 3.975000000000003642 ) ) ;
#120347=CARTESIAN_POINT ( 'NONE',  ( 29.24586038379621655, 3.974999999999996980, 6.884901960086287964 ) ) ;
#120351=CARTESIAN_POINT ( 'NONE',  ( 119.7295968585647614, -6.110000000000000320, -1.637169565754161393 ) ) ;
#120360=CARTESIAN_POINT ( 'NONE',  ( 125.9120968585647802, 5.291415217122921177, -3.054999999999994831 ) ) ;
#120366=VECTOR ( 'NONE', #18881, 1000.000000000000000 ) ;
#120371=CARTESIAN_POINT ( 'NONE',  ( 49.72959685856476852, -6.110000000000000320, -1.637169565754161393 ) ) ;
#120378=CARTESIAN_POINT ( 'NONE',  ( 40.16209685856478018, -5.291415217122919401, 3.054999999999997939 ) ) ;
#120410=CARTESIAN_POINT ( 'NONE',  ( 45.55793019189811588, 6.110000000000000320, -1.637169565754156064 ) ) ;
#120413=EDGE_CURVE ( 'NONE', #112319, #7244, #138046, .T. ) ;
#120447=CARTESIAN_POINT ( 'NONE',  ( 117.8912635252314516, -4.472830434245839371, -4.472830434245839371 ) ) ;
#120488=CARTESIAN_POINT ( 'NONE',  ( 39.57876352523144448, -7.482591942790327058E-16, 6.109999999999999432 ) ) ;
#120493=CARTESIAN_POINT ( 'NONE',  ( 126.4166666666666714, -6.884901960086287076, -3.975000000000000977 ) ) ;
#120520=CARTESIAN_POINT ( 'NONE',  ( 57.39169371712954870, 2.130196079827421762, 7.950000000000001066 ) ) ;
#120527=CARTESIAN_POINT ( 'NONE',  ( 55.54166666666665719, -3.975000000000002753, 6.884901960086286188 ) ) ;
#120536=CARTESIAN_POINT ( 'NONE',  ( 48.27126352523143993, 4.472830434245839371, 4.472830434245842035 ) ) ;
#120550=CARTESIAN_POINT ( 'NONE',  ( 78.89626352523143282, 4.472830434245840259, -4.472830434245838482 ) ) ;
#120560=CARTESIAN_POINT ( 'NONE',  ( 68.01626352523145158, -4.472830434245839371, 4.472830434245839371 ) ) ;
#120591=DIRECTION ( 'NONE',  ( -1.000000000000000000, -0.000000000000000000, -0.000000000000000000 ) ) ;
#120598=CARTESIAN_POINT ( 'NONE',  ( 86.53709685856478018, -3.054999999999998828, -5.291415217122919401 ) ) ;
#120627=CARTESIAN_POINT ( 'NONE',  ( 34.41709685856476852, 3.054999999999998828, 5.291415217122922066 ) ) ;
#120629=CARTESIAN_POINT ( 'NONE',  ( 45.33333333333332149, -6.884901960086287964, 3.974999999999998312 ) ) ;
#120652=EDGE_LOOP ( 'NONE', ( #2064, #67277, #63739, #32472 ) ) ;
#120659=PLANE ( 'NONE',  #51482 ) ;
#120681=CARTESIAN_POINT ( 'NONE',  ( 67.14126352523145158, 4.472830434245837594, 4.472830434245841147 ) ) ;
#120716=CARTESIAN_POINT ( 'NONE',  ( 89.18336038379621300, -2.130196079827426203, 7.949999999999997513 ) ) ;
#120721=EDGE_CURVE ( 'NONE', #82404, #1460, #58813, .T. ) ;
#120722=CARTESIAN_POINT ( 'NONE',  ( 83.39583333333334281, -2.130196079827427091, 7.949999999999999289 ) ) ;
#120735=CARTESIAN_POINT ( 'NONE',  ( 75.54209685856477563, 5.291415217122923842, -3.054999999999996163 ) ) ;
#120750=CARTESIAN_POINT ( 'NONE',  ( 77.85416666666667140, -2.130196079827425759, -7.950000000000000178 ) ) ;
#120755=CARTESIAN_POINT ( 'NONE',  ( 64.16709685856476142, -3.055000000000000160, -5.291415217122921177 ) ) ;
#120763=VECTOR ( 'NONE', #77755, 1000.000000000000000 ) ;
#120785=CARTESIAN_POINT ( 'NONE',  ( 115.5579301918981088, 6.110000000000000320, -1.637169565754156064 ) ) ;
#120796=VERTEX_POINT ( 'NONE', #71740 ) ;
#120797=CARTESIAN_POINT ( 'NONE',  ( 69.20419371712955581, -6.884901960086285300, -3.975000000000000089 ) ) ;
#120800=CARTESIAN_POINT ( 'NONE',  ( 58.99586038379622721, -3.974999999999998312, -6.884901960086286188 ) ) ;
#120813=CARTESIAN_POINT ( 'NONE',  ( 63.14626352523143282, -4.472830434245840259, 4.472830434245838482 ) ) ;
#120818=CARTESIAN_POINT ( 'NONE',  ( 99.16709685856477563, -3.055000000000000160, -5.291415217122921177 ) ) ;
#120835=CARTESIAN_POINT ( 'NONE',  ( 119.9329301918981088, 1.637169565754156508, 6.110000000000000320 ) ) ;
#120860=CARTESIAN_POINT ( 'NONE',  ( 28.29209685856476497, -5.291415217122921177, 3.054999999999999272 ) ) ;
#120871=CARTESIAN_POINT ( 'NONE',  ( 42.56249999999998579, -5.819803920172573086, -5.819803920172573974 ) ) ;
#120882=CARTESIAN_POINT ( 'NONE',  ( 112.8083603837962414, 7.949999999999997513, 2.130196079827431088 ) ) ;
#120902=VECTOR ( 'NONE', #110795, 1000.000000000000000 ) ;
#120905=EDGE_CURVE ( 'NONE', #69571, #32830, #131725, .T. ) ;
#120924=CARTESIAN_POINT ( 'NONE',  ( 70.85416666666669983, -2.130196079827501698, -7.949999999999956657 ) ) ;
#120931=CARTESIAN_POINT ( 'NONE',  ( 89.97959685856477563, 6.109999999999999432, 1.637169565754164280 ) ) ;
#120939=CARTESIAN_POINT ( 'NONE',  ( 86.39126352523146579, -4.472830434245839371, -4.472830434245839371 ) ) ;
#120990=CARTESIAN_POINT ( 'NONE',  ( 126.7295968585647756, -6.110000000000000320, -1.637169565754161393 ) ) ;
#121011=DIRECTION ( 'NONE',  ( -0.000000000000000000, 0.000000000000000000, 1.000000000000000000 ) ) ;
#121012=CARTESIAN_POINT ( 'NONE',  ( 107.2666937171295558, -7.949999999999998401, 2.130196079827423983 ) ) ;
#121014=EDGE_CURVE ( 'NONE', #20835, #133915, #17796, .T. ) ;
#121025=CARTESIAN_POINT ( 'NONE',  ( 84.20376352523145158, 6.109999999999999432, 1.122388791418549108E-15 ) ) ;
#121026=CARTESIAN_POINT ( 'NONE',  ( 7.649330195115605413, -8.844083433006840522, -3.472940883649443311 ) ) ;
#121039=AXIS2_PLACEMENT_3D ( 'NONE', #136163, #92639, #136878 ) ;
#121075=CARTESIAN_POINT ( 'NONE',  ( 103.8125000000000142, 5.819803920172571310, 5.819803920172575751 ) ) ;
#121092=AXIS2_PLACEMENT_3D ( 'NONE', #90448, #56445, #23008 ) ;
#121096=CARTESIAN_POINT ( 'NONE',  ( 30.41252705046289151, -7.949999999999998401, -4.867971026610728450E-16 ) ) ;
#121101=CARTESIAN_POINT ( 'NONE',  ( 117.9795968585647898, 6.109999999999999432, 1.637169565754164280 ) ) ;
#121102=ORIENTED_EDGE ( 'NONE', *, *, #27453, .T. ) ;
#121111=CARTESIAN_POINT ( 'NONE',  ( 112.3495968585647802, 6.109999999999996767, 1.637169565754163836 ) ) ;
#121121=CARTESIAN_POINT ( 'NONE',  ( 38.79209685856477563, -5.291415217122921177, 3.054999999999999272 ) ) ;
#121126=CARTESIAN_POINT ( 'NONE',  ( 36.95376352523144448, -6.109999999999998543, -3.741295971395162543E-16 ) ) ;
#121136=AXIS2_PLACEMENT_3D ( 'NONE', #35609, #13074, #126835 ) ;
#121151=ORIENTED_EDGE ( 'NONE', *, *, #135848, .T. ) ;
#121156=CARTESIAN_POINT ( 'NONE',  ( 47.59959685856477307, -6.109999999999997655, -1.637169565754160283 ) ) ;
#121165=AXIS2_PLACEMENT_3D ( 'NONE', #20882, #43375, #63010 ) ;
#121193=CARTESIAN_POINT ( 'NONE',  ( 115.9954301918981230, 5.291415217122917625, 3.055000000000002380 ) ) ;
#121234=CARTESIAN_POINT ( 'NONE',  ( 32.14126352523144448, 4.472830434245837594, 4.472830434245841147 ) ) ;
#121241=CARTESIAN_POINT ( 'NONE',  ( 125.6875000000000000, -5.819803920172573086, 5.819803920172572198 ) ) ;
#121251=DIRECTION ( 'NONE',  ( -1.000000000000000000, -0.000000000000000000, -0.000000000000000000 ) ) ;
#121254=CARTESIAN_POINT ( 'NONE',  ( 121.1879301918980900, 6.110000000000002984, -1.637169565754156730 ) ) ;
#121255=VERTEX_POINT ( 'NONE', #140367 ) ;
#121265=CARTESIAN_POINT ( 'NONE',  ( 52.72502705046289861, 5.819803920172573086, -5.819803920172572198 ) ) ;
#121272=CARTESIAN_POINT ( 'NONE',  ( 43.72916666666667140, 7.950000000000001954, -2.130196079827421762 ) ) ;
#121281=CARTESIAN_POINT ( 'NONE',  ( 34.85459685856477563, -1.637169565754161615, 6.110000000000000320 ) ) ;
#121296=CARTESIAN_POINT ( 'NONE',  ( 82.10459685856476142, 1.637169565754164946, -6.109999999999999432 ) ) ;
#121305=CARTESIAN_POINT ( 'NONE',  ( 63.34959685856478018, 6.109999999999996767, 1.637169565754163836 ) ) ;
#121323=CARTESIAN_POINT ( 'NONE',  ( 40.91252705046288440, -7.949999999999998401, -4.867971026610728450E-16 ) ) ;
#121332=CARTESIAN_POINT ( 'NONE',  ( 74.14126352523145158, 4.472830434245835818, 4.472830434245840259 ) ) ;
#121339=CARTESIAN_POINT ( 'NONE',  ( 122.7708333333333286, -7.949999999999998401, -2.130196079827426203 ) ) ;
#121367=DIRECTION ( 'NONE',  ( 0.000000000000000000, 0.000000000000000000, 1.000000000000000000 ) ) ;
#121408=CARTESIAN_POINT ( 'NONE',  ( 62.03709685856478728, -3.054999999999999272, -5.291415217122919401 ) ) ;
#121436=CARTESIAN_POINT ( 'NONE',  ( 86.26669371712955581, -7.949999999999999289, 2.130196079827424427 ) ) ;
#121441=CARTESIAN_POINT ( 'NONE',  ( 73.47916666666664298, -7.950000000000001066, 2.130196079827424427 ) ) ;
#121453=CARTESIAN_POINT ( 'NONE',  ( 71.31293019189810423, -1.637169565754159617, -6.110000000000001208 ) ) ;
#121469=CARTESIAN_POINT ( 'NONE',  ( 66.20876352523144703, -7.482591942790329030E-16, 6.110000000000001208 ) ) ;
#121483=ORIENTED_EDGE ( 'NONE', *, *, #112399, .T. ) ;
#121497=CARTESIAN_POINT ( 'NONE',  ( 107.5370968585647944, -3.054999999999998828, -5.291415217122919401 ) ) ;
#121507=CARTESIAN_POINT ( 'NONE',  ( 35.99999999999999289, 0.000000000000000000, -7.950000000000000178 ) ) ;
#121524=CARTESIAN_POINT ( 'NONE',  ( 56.43793019189809712, -6.110000000000001208, 1.637169565754158951 ) ) ;
#121531=CARTESIAN_POINT ( 'NONE',  ( 102.3754301918981184, -5.291415217122920289, -3.055000000000001492 ) ) ;
#121538=( BOUNDED_CURVE ( )  B_SPLINE_CURVE ( 2, ( #78008, #57699, #101878, #2544, #67878, #46851, #1805, #101161, #11270, #35948, #112063, #55540, #25020 ),
 .UNSPECIFIED., .F., .F. ) 
 B_SPLINE_CURVE_WITH_KNOTS ( ( 3, 2, 2, 2, 2, 2, 3 ),
 ( 0.1499999999999999944, 0.1527777777777777901, 0.1555555555555555580, 0.1583333333333333259, 0.1611111111111111216, 0.1638888888888888895, 0.1666666666666666574 ),
 .UNSPECIFIED. ) 
 CURVE ( )  GEOMETRIC_REPRESENTATION_ITEM ( )  RATIONAL_B_SPLINE_CURVE ( ( 1.000000000000000000, 0.9659258262890683122, 1.000000000000000000, 0.9659258262890683122, 1.000000000000000000, 0.9659258262890683122, 1.000000000000000000, 0.9659258262890683122, 1.000000000000000000, 0.9659258262890683122, 1.000000000000000000, 0.9659258262890683122, 1.000000000000000000 ) ) 
 REPRESENTATION_ITEM ( '' )  );
#121549=CARTESIAN_POINT ( 'NONE',  ( 123.5787635252314516, -7.482591942790325086E-16, 6.109999999999998543 ) ) ;
#121550=( BOUNDED_CURVE ( )  B_SPLINE_CURVE ( 2, ( #116558, #85336, #108491, #141909, #18641, #105653, #139770, #84651, #29527, #42601, #139034, #131018, #119386 ),
 .UNSPECIFIED., .F., .T. ) 
 B_SPLINE_CURVE_WITH_KNOTS ( ( 3, 2, 2, 2, 2, 2, 3 ),
 ( 0.4833333333333333370, 0.4861111111111111049, 0.4888888888888888729, 0.4916666666666666408, 0.4944444444444444642, 0.4972222222222222321, 0.5000000000000000000 ),
 .UNSPECIFIED. ) 
 CURVE ( )  GEOMETRIC_REPRESENTATION_ITEM ( )  RATIONAL_B_SPLINE_CURVE ( ( 1.000000000000000000, 0.9659258262890683122, 1.000000000000000000, 0.9659258262890683122, 1.000000000000000000, 0.9659258262890683122, 1.000000000000000000, 0.9659258262890683122, 1.000000000000000000, 0.9659258262890683122, 1.000000000000000000, 0.9659258262890683122, 1.000000000000000000 ) ) 
 REPRESENTATION_ITEM ( '' )  );
#121551=CARTESIAN_POINT ( 'NONE',  ( 10.32500000000000107, -9.500000000000001776, 0.000000000000000000 ) ) ;
#121572=ADVANCED_FACE ( 'NONE', ( #102597 ), #138066, .T. ) ;
#121596=CARTESIAN_POINT ( 'NONE',  ( 110.6208603837962272, -6.884901960086286188, 3.974999999999997424 ) ) ;
#121604=LINE ( 'NONE', #533, #99844 ) ;
#121632=CARTESIAN_POINT ( 'NONE',  ( 91.72959685856477563, -6.110000000000000320, -1.637169565754161393 ) ) ;
#121641=CARTESIAN_POINT ( 'NONE',  ( 48.25000000000000000, -9.735942053221458872E-16, 7.950000000000000178 ) ) ;
#121643=CARTESIAN_POINT ( 'NONE',  ( 81.57876352523143737, -7.482591942790325086E-16, 6.109999999999998543 ) ) ;
#121646=EDGE_LOOP ( 'NONE', ( #95864, #67580, #41814, #130464 ) ) ;
#121702=VERTEX_POINT ( 'NONE', #87254 ) ;
#121721=( BOUNDED_CURVE ( )  B_SPLINE_CURVE ( 2, ( #4736, #49039, #93235, #104823, #137469, #25105, #102700, #38162, #17110, #93944, #138178, #83083, #129423 ),
 .UNSPECIFIED., .F., .T. ) 
 B_SPLINE_CURVE_WITH_KNOTS ( ( 3, 2, 2, 2, 2, 2, 3 ),
 ( 0.3166666666666666519, 0.3194444444444444198, 0.3222222222222222432, 0.3250000000000000111, 0.3277777777777777790, 0.3305555555555555469, 0.3333333333333333148 ),
 .UNSPECIFIED. ) 
 CURVE ( )  GEOMETRIC_REPRESENTATION_ITEM ( )  RATIONAL_B_SPLINE_CURVE ( ( 1.000000000000000000, 0.9659258262890683122, 1.000000000000000000, 0.9659258262890683122, 1.000000000000000000, 0.9659258262890683122, 1.000000000000000000, 0.9659258262890683122, 1.000000000000000000, 0.9659258262890683122, 1.000000000000000000, 0.9659258262890683122, 1.000000000000000000 ) ) 
 REPRESENTATION_ITEM ( '' )  );
#121727=CARTESIAN_POINT ( 'NONE',  ( 80.55793019189812298, 6.110000000000001208, -1.637169565754156286 ) ) ;
#121728=CARTESIAN_POINT ( 'NONE',  ( 7.038781720212028858, -9.048404391359483157, 2.901793228214030851 ) ) ;
#121734=CARTESIAN_POINT ( 'NONE',  ( 34.78752705046288440, 0.000000000000000000, -7.949999999999998401 ) ) ;
#121773=CARTESIAN_POINT ( 'NONE',  ( 110.5208333333333286, 7.949999999999998401, 2.130196079827431532 ) ) ;
#121777=CARTESIAN_POINT ( 'NONE',  ( 102.9375000000000000, 5.819803920172573974, -5.819803920172572198 ) ) ;
#121796=CARTESIAN_POINT ( 'NONE',  ( 87.28752705046288440, 0.000000000000000000, -7.949999999999998401 ) ) ;
#121801=CARTESIAN_POINT ( 'NONE',  ( 120.7504301918981184, 3.055000000000002824, -5.291415217122919401 ) ) ;
#121810=CARTESIAN_POINT ( 'NONE',  ( 117.3079301918980946, -6.109999999999998543, 1.637169565754158063 ) ) ;
#121816=CARTESIAN_POINT ( 'NONE',  ( 97.54166666666667140, -3.975000000000002753, 6.884901960086286188 ) ) ;
#121819=CARTESIAN_POINT ( 'NONE',  ( 37.47959685856476852, 6.109999999999999432, 1.637169565754164280 ) ) ;
#121825=CARTESIAN_POINT ( 'NONE',  ( 26.45376352523144803, -6.109999999999998543, -3.741295971395162543E-16 ) ) ;
#121856=CARTESIAN_POINT ( 'NONE',  ( 50.37043019189811588, -3.055000000000001492, 5.291415217122917625 ) ) ;
#121893=CARTESIAN_POINT ( 'NONE',  ( 115.4120968585647944, 5.291415217122922066, -3.054999999999995275 ) ) ;
#121905=DIRECTION ( 'NONE',  ( 1.000000000000000000, 0.000000000000000000, 0.000000000000000000 ) ) ;
#121936=CARTESIAN_POINT ( 'NONE',  ( 26.45376352523144803, -6.109999999999999432, -3.741295971395163529E-16 ) ) ;
#121940=CARTESIAN_POINT ( 'NONE',  ( 125.1041666666666714, 2.130196079827422206, 7.950000000000001954 ) ) ;
#121953=CARTESIAN_POINT ( 'NONE',  ( 124.9795968585647756, 6.109999999999999432, 1.637169565754164280 ) ) ;
#121965=CARTESIAN_POINT ( 'NONE',  ( 46.60002705046288440, 5.819803920172570422, 5.819803920172574863 ) ) ;
#121971=CARTESIAN_POINT ( 'NONE',  ( 50.14583333333333570, 2.130196079827431976, -7.949999999999999289 ) ) ;
#121980=CARTESIAN_POINT ( 'NONE',  ( 37.33376352523143282, 6.110000000000001208, 1.122388791418549305E-15 ) ) ;
#121993=CARTESIAN_POINT ( 'NONE',  ( 86.91709685856477563, 3.054999999999998828, 5.291415217122922066 ) ) ;
#121995=DIRECTION ( 'NONE',  ( -1.000000000000000000, -0.000000000000000000, -0.000000000000000000 ) ) ;
#122004=CARTESIAN_POINT ( 'NONE',  ( 54.30793019189810167, -6.109999999999998543, 1.637169565754158063 ) ) ;
#122011=SURFACE_STYLE_FILL_AREA ( #111129 ) ;
#122032=CARTESIAN_POINT ( 'NONE',  ( 73.12043019189812298, 3.055000000000001936, -5.291415217122916737 ) ) ;
#122061=CARTESIAN_POINT ( 'NONE',  ( 26.68793019189810423, 6.110000000000002984, -1.637169565754156730 ) ) ;
#122112=VERTEX_POINT ( 'NONE', #119671 ) ;
#122119=CARTESIAN_POINT ( 'NONE',  ( 57.95376352523144448, -6.109999999999999432, -3.741295971395163529E-16 ) ) ;
#122122=CARTESIAN_POINT ( 'NONE',  ( 32.45419371712955581, 6.884901960086283523, 3.975000000000002753 ) ) ;
#122136=FACE_OUTER_BOUND ( 'NONE', #95638, .T. ) ;
#122139=CARTESIAN_POINT ( 'NONE',  ( 80.87086038379622721, 6.884901960086289741, -3.974999999999993427 ) ) ;
#122144=CARTESIAN_POINT ( 'NONE',  ( 69.25000000000000000, -9.735942053221458872E-16, 7.950000000000000178 ) ) ;
#122153=CARTESIAN_POINT ( 'NONE',  ( 62.41709685856476852, 3.054999999999998828, 5.291415217122922066 ) ) ;
#122173=CARTESIAN_POINT ( 'NONE',  ( 68.83376352523143282, 6.110000000000001208, 1.122388791418549305E-15 ) ) ;
#122204=CARTESIAN_POINT ( 'NONE',  ( 103.7454301918981230, -5.291415217122918513, -3.055000000000000160 ) ) ;
#122215=CARTESIAN_POINT ( 'NONE',  ( 71.00000000000000000, 0.000000000000000000, -7.950000000000000178 ) ) ;
#122232=CARTESIAN_POINT ( 'NONE',  ( 57.60459685856476852, 1.637169565754164946, -6.109999999999999432 ) ) ;
#122237=CARTESIAN_POINT ( 'NONE',  ( 87.35459685856476142, -1.637169565754161615, 6.110000000000000320 ) ) ;
#122248=LINE ( 'NONE', #110645, #22587 ) ;
#122252=CARTESIAN_POINT ( 'NONE',  ( 123.2870968585647944, 3.054999999999997495, 5.291415217122919401 ) ) ;
#122289=CARTESIAN_POINT ( 'NONE',  ( 41.68749999999997868, -5.819803920172573974, 5.819803920172573086 ) ) ;
#122299=CARTESIAN_POINT ( 'NONE',  ( 110.4750270504628702, -5.819803920172572198, 5.819803920172572198 ) ) ;
#122314=CARTESIAN_POINT ( 'NONE',  ( 90.12543019189811844, 5.291415217122919401, 3.055000000000002824 ) ) ;
#122340=CARTESIAN_POINT ( 'NONE',  ( 89.68793019189810423, 6.110000000000002984, -1.637169565754156730 ) ) ;
#122346=CARTESIAN_POINT ( 'NONE',  ( 85.24586038379622721, 3.974999999999996980, 6.884901960086287964 ) ) ;
#122352=CARTESIAN_POINT ( 'NONE',  ( 88.28709685856478018, 3.054999999999997495, 5.291415217122919401 ) ) ;
#122369=AXIS2_PLACEMENT_3D ( 'NONE', #806, #86432, #68 ) ;
#122390=CYLINDRICAL_SURFACE ( 'NONE', #101681, 7.950000000000000178 ) ;
#122412=CARTESIAN_POINT ( 'NONE',  ( 117.1045968585647756, 1.637169565754164946, -6.109999999999999432 ) ) ;
#122414=EDGE_CURVE ( 'NONE', #63944, #128763, #62301, .T. ) ;
#122431=DIRECTION ( 'NONE',  ( -1.000000000000000000, 0.000000000000000000, -0.000000000000000000 ) ) ;
#122432=CARTESIAN_POINT ( 'NONE',  ( 106.5375270504628844, -9.735942053221456900E-16, 7.949999999999998401 ) ) ;
#122444=CARTESIAN_POINT ( 'NONE',  ( 86.09959685856478018, -6.109999999999998543, -1.637169565754160727 ) ) ;
#122446=CARTESIAN_POINT ( 'NONE',  ( 98.07919371712955581, 3.975000000000002753, -6.884901960086283523 ) ) ;
#122478=CARTESIAN_POINT ( 'NONE',  ( 47.62086038379622011, -6.884901960086286188, 3.974999999999997424 ) ) ;
#122492=CARTESIAN_POINT ( 'NONE',  ( 102.7916666666666714, 3.975000000000003642, -6.884901960086285300 ) ) ;
#122499=CARTESIAN_POINT ( 'NONE',  ( 13.79777835071270076, 9.118581059549645929, 2.675923548408995156 ) ) ;
#122519=CARTESIAN_POINT ( 'NONE',  ( 85.53752705046288440, -9.735942053221456900E-16, 7.949999999999998401 ) ) ;
#122525=CARTESIAN_POINT ( 'NONE',  ( 116.2295968585647756, -6.110000000000000320, -1.637169565754161393 ) ) ;
#122535=CARTESIAN_POINT ( 'NONE',  ( 116.1412635252314374, 4.472830434245836706, 4.472830434245840259 ) ) ;
#122539=CARTESIAN_POINT ( 'NONE',  ( 98.56250000000000000, -5.819803920172573086, -5.819803920172573974 ) ) ;
#122543=CARTESIAN_POINT ( 'NONE',  ( 38.64626352523144703, -4.472830434245840259, 4.472830434245839371 ) ) ;
#122547=CARTESIAN_POINT ( 'NONE',  ( 31.70376352523145158, 6.109999999999998543, 1.122388791418548911E-15 ) ) ;
#122581=CARTESIAN_POINT ( 'NONE',  ( 47.45376352523145158, -6.109999999999998543, -3.741295971395162543E-16 ) ) ;
#122621=CARTESIAN_POINT ( 'NONE',  ( 113.6620968585647944, -5.291415217122919401, 3.054999999999998384 ) ) ;
#122637=EDGE_CURVE ( 'NONE', #121702, #49011, #121538, .T. ) ;
#122660=CARTESIAN_POINT ( 'NONE',  ( 32.87043019189811588, -3.055000000000001936, 5.291415217122918513 ) ) ;
#122680=CARTESIAN_POINT ( 'NONE',  ( 122.9379301918981042, -6.110000000000001208, 1.637169565754158951 ) ) ;
#122690=CARTESIAN_POINT ( 'NONE',  ( 44.26669371712954870, -7.949999999999999289, 2.130196079827424427 ) ) ;
#122696=CARTESIAN_POINT ( 'NONE',  ( 43.29166666666665719, 3.975000000000003642, -6.884901960086285300 ) ) ;
#122708=CARTESIAN_POINT ( 'NONE',  ( 38.93793019189809002, -6.110000000000001208, 1.637169565754158951 ) ) ;
#122732=EDGE_CURVE ( 'NONE', #116147, #7244, #105032, .T. ) ;
#122736=CARTESIAN_POINT ( 'NONE',  ( 59.84959685856477307, 6.109999999999996767, 1.637169565754163836 ) ) ;
#122739=DIRECTION ( 'NONE',  ( -1.000000000000000000, -0.000000000000000000, -0.000000000000000000 ) ) ;
#122762=CARTESIAN_POINT ( 'NONE',  ( 71.22459685856478018, -1.637169565754160949, 6.109999999999997655 ) ) ;
#122770=CARTESIAN_POINT ( 'NONE',  ( 123.2083333333333428, -3.974999999999999201, -6.884901960086287964 ) ) ;
#122795=CARTESIAN_POINT ( 'NONE',  ( 30.77126352523143638, 4.472830434245838482, 4.472830434245842035 ) ) ;
#122836=CARTESIAN_POINT ( 'NONE',  ( 25.02392480454907187, -6.350000000000004974, -3.888253587292851012E-16 ) ) ;
#122850=CARTESIAN_POINT ( 'NONE',  ( 58.82876352523144448, 0.000000000000000000, -6.109999999999999432 ) ) ;
#122862=CARTESIAN_POINT ( 'NONE',  ( 0.000000000000000000, 0.000000000000000000, 0.000000000000000000 ) ) ;
#122871=CARTESIAN_POINT ( 'NONE',  ( 71.24586038379622721, 3.974999999999996980, 6.884901960086287964 ) ) ;
#122876=CARTESIAN_POINT ( 'NONE',  ( 72.16666666666665719, 6.884901960086285300, 3.975000000000003642 ) ) ;
#122889=CARTESIAN_POINT ( 'NONE',  ( 63.29209685856476852, -5.291415217122921177, 3.054999999999999272 ) ) ;
#122912=CARTESIAN_POINT ( 'NONE',  ( 56.43793019189809712, -6.110000000000001208, 1.637169565754158951 ) ) ;
#122947=CARTESIAN_POINT ( 'NONE',  ( 100.9745968585647660, 1.637169565754164280, -6.109999999999996767 ) ) ;
#122962=CARTESIAN_POINT ( 'NONE',  ( 26.99999999999998579, -7.850927237173508821, -1.251176053402193178 ) ) ;
#122966=CARTESIAN_POINT ( 'NONE',  ( 87.62500000000001421, -7.950000000000000178, -4.867971026610729436E-16 ) ) ;
#122972=CARTESIAN_POINT ( 'NONE',  ( 56.87543019189809712, -5.291415217122920289, -3.055000000000001492 ) ) ;
#122977=CARTESIAN_POINT ( 'NONE',  ( 94.20876352523144703, -7.482591942790329030E-16, 6.110000000000001208 ) ) ;
#122981=EDGE_LOOP ( 'NONE', ( #59054, #42099, #105337, #34000 ) ) ;
#122983=VECTOR ( 'NONE', #83428, 1000.000000000000000 ) ;
#123001=FACE_OUTER_BOUND ( 'NONE', #64565, .T. ) ;
#123008=EDGE_LOOP ( 'NONE', ( #97454, #132674, #134659, #9353 ) ) ;
#123023=CARTESIAN_POINT ( 'NONE',  ( 9.748310473850249736, 8.447540412293815137, -4.346633328725724610 ) ) ;
#123051=CARTESIAN_POINT ( 'NONE',  ( 106.9750270504628986, -5.819803920172572198, 5.819803920172572198 ) ) ;
#123071=CARTESIAN_POINT ( 'NONE',  ( 91.43793019189810423, -6.110000000000001208, 1.637169565754158951 ) ) ;
#123091=CARTESIAN_POINT ( 'NONE',  ( 86.75000000000000000, -9.735942053221458872E-16, 7.950000000000000178 ) ) ;
#123096=CARTESIAN_POINT ( 'NONE',  ( 94.35459685856476142, -1.637169565754161615, 6.110000000000000320 ) ) ;
#123108=CARTESIAN_POINT ( 'NONE',  ( 103.5208333333333428, 7.949999999999998401, 2.130196079827431532 ) ) ;
#123113=CARTESIAN_POINT ( 'NONE',  ( 84.20376352523145158, 6.109999999999998543, 1.122388791418548911E-15 ) ) ;
#123122=VECTOR ( 'NONE', #18853, 1000.000000000000000 ) ;
#123144=CARTESIAN_POINT ( 'NONE',  ( 56.66252705046289151, 7.949999999999998401, 1.460391307983218338E-15 ) ) ;
#123155=CARTESIAN_POINT ( 'NONE',  ( 115.8708603837962414, 6.884901960086289741, -3.974999999999993427 ) ) ;
#123164=CARTESIAN_POINT ( 'NONE',  ( 114.4795968585647614, 6.109999999999999432, 1.637169565754164280 ) ) ;
#123198=CARTESIAN_POINT ( 'NONE',  ( 83.18293019189810877, -1.637169565754159173, -6.109999999999999432 ) ) ;
#123204=ORIENTED_EDGE ( 'NONE', *, *, #128286, .F. ) ;
#123253=CARTESIAN_POINT ( 'NONE',  ( 88.93750000000000000, 5.819803920172573974, -5.819803920172572198 ) ) ;
#123281=CARTESIAN_POINT ( 'NONE',  ( 118.5629301918981042, 1.637169565754157174, 6.110000000000002984 ) ) ;
#123292=CARTESIAN_POINT ( 'NONE',  ( 111.4745968585647944, 1.637169565754164058, -6.109999999999996767 ) ) ;
#123302=CARTESIAN_POINT ( 'NONE',  ( 25.02392480454907187, -6.350000000000004974, -3.888253587292851012E-16 ) ) ;
#123306=CARTESIAN_POINT ( 'NONE',  ( 33.59959685856477307, -6.109999999999997655, -1.637169565754160283 ) ) ;
#123307=ORIENTED_EDGE ( 'NONE', *, *, #46153, .T. ) ;
#123338=CARTESIAN_POINT ( 'NONE',  ( 49.93293019189810167, 1.637169565754156508, 6.110000000000000320 ) ) ;
#123355=ORIENTED_EDGE ( 'NONE', *, *, #83332, .T. ) ;
#123361=ORIENTED_EDGE ( 'NONE', *, *, #46899, .F. ) ;
#123375=CARTESIAN_POINT ( 'NONE',  ( 107.6829301918981088, -1.637169565754159173, -6.109999999999999432 ) ) ;
#123379=CARTESIAN_POINT ( 'NONE',  ( 0.000000000000000000, 0.000000000000000000, 6.349999999999999645 ) ) ;
#123417=CARTESIAN_POINT ( 'NONE',  ( 0.000000000000000000, 9.735942053221458872E-16, -7.950000000000000178 ) ) ;
#123422=CARTESIAN_POINT ( 'NONE',  ( 125.7882715818462174, -5.693400499257576186, 5.136054288641274113 ) ) ;
#123446=CARTESIAN_POINT ( 'NONE',  ( 123.5212635252314470, -4.472830434245839371, -4.472830434245840259 ) ) ;
#123450=CARTESIAN_POINT ( 'NONE',  ( 78.29166666666665719, 3.975000000000003642, -6.884901960086285300 ) ) ;
#123455=CARTESIAN_POINT ( 'NONE',  ( 44.99586038379622721, -3.974999999999998312, -6.884901960086286188 ) ) ;
#123461=CARTESIAN_POINT ( 'NONE',  ( 49.99999999999998579, 0.000000000000000000, -7.950000000000000178 ) ) ;
#123465=CARTESIAN_POINT ( 'NONE',  ( 127.0000000000000568, -4.172191364199829167, -4.786994800550450790 ) ) ;
#123468=CARTESIAN_POINT ( 'NONE',  ( 33.83376352523143282, 6.110000000000001208, 1.122388791418549305E-15 ) ) ;
#123492=CARTESIAN_POINT ( 'NONE',  ( 55.47459685856478018, 1.637169565754164058, -6.109999999999996767 ) ) ;
#123520=CARTESIAN_POINT ( 'NONE',  ( 76.03709685856478018, -3.054999999999998828, -5.291415217122919401 ) ) ;
#123546=AXIS2_PLACEMENT_3D ( 'NONE', #117564, #50930, #18246 ) ;
#123547=CARTESIAN_POINT ( 'NONE',  ( 42.66252705046289151, 7.949999999999998401, 1.460391307983218338E-15 ) ) ;
#123599=CARTESIAN_POINT ( 'NONE',  ( 55.47459685856478018, 1.637169565754164280, -6.109999999999997655 ) ) ;
#123605=ADVANCED_FACE ( 'NONE', ( #79684 ), #123867, .T. ) ;
#123612=CYLINDRICAL_SURFACE ( 'NONE', #20918, 7.950000000000000178 ) ;
#123622=CARTESIAN_POINT ( 'NONE',  ( 74.01669371712955581, 7.950000000000001066, -2.130196079827421318 ) ) ;
#123627=CARTESIAN_POINT ( 'NONE',  ( 75.66666666666665719, 6.884901960086285300, 3.975000000000003642 ) ) ;
#123637=CARTESIAN_POINT ( 'NONE',  ( 63.58376352523143993, -6.110000000000001208, -3.741295971395164515E-16 ) ) ;
#123642=CARTESIAN_POINT ( 'NONE',  ( 44.75000000000000000, -9.735942053221458872E-16, 7.950000000000000178 ) ) ;
#123653=CARTESIAN_POINT ( 'NONE',  ( 58.33376352523143993, 6.110000000000001208, 1.122388791418549305E-15 ) ) ;
#123685=CARTESIAN_POINT ( 'NONE',  ( 99.22459685856478018, -1.637169565754160949, 6.109999999999997655 ) ) ;
#123708=CARTESIAN_POINT ( 'NONE',  ( 57.45876352523143993, 0.000000000000000000, -6.110000000000001208 ) ) ;
#123713=CARTESIAN_POINT ( 'NONE',  ( 93.62543019189811844, 5.291415217122919401, 3.055000000000002824 ) ) ;
#123729=VERTEX_POINT ( 'NONE', #25964 ) ;
#123753=CARTESIAN_POINT ( 'NONE',  ( 94.28752705046289861, 0.000000000000000000, -7.949999999999998401 ) ) ;
#123760=CARTESIAN_POINT ( 'NONE',  ( 0.000000000000000000, 5.817072295949924468E-16, -4.749999999999997335 ) ) ;
#123778=CARTESIAN_POINT ( 'NONE',  ( 104.7875270504628986, 0.000000000000000000, -7.949999999999998401 ) ) ;
#123796=CARTESIAN_POINT ( 'NONE',  ( 91.72959685856477563, -6.110000000000000320, -1.637169565754161393 ) ) ;
#123813=FACE_OUTER_BOUND ( 'NONE', #105865, .T. ) ;
#123818=CARTESIAN_POINT ( 'NONE',  ( 87.64626352523141861, -4.472830434245840259, 4.472830434245839371 ) ) ;
#123831=CARTESIAN_POINT ( 'NONE',  ( 80.26626352523145158, 4.472830434245839371, -4.472830434245838482 ) ) ;
#123867=CYLINDRICAL_SURFACE ( 'NONE', #82779, 7.950000000000000178 ) ;
#123869=CARTESIAN_POINT ( 'NONE',  ( 0.000000000000000000, 0.000000000000000000, 7.950000000000000178 ) ) ;
#123870=ORIENTED_EDGE ( 'NONE', *, *, #120106, .T. ) ;
#123874=B_SPLINE_CURVE_WITH_KNOTS ( 'NONE', 1,
 ( #29573, #60840 ),
 .UNSPECIFIED., .F., .F.,
 ( 2, 2 ),
 ( 0.000000000000000000, 1.000000000000000000 ),
 .UNSPECIFIED. ) ;
#123876=CARTESIAN_POINT ( 'NONE',  ( 94.04166666666665719, -3.975000000000002753, 6.884901960086286188 ) ) ;
#123881=CARTESIAN_POINT ( 'NONE',  ( 122.5004301918981184, -3.055000000000002380, 5.291415217122920289 ) ) ;
#123912=CARTESIAN_POINT ( 'NONE',  ( 79.82876352523145158, 0.000000000000000000, -6.109999999999999432 ) ) ;
#123946=CARTESIAN_POINT ( 'NONE',  ( 48.05836038379622011, -7.949999999999996625, -2.130196079827426203 ) ) ;
#123958=CARTESIAN_POINT ( 'NONE',  ( 91.70833333333334281, -3.974999999999999201, -6.884901960086287964 ) ) ;
#123982=CARTESIAN_POINT ( 'NONE',  ( 115.7920968585647756, -5.291415217122921177, 3.054999999999999272 ) ) ;
#123986=CARTESIAN_POINT ( 'NONE',  ( 99.72916666666665719, 7.950000000000001954, -2.130196079827421762 ) ) ;
#123991=CARTESIAN_POINT ( 'NONE',  ( 113.0787635252314516, -7.482591942790325086E-16, 6.109999999999998543 ) ) ;
#124003=CARTESIAN_POINT ( 'NONE',  ( 27.18293019189811588, -1.637169565754158951, -6.109999999999998543 ) ) ;
#124011=FACE_OUTER_BOUND ( 'NONE', #98450, .T. ) ;
#124032=CARTESIAN_POINT ( 'NONE',  ( 41.76626352523145158, 4.472830434245838482, -4.472830434245837594 ) ) ;
#124041=ADVANCED_FACE ( 'NONE', ( #13279 ), #101741, .T. ) ;
#124065=CARTESIAN_POINT ( 'NONE',  ( 114.0995968585647660, -6.109999999999998543, -1.637169565754160727 ) ) ;
#124104=CARTESIAN_POINT ( 'NONE',  ( 126.4306647761266049, -6.963203063247377145, -0.9358753878083012623 ) ) ;
#124109=CARTESIAN_POINT ( 'NONE',  ( 122.3333333333333286, -6.884901960086287964, 3.974999999999998312 ) ) ;
#124121=CARTESIAN_POINT ( 'NONE',  ( 120.0212635252314328, -4.472830434245839371, -4.472830434245840259 ) ) ;
#124125=CARTESIAN_POINT ( 'NONE',  ( 78.00000000000000000, 0.000000000000000000, -7.950000000000000178 ) ) ;
#124130=CARTESIAN_POINT ( 'NONE',  ( 44.41252705046289151, -7.949999999999998401, -4.867971026610728450E-16 ) ) ;
#124136=CARTESIAN_POINT ( 'NONE',  ( 43.87500000000000000, 7.950000000000000178, 1.460391307983218535E-15 ) ) ;
#124144=CARTESIAN_POINT ( 'NONE',  ( 36.60459685856475431, 1.637169565754164946, -6.109999999999999432 ) ) ;
#124171=CARTESIAN_POINT ( 'NONE',  ( 54.74543019189812298, -5.291415217122918513, -3.055000000000000160 ) ) ;
#124199=CARTESIAN_POINT ( 'NONE',  ( 73.41209685856478018, 5.291415217122921177, -3.054999999999994831 ) ) ;
#124209=CARTESIAN_POINT ( 'NONE',  ( 102.5000000000000142, 0.000000000000000000, -7.950000000000000178 ) ) ;
#124210=DIRECTION ( 'NONE',  ( 0.000000000000000000, 0.000000000000000000, 1.000000000000000000 ) ) ;
#124223=CARTESIAN_POINT ( 'NONE',  ( 26.25043019189810067, 3.055000000000002824, -5.291415217122919401 ) ) ;
#124227=CARTESIAN_POINT ( 'NONE',  ( 43.53752705046289151, -9.735942053221456900E-16, 7.949999999999998401 ) ) ;
#124247=CARTESIAN_POINT ( 'NONE',  ( 28.27083333333332860, -7.949999999999998401, -2.130196079827426203 ) ) ;
#124275=CARTESIAN_POINT ( 'NONE',  ( 60.14126352523143737, 4.472830434245837594, 4.472830434245841147 ) ) ;
#124286=CARTESIAN_POINT ( 'NONE',  ( 33.03752705046289151, -9.735942053221456900E-16, 7.949999999999998401 ) ) ;
#124299=CARTESIAN_POINT ( 'NONE',  ( 79.12086038379622721, -6.884901960086286188, 3.974999999999997424 ) ) ;
#124301=VECTOR ( 'NONE', #114081, 1000.000000000000000 ) ;
#124304=CARTESIAN_POINT ( 'NONE',  ( 76.25000000000000000, -9.735942053221458872E-16, 7.950000000000000178 ) ) ;
#124312=CARTESIAN_POINT ( 'NONE',  ( 65.18793019189811844, 6.110000000000002984, -1.637169565754156730 ) ) ;
#124327=CARTESIAN_POINT ( 'NONE',  ( 127.0000000000000000, 7.776507174585694135E-16, -6.350000000000001421 ) ) ;
#124334=ADVANCED_FACE ( 'NONE', ( #78399 ), #10263, .T. ) ;
#124335=CARTESIAN_POINT ( 'NONE',  ( 57.16709685856477563, -3.055000000000000160, -5.291415217122921177 ) ) ;
#124371=CARTESIAN_POINT ( 'NONE',  ( 106.2245968585647802, -1.637169565754160949, 6.109999999999997655 ) ) ;
#124377=CARTESIAN_POINT ( 'NONE',  ( 0.000000000000000000, 7.776507174585692163E-16, -6.349999999999999645 ) ) ;
#124393=CARTESIAN_POINT ( 'NONE',  ( 58.91709685856477563, 3.054999999999998828, 5.291415217122922066 ) ) ;
#124399=CARTESIAN_POINT ( 'NONE',  ( 88.95876352523143282, 0.000000000000000000, -6.110000000000001208 ) ) ;
#124410=CARTESIAN_POINT ( 'NONE',  ( 125.1829301918981372, -1.637169565754159173, -6.109999999999999432 ) ) ;
#124435=UNCERTAINTY_MEASURE_WITH_UNIT (LENGTH_MEASURE( 1.000000000000000082E-05 ), #114529, 'distance_accuracy_value', 'NONE');
#124469=CARTESIAN_POINT ( 'NONE',  ( 99.97502705046289861, -5.819803920172572198, 5.819803920172572198 ) ) ;
#124483=CARTESIAN_POINT ( 'NONE',  ( 97.27126352523143282, 4.472830434245839371, 4.472830434245842035 ) ) ;
#124499=CARTESIAN_POINT ( 'NONE',  ( 103.0375270504628986, -9.735942053221456900E-16, 7.949999999999998401 ) ) ;
#124507=CARTESIAN_POINT ( 'NONE',  ( 82.68793019189809002, 6.110000000000002984, -1.637169565754156730 ) ) ;
#124521=( BOUNDED_CURVE ( )  B_SPLINE_CURVE ( 2, ( #64165, #97477, #143139, #19221, #8997, #118524, #8304, #31532, #63480, #130866, #75063, #86642, #9761 ),
 .UNSPECIFIED., .F., .F. ) 
 B_SPLINE_CURVE_WITH_KNOTS ( ( 3, 2, 2, 2, 2, 2, 3 ),
 ( 0.1833333333333333204, 0.1861111111111111160, 0.1888888888888888840, 0.1916666666666666796, 0.1944444444444444475, 0.1972222222222222154, 0.2000000000000000111 ),
 .UNSPECIFIED. ) 
 CURVE ( )  GEOMETRIC_REPRESENTATION_ITEM ( )  RATIONAL_B_SPLINE_CURVE ( ( 1.000000000000000000, 0.9659258262890683122, 1.000000000000000000, 0.9659258262890683122, 1.000000000000000000, 0.9659258262890683122, 1.000000000000000000, 0.9659258262890683122, 1.000000000000000000, 0.9659258262890683122, 1.000000000000000000, 0.9659258262890683122, 1.000000000000000000 ) ) 
 REPRESENTATION_ITEM ( '' )  );
#124523=CARTESIAN_POINT ( 'NONE',  ( 79.82876352523145158, 0.000000000000000000, -6.109999999999998543 ) ) ;
#124539=CARTESIAN_POINT ( 'NONE',  ( 1.500000000000000000, 0.000000000000000000, -8.000000000000001776 ) ) ;
#124550=DIRECTION ( 'NONE',  ( -7.447409204830965619E-33, 6.123233995736750012E-17, -1.000000000000000000 ) ) ;
#124573=CARTESIAN_POINT ( 'NONE',  ( 121.7712635252314328, 4.472830434245838482, 4.472830434245842035 ) ) ;
#124596=AXIS2_PLACEMENT_3D ( 'NONE', #75544, #94588, #20413 ) ;
#124650=CARTESIAN_POINT ( 'NONE',  ( 95.06250000000000000, -5.819803920172572198, -5.819803920172573086 ) ) ;
#124657=CARTESIAN_POINT ( 'NONE',  ( 12.52989244501176813, 8.713222490859248381, -3.789296364347416901 ) ) ;
#124665=CARTESIAN_POINT ( 'NONE',  ( 126.1498859171888114, 5.910167777758539742, -4.315024036782260985 ) ) ;
#124667=CARTESIAN_POINT ( 'NONE',  ( 126.7870968585647944, 3.054999999999997495, 5.291415217122919401 ) ) ;
#124679=CARTESIAN_POINT ( 'NONE',  ( 106.8962635252314328, 4.472830434245840259, -4.472830434245839371 ) ) ;
#124680=( BOUNDED_CURVE ( )  B_SPLINE_CURVE ( 2, ( #33139, #440, #120800, #65027, #30226, #130283, #96872, #88199, #41825, #141878, #118666, #86045, #109930 ),
 .UNSPECIFIED., .F., .T. ) 
 B_SPLINE_CURVE_WITH_KNOTS ( ( 3, 2, 2, 2, 2, 2, 3 ),
 ( 0.6666666666666666297, 0.6694444444444443976, 0.6722222222222222765, 0.6750000000000000444, 0.6777777777777778123, 0.6805555555555555802, 0.6833333333333333481 ),
 .UNSPECIFIED. ) 
 CURVE ( )  GEOMETRIC_REPRESENTATION_ITEM ( )  RATIONAL_B_SPLINE_CURVE ( ( 1.000000000000000000, 0.9659258262890683122, 1.000000000000000000, 0.9659258262890683122, 1.000000000000000000, 0.9659258262890683122, 1.000000000000000000, 0.9659258262890683122, 1.000000000000000000, 0.9659258262890683122, 1.000000000000000000, 0.9659258262890683122, 1.000000000000000000 ) ) 
 REPRESENTATION_ITEM ( '' )  );
#124691=CARTESIAN_POINT ( 'NONE',  ( 103.0162635252314374, -4.472830434245839371, 4.472830434245839371 ) ) ;
#124725=CARTESIAN_POINT ( 'NONE',  ( 62.93336038379622721, 2.130196079827431532, -7.949999999999996625 ) ) ;
#124736=CARTESIAN_POINT ( 'NONE',  ( 41.32876352523144448, 0.000000000000000000, -6.109999999999998543 ) ) ;
#124754=VECTOR ( 'NONE', #56139, 1000.000000000000000 ) ;
#124771=CARTESIAN_POINT ( 'NONE',  ( 112.4954301918981230, 5.291415217122917625, 3.055000000000002380 ) ) ;
#124805=VECTOR ( 'NONE', #130469, 1000.000000000000000 ) ;
#124822=CARTESIAN_POINT ( 'NONE',  ( 116.5000000000000000, 0.000000000000000000, -7.950000000000000178 ) ) ;
#124829=ORIENTED_EDGE ( 'NONE', *, *, #132062, .T. ) ;
#124833=CARTESIAN_POINT ( 'NONE',  ( 111.4170968585647614, 3.054999999999998828, 5.291415217122922066 ) ) ;
#124842=CARTESIAN_POINT ( 'NONE',  ( 42.95419371712954870, 6.884901960086283523, 3.975000000000002753 ) ) ;
#124847=CARTESIAN_POINT ( 'NONE',  ( 35.27083333333330728, -7.949999999999999289, -2.130196079827426203 ) ) ;
#124858=CARTESIAN_POINT ( 'NONE',  ( 128.2454301918981230, -5.291415217122918513, -3.055000000000000160 ) ) ;
#124882=CARTESIAN_POINT ( 'NONE',  ( 57.66209685856478728, -5.291415217122919401, 3.054999999999997939 ) ) ;
#124909=ORIENTED_EDGE ( 'NONE', *, *, #82817, .T. ) ;
#124913=CARTESIAN_POINT ( 'NONE',  ( 62.03709685856478728, -3.054999999999998828, -5.291415217122919401 ) ) ;
#124934=CARTESIAN_POINT ( 'NONE',  ( 41.78752705046289151, 0.000000000000000000, -7.949999999999998401 ) ) ;
#124963=CARTESIAN_POINT ( 'NONE',  ( 78.00000000000000000, 0.000000000000000000, -7.950000000000000178 ) ) ;
#124986=CARTESIAN_POINT ( 'NONE',  ( 57.07876352523144448, -7.482591942790327058E-16, 6.109999999999999432 ) ) ;
#125009=CARTESIAN_POINT ( 'NONE',  ( 117.2291666666666572, 7.950000000000001954, -2.130196079827421762 ) ) ;
#125010=CARTESIAN_POINT ( 'NONE',  ( 73.72502705046288440, 5.819803920172573086, -5.819803920172572198 ) ) ;
#125013=CARTESIAN_POINT ( 'NONE',  ( 63.85416666666665719, -2.130196079827425315, -7.950000000000001066 ) ) ;
#125023=CARTESIAN_POINT ( 'NONE',  ( 63.72959685856477563, -6.110000000000000320, -1.637169565754161393 ) ) ;
#125047=CARTESIAN_POINT ( 'NONE',  ( 111.0583603837962130, -7.949999999999996625, -2.130196079827426203 ) ) ;
#125049=VERTEX_POINT ( 'NONE', #64327 ) ;
#125068=FACE_OUTER_BOUND ( 'NONE', #87720, .T. ) ;
#125076=CARTESIAN_POINT ( 'NONE',  ( 94.84959685856476597, 6.109999999999996767, 1.637169565754163836 ) ) ;
#125081=EDGE_CURVE ( 'NONE', #18455, #73811, #76654, .T. ) ;
#125102=CARTESIAN_POINT ( 'NONE',  ( 49.72959685856476852, -6.110000000000000320, -1.637169565754161393 ) ) ;
#125133=CARTESIAN_POINT ( 'NONE',  ( 0.000000000000000000, 0.000000000000000000, 7.950000000000000178 ) ) ;
#125135=EDGE_CURVE ( 'NONE', #139751, #83228, #122248, .T. ) ;
#125152=CARTESIAN_POINT ( 'NONE',  ( 10.32500000000000107, 8.432637487761466488, -4.375000000000001776 ) ) ;
#125184=CARTESIAN_POINT ( 'NONE',  ( 106.2458603837962272, 3.974999999999996980, 6.884901960086287964 ) ) ;
#125202=CARTESIAN_POINT ( 'NONE',  ( 91.29209685856477563, -5.291415217122921177, 3.054999999999999272 ) ) ;
#125216=DIRECTION ( 'NONE',  ( -1.000000000000000000, -0.000000000000000000, -0.000000000000000000 ) ) ;
#125224=CARTESIAN_POINT ( 'NONE',  ( 83.85459685856478984, -1.637169565754161615, 6.110000000000000320 ) ) ;
#125233=CARTESIAN_POINT ( 'NONE',  ( 103.6666666666666714, 6.884901960086285300, 3.975000000000003642 ) ) ;
#125235=CARTESIAN_POINT ( 'NONE',  ( 73.84959685856480860, 6.109999999999996767, 1.637169565754163836 ) ) ;
#125245=CARTESIAN_POINT ( 'NONE',  ( 45.28752705046289151, 0.000000000000000000, -7.949999999999998401 ) ) ;
#125289=CARTESIAN_POINT ( 'NONE',  ( 114.9170968585647756, 3.054999999999998828, 5.291415217122922066 ) ) ;
#125324=CARTESIAN_POINT ( 'NONE',  ( 11.75018676184482835, -8.548269360537348760, 4.146342017647454803 ) ) ;
#125360=CARTESIAN_POINT ( 'NONE',  ( 28.93293019189811943, 1.637169565754156730, 6.110000000000001208 ) ) ;
#125376=CARTESIAN_POINT ( 'NONE',  ( 90.97916666666667140, -7.950000000000001066, 2.130196079827424427 ) ) ;
#125387=CARTESIAN_POINT ( 'NONE',  ( 11.74803111135162226, 8.547913778412416619, -4.147067623587493479 ) ) ;
#125393=CARTESIAN_POINT ( 'NONE',  ( 125.5279775329496630, -3.465570510557019812, -7.141980925050981810 ) ) ;
#125404=CARTESIAN_POINT ( 'NONE',  ( 109.2295968585647614, -6.110000000000000320, -1.637169565754161393 ) ) ;
#125407=EDGE_CURVE ( 'NONE', #92088, #122112, #124521, .T. ) ;
#125415=CARTESIAN_POINT ( 'NONE',  ( 104.4745968585647802, 1.637169565754164058, -6.109999999999996767 ) ) ;
#125416=EDGE_LOOP ( 'NONE', ( #38832, #89132, #67129 ) ) ;
#125462=CARTESIAN_POINT ( 'NONE',  ( 37.97459685856477307, 1.637169565754164280, -6.109999999999996767 ) ) ;
#125479=ORIENTED_EDGE ( 'NONE', *, *, #99244, .T. ) ;
#125487=ORIENTED_EDGE ( 'NONE', *, *, #79927, .T. ) ;
#125497=ORIENTED_EDGE ( 'NONE', *, *, #83237, .F. ) ;
#125498=CARTESIAN_POINT ( 'NONE',  ( 97.76626352523143737, 4.472830434245839371, -4.472830434245839371 ) ) ;
#125506=ORIENTED_EDGE ( 'NONE', *, *, #24180, .F. ) ;
#125535=CARTESIAN_POINT ( 'NONE',  ( 112.2708333333333144, -7.949999999999998401, -2.130196079827426203 ) ) ;
#125555=CARTESIAN_POINT ( 'NONE',  ( 123.0625000000000142, -5.819803920172572198, -5.819803920172573086 ) ) ;
#125567=CARTESIAN_POINT ( 'NONE',  ( 111.5629301918981184, 1.637169565754157174, 6.110000000000002984 ) ) ;
#125576=( BOUNDED_CURVE ( )  B_SPLINE_CURVE ( 2, ( #99621, #13318, #35855, #100368, #80071, #124247, #24921, #1018, #47456, #91622, #34388, #78608, #11159 ),
 .UNSPECIFIED., .F., .F. ) 
 B_SPLINE_CURVE_WITH_KNOTS ( ( 3, 2, 2, 2, 2, 2, 3 ),
 ( 0.9333333333333333481, 0.9361111111111111160, 0.9388888888888888840, 0.9416666666666666519, 0.9444444444444444198, 0.9472222222222221877, 0.9499999999999999556 ),
 .UNSPECIFIED. ) 
 CURVE ( )  GEOMETRIC_REPRESENTATION_ITEM ( )  RATIONAL_B_SPLINE_CURVE ( ( 1.000000000000000000, 0.9659258262890683122, 1.000000000000000000, 0.9659258262890683122, 1.000000000000000000, 0.9659258262890683122, 1.000000000000000000, 0.9659258262890683122, 1.000000000000000000, 0.9659258262890683122, 1.000000000000000000, 0.9659258262890683122, 1.000000000000000000 ) ) 
 REPRESENTATION_ITEM ( '' )  );
#125579=CARTESIAN_POINT ( 'NONE',  ( 35.22502705046287730, 5.819803920172573086, -5.819803920172572198 ) ) ;
#125585=CARTESIAN_POINT ( 'NONE',  ( 39.49999999999999289, 0.000000000000000000, -7.950000000000000178 ) ) ;
#125598=CARTESIAN_POINT ( 'NONE',  ( 31.79209685856476852, -5.291415217122921177, 3.054999999999999272 ) ) ;
#125615=CARTESIAN_POINT ( 'NONE',  ( 44.82876352523145158, 0.000000000000000000, -6.109999999999998543 ) ) ;
#125616=CARTESIAN_POINT ( 'NONE',  ( 124.5208333333333286, 7.949999999999998401, 2.130196079827431532 ) ) ;
#125620=FACE_OUTER_BOUND ( 'NONE', #23975, .T. ) ;
#125642=CARTESIAN_POINT ( 'NONE',  ( 64.80793019189812298, -6.109999999999998543, 1.637169565754158507 ) ) ;
#125681=VERTEX_POINT ( 'NONE', #30464 ) ;
#125723=CARTESIAN_POINT ( 'NONE',  ( 47.59959685856478018, -6.109999999999998543, -1.637169565754160727 ) ) ;
#125747=CARTESIAN_POINT ( 'NONE',  ( 68.76669371712957002, -7.949999999999999289, 2.130196079827424427 ) ) ;
#125752=CARTESIAN_POINT ( 'NONE',  ( 66.47916666666665719, -7.950000000000001066, 2.130196079827424427 ) ) ;
#125756=AXIS2_PLACEMENT_3D ( 'NONE', #23419, #69101, #2359 ) ;
#125762=CARTESIAN_POINT ( 'NONE',  ( 57.31293019189811133, -1.637169565754159617, -6.110000000000001208 ) ) ;
#125772=CARTESIAN_POINT ( 'NONE',  ( 86.60416666666667140, 2.130196079827460398, 7.949999999999981526 ) ) ;
#125784=CARTESIAN_POINT ( 'NONE',  ( 111.7875270504628986, 0.000000000000000000, -7.949999999999998401 ) ) ;
#125796=CARTESIAN_POINT ( 'NONE',  ( 62.64169371712956291, -2.130196079827424871, -7.949999999999998401 ) ) ;
#125812=CARTESIAN_POINT ( 'NONE',  ( 89.45376352523146579, -6.109999999999998543, -3.741295971395162543E-16 ) ) ;
#125821=CARTESIAN_POINT ( 'NONE',  ( 35.99999999999999289, 0.000000000000000000, -7.950000000000000178 ) ) ;
#125824=CARTESIAN_POINT ( 'NONE',  ( 111.2500000000000000, -9.735942053221458872E-16, 7.950000000000000178 ) ) ;
#125828=EDGE_CURVE ( 'NONE', #18455, #127835, #37013, .T. ) ;
#125838=CARTESIAN_POINT ( 'NONE',  ( 41.41709685856477563, 3.054999999999998828, 5.291415217122922066 ) ) ;
#125855=ORIENTED_EDGE ( 'NONE', *, *, #57378, .F. ) ;
#125889=CARTESIAN_POINT ( 'NONE',  ( 71.37043019189812298, -3.055000000000001936, 5.291415217122918513 ) ) ;
#125891=CARTESIAN_POINT ( 'NONE',  ( 74.60002705046289861, 5.819803920172570422, 5.819803920172575751 ) ) ;
#125912=CARTESIAN_POINT ( 'NONE',  ( 101.8708603837962272, 6.884901960086289741, -3.974999999999993427 ) ) ;
#125927=CARTESIAN_POINT ( 'NONE',  ( 86.77126352523141861, 4.472830434245839371, 4.472830434245842035 ) ) ;
#125947=CARTESIAN_POINT ( 'NONE',  ( 85.75043019189810423, 3.055000000000002824, -5.291415217122919401 ) ) ;
#125959=CARTESIAN_POINT ( 'NONE',  ( 79.39126352523146579, -4.472830434245839371, -4.472830434245839371 ) ) ;
#125964=CARTESIAN_POINT ( 'NONE',  ( 33.62086038379622011, -6.884901960086286188, 3.974999999999997424 ) ) ;
#126001=ORIENTED_EDGE ( 'NONE', *, *, #59533, .F. ) ;
#126006=CARTESIAN_POINT ( 'NONE',  ( 70.00043019189810423, -3.055000000000002380, 5.291415217122920289 ) ) ;
#126010=( BOUNDED_CURVE ( )  B_SPLINE_CURVE ( 2, ( #19100, #62626, #49632, #140180, #63365, #93809, #106806, #82943, #7496, #107534, #51753, #127141, #22635 ),
 .UNSPECIFIED., .F., .T. ) 
 B_SPLINE_CURVE_WITH_KNOTS ( ( 3, 2, 2, 2, 2, 2, 3 ),
 ( 0.2333333333333333370, 0.2361111111111111049, 0.2388888888888889006, 0.2416666666666666685, 0.2444444444444444364, 0.2472222222222222321, 0.2500000000000000000 ),
 .UNSPECIFIED. ) 
 CURVE ( )  GEOMETRIC_REPRESENTATION_ITEM ( )  RATIONAL_B_SPLINE_CURVE ( ( 1.000000000000000000, 0.9659258262890683122, 1.000000000000000000, 0.9659258262890683122, 1.000000000000000000, 0.9659258262890683122, 1.000000000000000000, 0.9659258262890683122, 1.000000000000000000, 0.9659258262890683122, 1.000000000000000000, 0.9659258262890683122, 1.000000000000000000 ) ) 
 REPRESENTATION_ITEM ( '' )  );
#126015=CARTESIAN_POINT ( 'NONE',  ( 112.1462635252314328, -4.472830434245840259, 4.472830434245838482 ) ) ;
#126021=CARTESIAN_POINT ( 'NONE',  ( 35.37086038379622011, 6.884901960086289741, -3.974999999999993427 ) ) ;
#126050=CARTESIAN_POINT ( 'NONE',  ( 13.79677315470453181, -9.118197820415756993, -2.677214429515783145 ) ) ;
#126065=CARTESIAN_POINT ( 'NONE',  ( 74.06249999999998579, -5.819803920172573086, -5.819803920172573974 ) ) ;
#126082=CARTESIAN_POINT ( 'NONE',  ( 31.41209685856477662, 5.291415217122922066, -3.054999999999995275 ) ) ;
#126097=CARTESIAN_POINT ( 'NONE',  ( 90.54166666666665719, -3.975000000000002753, 6.884901960086286188 ) ) ;
#126108=CARTESIAN_POINT ( 'NONE',  ( 125.9664974496730281, 3.788224211676681552, -6.458789565855242110 ) ) ;
#126119=CARTESIAN_POINT ( 'NONE',  ( 112.7295968585647756, -6.110000000000000320, -1.637169565754161393 ) ) ;
#126127=CARTESIAN_POINT ( 'NONE',  ( 104.3287635252314658, 0.000000000000000000, -6.109999999999998543 ) ) ;
#126157=CARTESIAN_POINT ( 'NONE',  ( 0.000000000000000000, 0.000000000000000000, 0.000000000000000000 ) ) ;
#126164=CARTESIAN_POINT ( 'NONE',  ( 64.10002705046287019, 5.819803920172570422, 5.819803920172575751 ) ) ;
#126173=CARTESIAN_POINT ( 'NONE',  ( 34.76626352523143737, 4.472830434245838482, -4.472830434245837594 ) ) ;
#126205=CARTESIAN_POINT ( 'NONE',  ( 105.4954301918981230, 5.291415217122917625, 3.055000000000002380 ) ) ;
#126238=DIRECTION ( 'NONE',  ( 0.000000000000000000, 0.000000000000000000, 1.000000000000000000 ) ) ;
#126255=CARTESIAN_POINT ( 'NONE',  ( 124.8125000000000142, 5.819803920172571310, 5.819803920172575751 ) ) ;
#126266=CARTESIAN_POINT ( 'NONE',  ( 109.2295968585647614, -6.110000000000000320, -1.637169565754161393 ) ) ;
#126275=CARTESIAN_POINT ( 'NONE',  ( 40.18336038379622721, -2.130196079827426203, 7.949999999999997513 ) ) ;
#126277=CARTESIAN_POINT ( 'NONE',  ( 127.0000000000000000, -4.017717506652945580, -5.045834523320674059 ) ) ;
#126280=CARTESIAN_POINT ( 'NONE',  ( 35.41666666666666430, -6.884901960086287076, -3.975000000000000977 ) ) ;
#126290=CARTESIAN_POINT ( 'NONE',  ( 32.81293019189809002, -1.637169565754159617, -6.110000000000001208 ) ) ;
#126305=CARTESIAN_POINT ( 'NONE',  ( 49.34959685856478728, 6.109999999999996767, 1.637169565754163836 ) ) ;
#126335=CARTESIAN_POINT ( 'NONE',  ( 68.16209685856478018, -5.291415217122919401, 3.054999999999997939 ) ) ;
#126356=CARTESIAN_POINT ( 'NONE',  ( 30.60416666666665719, 2.130196079827422206, 7.950000000000001954 ) ) ;
#126374=ORIENTED_EDGE ( 'NONE', *, *, #129355, .T. ) ;
#126403=CARTESIAN_POINT ( 'NONE',  ( 51.39126352523145158, -4.472830434245839371, -4.472830434245839371 ) ) ;
#126425=CARTESIAN_POINT ( 'NONE',  ( 66.43336038379622721, 2.130196079827431532, -7.949999999999997513 ) ) ;
#126430=CARTESIAN_POINT ( 'NONE',  ( 61.37500000000000000, 7.950000000000000178, 1.460391307983218535E-15 ) ) ;
#126438=CARTESIAN_POINT ( 'NONE',  ( 127.0000000000000568, -4.172191364199829167, -4.786994800550450790 ) ) ;
#126440=CARTESIAN_POINT ( 'NONE',  ( 57.45876352523143993, 0.000000000000000000, -6.110000000000001208 ) ) ;
#126452=DIRECTION ( 'NONE',  ( 0.000000000000000000, 0.000000000000000000, 1.000000000000000000 ) ) ;
#126459=EDGE_CURVE ( 'NONE', #16751, #2806, #109695, .T. ) ;
#126490=CARTESIAN_POINT ( 'NONE',  ( 96.89126352523143737, -4.472830434245838482, -4.472830434245838482 ) ) ;
#126517=CARTESIAN_POINT ( 'NONE',  ( 45.79209685856476852, -5.291415217122921177, 3.054999999999999272 ) ) ;
#126564=CARTESIAN_POINT ( 'NONE',  ( 75.45376352523145158, -6.109999999999999432, -3.741295971395163529E-16 ) ) ;
#126585=CARTESIAN_POINT ( 'NONE',  ( 121.4125270504628986, -7.949999999999998401, -4.867971026610728450E-16 ) ) ;
#126588=CARTESIAN_POINT ( 'NONE',  ( 97.05836038379621300, -7.949999999999997513, -2.130196079827425759 ) ) ;
#126598=DIRECTION ( 'NONE',  ( 0.000000000000000000, 0.000000000000000000, 1.000000000000000000 ) ) ;
#126601=CARTESIAN_POINT ( 'NONE',  ( 46.30836038379622721, 7.949999999999996625, 2.130196079827431088 ) ) ;
#126603=CARTESIAN_POINT ( 'NONE',  ( 87.93793019189809002, -6.110000000000001208, 1.637169565754158951 ) ) ;
#126612=CARTESIAN_POINT ( 'NONE',  ( 117.1833603837962130, -2.130196079827426203, 7.949999999999996625 ) ) ;
#126613=DIRECTION ( 'NONE',  ( -1.000000000000000000, -0.000000000000000000, -0.000000000000000000 ) ) ;
#126625=CARTESIAN_POINT ( 'NONE',  ( 79.47959685856477563, 6.109999999999999432, 1.637169565754164280 ) ) ;
#126656=CARTESIAN_POINT ( 'NONE',  ( 25.08376352523143638, -6.110000000000001208, -3.741295971395164515E-16 ) ) ;
#126684=CARTESIAN_POINT ( 'NONE',  ( 73.64626352523140440, -4.472830434245840259, 4.472830434245838482 ) ) ;
#126691=CARTESIAN_POINT ( 'NONE',  ( 110.3962635252314328, 4.472830434245840259, -4.472830434245838482 ) ) ;
#126697=CARTESIAN_POINT ( 'NONE',  ( 34.78752705046288440, 0.000000000000000000, -7.949999999999998401 ) ) ;
#126715=AXIS2_PLACEMENT_3D ( 'NONE', #21313, #120591, #139557 ) ;
#126735=CARTESIAN_POINT ( 'NONE',  ( 73.04166666666667140, -3.975000000000002753, 6.884901960086286188 ) ) ;
#126755=CARTESIAN_POINT ( 'NONE',  ( 107.0208333333333144, 7.949999999999998401, 2.130196079827431532 ) ) ;
#126756=CARTESIAN_POINT ( 'NONE',  ( 123.6000270504628702, 5.819803920172570422, 5.819803920172574863 ) ) ;
#126772=CARTESIAN_POINT ( 'NONE',  ( 80.18749999999997158, -5.819803920172573086, 5.819803920172572198 ) ) ;
#126787=CARTESIAN_POINT ( 'NONE',  ( 127.0000000000000000, 1.864289179696898779, 6.174700466780991270 ) ) ;
#126798=CARTESIAN_POINT ( 'NONE',  ( 113.3129301918981042, -1.637169565754159617, -6.110000000000001208 ) ) ;
#126809=CARTESIAN_POINT ( 'NONE',  ( 101.8495968585647660, 6.109999999999996767, 1.637169565754163836 ) ) ;
#126835=DIRECTION ( 'NONE',  ( 0.000000000000000000, 0.000000000000000000, 1.000000000000000000 ) ) ;
#126846=CARTESIAN_POINT ( 'NONE',  ( 64.39169371712957002, 2.130196079827421762, 7.950000000000000178 ) ) ;
#126849=ORIENTED_EDGE ( 'NONE', *, *, #16859, .T. ) ;
#126856=CARTESIAN_POINT ( 'NONE',  ( 33.89126352523143737, -4.472830434245838482, -4.472830434245838482 ) ) ;
#126887=CARTESIAN_POINT ( 'NONE',  ( 102.8704301918981230, -3.055000000000001936, 5.291415217122918513 ) ) ;
#126944=CARTESIAN_POINT ( 'NONE',  ( 116.9375000000000142, 5.819803920172573974, -5.819803920172572198 ) ) ;
#126960=CARTESIAN_POINT ( 'NONE',  ( 114.7712635252314186, 4.472830434245839371, 4.472830434245842035 ) ) ;
#126969=CARTESIAN_POINT ( 'NONE',  ( 35.80836038379622721, 7.949999999999997513, 2.130196079827431088 ) ) ;
#126974=CARTESIAN_POINT ( 'NONE',  ( 35.99999999999999289, 0.000000000000000000, -7.950000000000000178 ) ) ;
#126986=CARTESIAN_POINT ( 'NONE',  ( 31.50043019189810423, -3.055000000000002380, 5.291415217122920289 ) ) ;
#126997=CARTESIAN_POINT ( 'NONE',  ( 55.56293019189809712, 1.637169565754157174, 6.110000000000002984 ) ) ;
#127003=CARTESIAN_POINT ( 'NONE',  ( 52.26626352523145158, 4.472830434245839371, -4.472830434245838482 ) ) ;
#127016=CARTESIAN_POINT ( 'NONE',  ( 44.85002705046287730, -5.819803920172573086, -5.819803920172573086 ) ) ;
#127037=CARTESIAN_POINT ( 'NONE',  ( 69.18293019189809456, -1.637169565754158951, -6.109999999999998543 ) ) ;
#127045=( BOUNDED_CURVE ( )  B_SPLINE_CURVE ( 2, ( #54890, #128851, #32416, #64323, #53437, #84650, #118692, #97651, #19383, #52711, #120084, #31000, #86799 ),
 .UNSPECIFIED., .F., .F. ) 
 B_SPLINE_CURVE_WITH_KNOTS ( ( 3, 2, 2, 2, 2, 2, 3 ),
 ( 0.3333333333333333148, 0.3361111111111111382, 0.3388888888888889062, 0.3416666666666666741, 0.3444444444444444975, 0.3472222222222222654, 0.3500000000000000333 ),
 .UNSPECIFIED. ) 
 CURVE ( )  GEOMETRIC_REPRESENTATION_ITEM ( )  RATIONAL_B_SPLINE_CURVE ( ( 1.000000000000000000, 0.9659258262890683122, 1.000000000000000000, 0.9659258262890683122, 1.000000000000000000, 0.9659258262890683122, 1.000000000000000000, 0.9659258262890683122, 1.000000000000000000, 0.9659258262890683122, 1.000000000000000000, 0.9659258262890676461, 1.000000000000000666 ) ) 
 REPRESENTATION_ITEM ( '' )  );
#127089=FACE_OUTER_BOUND ( 'NONE', #68462, .T. ) ;
#127114=CARTESIAN_POINT ( 'NONE',  ( 50.95376352523145158, -6.109999999999999432, -3.741295971395163529E-16 ) ) ;
#127141=CARTESIAN_POINT ( 'NONE',  ( 103.1833603837962130, -2.130196079827426203, 7.949999999999996625 ) ) ;
#127142=CARTESIAN_POINT ( 'NONE',  ( 61.91252705046289151, -7.949999999999998401, -4.867971026610728450E-16 ) ) ;
#127146=CARTESIAN_POINT ( 'NONE',  ( 64.72916666666667140, 7.950000000000001954, -2.130196079827421762 ) ) ;
#127155=CARTESIAN_POINT ( 'NONE',  ( 60.22959685856476142, -6.110000000000000320, -1.637169565754161393 ) ) ;
#127189=CARTESIAN_POINT ( 'NONE',  ( 64.00000000000000000, 0.000000000000000000, -7.950000000000000178 ) ) ;
#127208=CARTESIAN_POINT ( 'NONE',  ( 90.76626352523145158, 4.472830434245838482, -4.472830434245837594 ) ) ;
#127233=CARTESIAN_POINT ( 'NONE',  ( 47.10459685856477563, 1.637169565754164946, -6.109999999999999432 ) ) ;
#127269=CARTESIAN_POINT ( 'NONE',  ( 67.06249999999998579, -5.819803920172573086, -5.819803920172573974 ) ) ;
#127290=CARTESIAN_POINT ( 'NONE',  ( 77.64126352523146579, 4.472830434245837594, 4.472830434245841147 ) ) ;
#127315=CARTESIAN_POINT ( 'NONE',  ( 89.47502705046288440, -5.819803920172572198, 5.819803920172572198 ) ) ;
#127316=CARTESIAN_POINT ( 'NONE',  ( 71.43749999999998579, 5.819803920172574863, -5.819803920172573086 ) ) ;
#127326=CARTESIAN_POINT ( 'NONE',  ( 46.01669371712956291, 7.950000000000000178, -2.130196079827421318 ) ) ;
#127329=CARTESIAN_POINT ( 'NONE',  ( 87.20876352523143282, -7.482591942790329030E-16, 6.110000000000001208 ) ) ;
#127335=EDGE_LOOP ( 'NONE', ( #68745, #64928, #98335, #128012 ) ) ;
#127341=DIRECTION ( 'NONE',  ( 1.000000000000000000, 0.000000000000000000, 0.000000000000000000 ) ) ;
#127355=CARTESIAN_POINT ( 'NONE',  ( 78.31293019189810423, -1.637169565754159617, -6.110000000000001208 ) ) ;
#127370=AXIS2_PLACEMENT_3D ( 'NONE', #13024, #12322, #47858 ) ;
#127409=CARTESIAN_POINT ( 'NONE',  ( 72.04209685856477563, 5.291415217122923842, -3.054999999999996163 ) ) ;
#127415=CARTESIAN_POINT ( 'NONE',  ( 105.5837635252314328, -6.110000000000001208, -3.741295971395164515E-16 ) ) ;
#127432=CARTESIAN_POINT ( 'NONE',  ( 114.7041937171295558, -6.884901960086285300, -3.975000000000000089 ) ) ;
#127450=CARTESIAN_POINT ( 'NONE',  ( 10.32500000000000107, -8.432637487761466488, 4.375000000000001776 ) ) ;
#127488=CARTESIAN_POINT ( 'NONE',  ( 117.4750270504628702, -5.819803920172572198, 5.819803920172572198 ) ) ;
#127506=CARTESIAN_POINT ( 'NONE',  ( 81.79166666666667140, 3.975000000000003642, -6.884901960086285300 ) ) ;
#127513=CARTESIAN_POINT ( 'NONE',  ( 30.12086038379621655, -6.884901960086286188, 3.974999999999997424 ) ) ;
#127531=CARTESIAN_POINT ( 'NONE',  ( 98.87543019189810423, -5.291415217122920289, -3.055000000000001492 ) ) ;
#127542=CARTESIAN_POINT ( 'NONE',  ( 103.3079301918981088, -6.109999999999998543, 1.637169565754158063 ) ) ;
#127571=CARTESIAN_POINT ( 'NONE',  ( 113.5162635252314516, -4.472830434245838482, 4.472830434245838482 ) ) ;
#127600=CARTESIAN_POINT ( 'NONE',  ( 31.41209685856477662, 5.291415217122921177, -3.054999999999994831 ) ) ;
#127638=CARTESIAN_POINT ( 'NONE',  ( 103.8912635252314516, -4.472830434245839371, -4.472830434245839371 ) ) ;
#127687=CARTESIAN_POINT ( 'NONE',  ( 26.48225813788241112, 5.499261314031191006, -3.174999999999997158 ) ) ;
#127694=CARTESIAN_POINT ( 'NONE',  ( 114.8958333333333286, -2.130196079827427091, 7.949999999999999289 ) ) ;
#127698=AXIS2_PLACEMENT_3D ( 'NONE', #65420, #29885, #42942 ) ;
#127707=CARTESIAN_POINT ( 'NONE',  ( 111.7087635252314470, -7.482591942790329030E-16, 6.110000000000001208 ) ) ;
#127717=CARTESIAN_POINT ( 'NONE',  ( 37.26669371712955581, -7.949999999999999289, 2.130196079827424427 ) ) ;
#127724=CARTESIAN_POINT ( 'NONE',  ( 26.81249999999998934, 5.819803920172571310, 5.819803920172575751 ) ) ;
#127734=CARTESIAN_POINT ( 'NONE',  ( 29.31293019189811133, -1.637169565754159617, -6.110000000000001208 ) ) ;
#127742=CARTESIAN_POINT ( 'NONE',  ( 63.12500000000000000, -7.950000000000000178, -4.867971026610729436E-16 ) ) ;
#127744=CARTESIAN_POINT ( 'NONE',  ( 50.60459685856477563, 1.637169565754164946, -6.109999999999999432 ) ) ;
#127751=CARTESIAN_POINT ( 'NONE',  ( 46.72459685856476597, -1.637169565754160949, 6.109999999999997655 ) ) ;
#127753=CARTESIAN_POINT ( 'NONE',  ( 123.5000000000000000, 0.000000000000000000, -7.950000000000000178 ) ) ;
#127786=CARTESIAN_POINT ( 'NONE',  ( 65.68293019189810877, -1.637169565754158951, -6.109999999999998543 ) ) ;
#127793=EDGE_CURVE ( 'NONE', #2756, #8484, #118905, .T. ) ;
#127812=CARTESIAN_POINT ( 'NONE',  ( 55.20419371712956291, -6.884901960086285300, -3.975000000000000089 ) ) ;
#127822=CARTESIAN_POINT ( 'NONE',  ( 128.8287635252314658, 0.000000000000000000, -6.109999999999999432 ) ) ;
#127835=VERTEX_POINT ( 'NONE', #29746 ) ;
#127848=CARTESIAN_POINT ( 'NONE',  ( 0.000000000000000000, 0.000000000000000000, 0.000000000000000000 ) ) ;
#127869=CARTESIAN_POINT ( 'NONE',  ( 44.24543019189810877, -5.291415217122919401, -3.055000000000000604 ) ) ;
#127873=ORIENTED_EDGE ( 'NONE', *, *, #87012, .F. ) ;
#127880=AXIS2_PLACEMENT_3D ( 'NONE', #8925, #141658, #53195 ) ;
#127892=CARTESIAN_POINT ( 'NONE',  ( 67.30836038379622721, 7.949999999999997513, 2.130196079827431088 ) ) ;
#127896=CARTESIAN_POINT ( 'NONE',  ( 60.35416666666667140, -2.130196079827425315, -7.950000000000001066 ) ) ;
#127903=CARTESIAN_POINT ( 'NONE',  ( 34.24999999999998579, -9.735942053221458872E-16, 7.950000000000000178 ) ) ;
#127906=CARTESIAN_POINT ( 'NONE',  ( 59.35459685856476142, -1.637169565754161615, 6.110000000000000320 ) ) ;
#127918=CARTESIAN_POINT ( 'NONE',  ( 101.1416937171295558, -2.130196079827424871, -7.949999999999998401 ) ) ;
#127935=CYLINDRICAL_SURFACE ( 'NONE', #69956, 7.950000000000000178 ) ;
#127958=CARTESIAN_POINT ( 'NONE',  ( 95.28709685856479439, 3.054999999999997495, 5.291415217122919401 ) ) ;
#127991=CARTESIAN_POINT ( 'NONE',  ( 47.97959685856477563, 6.109999999999999432, 1.637169565754164280 ) ) ;
#128006=FACE_OUTER_BOUND ( 'NONE', #95481, .T. ) ;
#128012=ORIENTED_EDGE ( 'NONE', *, *, #31583, .F. ) ;
#128041=CARTESIAN_POINT ( 'NONE',  ( 73.99543019189810877, 5.291415217122917625, 3.055000000000002380 ) ) ;
#128063=CARTESIAN_POINT ( 'NONE',  ( 89.62086038379622721, -6.884901960086286188, 3.974999999999997424 ) ) ;
#128072=CARTESIAN_POINT ( 'NONE',  ( 0.000000000000000000, 0.000000000000000000, 0.000000000000000000 ) ) ;
#128075=CARTESIAN_POINT ( 'NONE',  ( 45.43336038379621300, 2.130196079827431532, -7.949999999999996625 ) ) ;
#128078=CARTESIAN_POINT ( 'NONE',  ( 82.25043019189810423, 3.055000000000002824, -5.291415217122919401 ) ) ;
#128098=CARTESIAN_POINT ( 'NONE',  ( 70.87543019189810423, -5.291415217122920289, -3.055000000000001492 ) ) ;
#128126=VERTEX_POINT ( 'NONE', #79016 ) ;
#128154=CARTESIAN_POINT ( 'NONE',  ( 73.93793019189809002, -6.110000000000001208, 1.637169565754158951 ) ) ;
#128160=CARTESIAN_POINT ( 'NONE',  ( 110.5420968585647756, 5.291415217122923842, -3.054999999999996163 ) ) ;
#128177=CARTESIAN_POINT ( 'NONE',  ( 114.2666937171295700, -7.949999999999998401, 2.130196079827423983 ) ) ;
#128191=CARTESIAN_POINT ( 'NONE',  ( 14.69991882521100557, -9.499962616874643828, 0.2903383370780639461 ) ) ;
#128221=CARTESIAN_POINT ( 'NONE',  ( 123.7458603837962272, 3.974999999999996980, 6.884901960086287964 ) ) ;
#128236=CARTESIAN_POINT ( 'NONE',  ( 80.47916666666664298, -7.950000000000001066, 2.130196079827424427 ) ) ;
#128243=CARTESIAN_POINT ( 'NONE',  ( 30.85002705046288085, -5.819803920172573086, -5.819803920172573086 ) ) ;
#128261=CARTESIAN_POINT ( 'NONE',  ( 101.2087635252314470, -7.482591942790329030E-16, 6.110000000000001208 ) ) ;
#128267=ADVANCED_FACE ( 'NONE', ( #77420 ), #88993, .T. ) ;
#128270=CIRCLE ( 'NONE', #88855, 6.350000000000001421 ) ;
#128271=CARTESIAN_POINT ( 'NONE',  ( 96.16209685856478018, -5.291415217122919401, 3.054999999999997939 ) ) ;
#128286=EDGE_CURVE ( 'NONE', #87171, #29769, #36461, .T. ) ;
#128298=CARTESIAN_POINT ( 'NONE',  ( 117.0162635252314374, -4.472830434245838482, 4.472830434245838482 ) ) ;
#128324=CARTESIAN_POINT ( 'NONE',  ( 29.07876352523144803, -7.482591942790325086E-16, 6.109999999999998543 ) ) ;
#128360=CARTESIAN_POINT ( 'NONE',  ( 104.4745968585647802, 1.637169565754164280, -6.109999999999997655 ) ) ;
#128396=CARTESIAN_POINT ( 'NONE',  ( 47.37500000000000000, 7.950000000000000178, 1.460391307983218535E-15 ) ) ;
#128402=ORIENTED_EDGE ( 'NONE', *, *, #48779, .F. ) ;
#128405=CARTESIAN_POINT ( 'NONE',  ( 114.4583333333333286, 3.974999999999997424, 6.884901960086288852 ) ) ;
#128409=ORIENTED_EDGE ( 'NONE', *, *, #70196, .T. ) ;
#128417=CARTESIAN_POINT ( 'NONE',  ( 100.3337635252314328, 6.110000000000001208, 1.122388791418549305E-15 ) ) ;
#128428=CARTESIAN_POINT ( 'NONE',  ( 39.74586038379622721, 3.974999999999996980, 6.884901960086287964 ) ) ;
#128435=CARTESIAN_POINT ( 'NONE',  ( 126.8754301918981184, -5.291415217122920289, -3.055000000000001492 ) ) ;
#128446=CARTESIAN_POINT ( 'NONE',  ( 125.0370968585647944, -3.054999999999998828, -5.291415217122919401 ) ) ;
#128455=CARTESIAN_POINT ( 'NONE',  ( 47.39626352523143282, 4.472830434245840259, -4.472830434245839371 ) ) ;
#128462=CARTESIAN_POINT ( 'NONE',  ( 51.82876352523144448, 0.000000000000000000, -6.109999999999998543 ) ) ;
#128473=CARTESIAN_POINT ( 'NONE',  ( 60.60002705046289861, 5.819803920172570422, 5.819803920172575751 ) ) ;
#128476=CARTESIAN_POINT ( 'NONE',  ( 43.68336038379622011, -2.130196079827426203, 7.949999999999996625 ) ) ;
#128492=CARTESIAN_POINT ( 'NONE',  ( 60.72459685856477307, -1.637169565754160949, 6.109999999999997655 ) ) ;
#128494=( BOUNDED_CURVE ( )  B_SPLINE_CURVE ( 2, ( #40958, #130850, #85161, #20611, #130120, #76461, #107626, #52536, #120629, #129375, #57569, #135138, #89449 ),
 .UNSPECIFIED., .F., .T. ) 
 B_SPLINE_CURVE_WITH_KNOTS ( ( 3, 2, 2, 2, 2, 2, 3 ),
 ( 0.7666666666666666075, 0.7694444444444443754, 0.7722222222222221433, 0.7749999999999999112, 0.7777777777777777901, 0.7805555555555555580, 0.7833333333333333259 ),
 .UNSPECIFIED. ) 
 CURVE ( )  GEOMETRIC_REPRESENTATION_ITEM ( )  RATIONAL_B_SPLINE_CURVE ( ( 1.000000000000001332, 0.9659258262890669799, 1.000000000000000000, 0.9659258262890683122, 1.000000000000000000, 0.9659258262890683122, 1.000000000000000000, 0.9659258262890683122, 1.000000000000000000, 0.9659258262890683122, 1.000000000000000000, 0.9659258262890683122, 1.000000000000000000 ) ) 
 REPRESENTATION_ITEM ( '' )  );
#128502=CARTESIAN_POINT ( 'NONE',  ( 35.99999999999999289, 0.000000000000000000, -7.950000000000000178 ) ) ;
#128561=CARTESIAN_POINT ( 'NONE',  ( 48.91209685856478018, 5.291415217122922066, -3.054999999999995275 ) ) ;
#128572=CARTESIAN_POINT ( 'NONE',  ( 83.10416666666667140, 2.130196079827498146, 7.949999999999958433 ) ) ;
#128573=CARTESIAN_POINT ( 'NONE',  ( 127.1670968585647756, -3.055000000000000160, -5.291415217122921177 ) ) ;
#128584=CARTESIAN_POINT ( 'NONE',  ( 64.68336038379622721, -2.130196079827426203, 7.949999999999997513 ) ) ;
#128590=CARTESIAN_POINT ( 'NONE',  ( 55.24999999999999289, -9.735942053221458872E-16, 7.950000000000000178 ) ) ;
#128600=CARTESIAN_POINT ( 'NONE',  ( 61.25043019189810423, 3.055000000000002824, -5.291415217122919401 ) ) ;
#128604=ORIENTED_EDGE ( 'NONE', *, *, #116290, .T. ) ;
#128625=CARTESIAN_POINT ( 'NONE',  ( 72.39126352523145158, -4.472830434245839371, -4.472830434245839371 ) ) ;
#128652=CARTESIAN_POINT ( 'NONE',  ( 82.89126352523143737, -4.472830434245838482, -4.472830434245838482 ) ) ;
#128677=CARTESIAN_POINT ( 'NONE',  ( 35.00043019189810423, -3.055000000000002380, 5.291415217122920289 ) ) ;
#128706=VERTEX_POINT ( 'NONE', #11201 ) ;
#128708=ORIENTED_EDGE ( 'NONE', *, *, #138528, .F. ) ;
#128715=CARTESIAN_POINT ( 'NONE',  ( 96.95833333333334281, 3.974999999999997424, 6.884901960086288852 ) ) ;
#128727=CARTESIAN_POINT ( 'NONE',  ( 74.72459685856476597, -1.637169565754161171, 6.109999999999998543 ) ) ;
#128747=CARTESIAN_POINT ( 'NONE',  ( 98.51669371712955581, 7.950000000000001066, -2.130196079827421318 ) ) ;
#128763=VERTEX_POINT ( 'NONE', #124286 ) ;
#128764=CARTESIAN_POINT ( 'NONE',  ( 87.35459685856476142, -1.637169565754161615, 6.110000000000000320 ) ) ;
#128783=CARTESIAN_POINT ( 'NONE',  ( 74.22959685856476142, -6.110000000000000320, -1.637169565754161393 ) ) ;
#128826=CARTESIAN_POINT ( 'NONE',  ( 27.00000000000001066, -6.477409876647271858, -3.272594246810044627 ) ) ;
#128838=CARTESIAN_POINT ( 'NONE',  ( 71.89626352523143282, 4.472830434245840259, -4.472830434245838482 ) ) ;
#128844=CARTESIAN_POINT ( 'NONE',  ( 108.6462635252314186, -4.472830434245840259, 4.472830434245838482 ) ) ;
#128851=CARTESIAN_POINT ( 'NONE',  ( 91.85416666666667140, -2.130196079827425759, -7.950000000000000178 ) ) ;
#128887=CARTESIAN_POINT ( 'NONE',  ( 33.83376352523143282, 6.110000000000001208, 1.122388791418549305E-15 ) ) ;
#128909=CARTESIAN_POINT ( 'NONE',  ( 121.4125270504628986, -7.949999999999998401, -4.867971026610728450E-16 ) ) ;
#128928=CARTESIAN_POINT ( 'NONE',  ( 86.31249999999997158, 5.819803920172571310, 5.819803920172575751 ) ) ;
#128931=EDGE_CURVE ( 'NONE', #125049, #122112, #103928, .T. ) ;
#128945=CARTESIAN_POINT ( 'NONE',  ( 41.10416666666666430, 2.130196079827422206, 7.950000000000001954 ) ) ;
#128955=CARTESIAN_POINT ( 'NONE',  ( 103.3962635252314328, 4.472830434245840259, -4.472830434245839371 ) ) ;
#128962=CARTESIAN_POINT ( 'NONE',  ( 75.22916666666667140, 7.950000000000001954, -2.130196079827421762 ) ) ;
#128964=CARTESIAN_POINT ( 'NONE',  ( 96.30793019189810877, -6.109999999999998543, 1.637169565754158063 ) ) ;
#129029=EDGE_LOOP ( 'NONE', ( #119421, #64325, #137247, #83236 ) ) ;
#129046=CARTESIAN_POINT ( 'NONE',  ( 88.72459685856478018, -1.637169565754161171, 6.109999999999998543 ) ) ;
#129058=ORIENTED_EDGE ( 'NONE', *, *, #96974, .T. ) ;
#129082=CARTESIAN_POINT ( 'NONE',  ( 32.35416666666665719, -2.130196079827501698, -7.949999999999956657 ) ) ;
#129096=CARTESIAN_POINT ( 'NONE',  ( 107.0208333333333002, 7.949999999999999289, 2.130196079827431532 ) ) ;
#129109=CARTESIAN_POINT ( 'NONE',  ( 105.8754301918981042, -5.291415217122920289, -3.055000000000001492 ) ) ;
#129127=CARTESIAN_POINT ( 'NONE',  ( 125.2712635252314470, 4.472830434245839371, 4.472830434245842035 ) ) ;
#129137=CARTESIAN_POINT ( 'NONE',  ( 122.2662635252314374, 4.472830434245839371, -4.472830434245838482 ) ) ;
#129147=CARTESIAN_POINT ( 'NONE',  ( 41.56293019189811133, 1.637169565754157174, 6.110000000000002984 ) ) ;
#129156=CARTESIAN_POINT ( 'NONE',  ( 43.95376352523145158, -6.109999999999998543, -3.741295971395162543E-16 ) ) ;
#129167=VERTEX_POINT ( 'NONE', #76339 ) ;
#129176=CARTESIAN_POINT ( 'NONE',  ( 56.34959685856478018, 6.109999999999996767, 1.637169565754163836 ) ) ;
#129199=CARTESIAN_POINT ( 'NONE',  ( 54.62086038379622721, -6.884901960086286188, 3.974999999999997424 ) ) ;
#129211=CARTESIAN_POINT ( 'NONE',  ( 119.4954301918981230, 5.291415217122917625, 3.055000000000002380 ) ) ;
#129251=CARTESIAN_POINT ( 'NONE',  ( 35.78709685856478018, 3.054999999999997939, 5.291415217122920289 ) ) ;
#129277=CARTESIAN_POINT ( 'NONE',  ( 56.37086038379622721, 6.884901960086289741, -3.974999999999993427 ) ) ;
#129282=CARTESIAN_POINT ( 'NONE',  ( 54.81249999999998579, 5.819803920172571310, 5.819803920172575751 ) ) ;
#129290=CARTESIAN_POINT ( 'NONE',  ( 47.68793019189809712, 6.110000000000002984, -1.637169565754156730 ) ) ;
#129313=VECTOR ( 'NONE', #101848, 1000.000000000000000 ) ;
#129318=CARTESIAN_POINT ( 'NONE',  ( 62.91209685856477307, 5.291415217122921177, -3.054999999999994831 ) ) ;
#129344=CARTESIAN_POINT ( 'NONE',  ( 62.25000000000000000, -9.735942053221458872E-16, 7.950000000000000178 ) ) ;
#129348=ORIENTED_EDGE ( 'NONE', *, *, #54368, .F. ) ;
#129350=CARTESIAN_POINT ( 'NONE',  ( 81.87043019189812298, -3.055000000000001492, 5.291415217122917625 ) ) ;
#129355=EDGE_CURVE ( 'NONE', #13817, #1460, #109114, .T. ) ;
#129362=CARTESIAN_POINT ( 'NONE',  ( 0.000000000000000000, 0.000000000000000000, 0.000000000000000000 ) ) ;
#129366=VERTEX_POINT ( 'NONE', #16585 ) ;
#129373=CARTESIAN_POINT ( 'NONE',  ( 37.47959685856476142, 6.109999999999999432, 1.637169565754164280 ) ) ;
#129375=CARTESIAN_POINT ( 'NONE',  ( 45.18749999999998579, -5.819803920172573974, 5.819803920172573086 ) ) ;
#129423=CARTESIAN_POINT ( 'NONE',  ( 94.28752705046289861, 0.000000000000000000, -7.949999999999998401 ) ) ;
#129429=CARTESIAN_POINT ( 'NONE',  ( 67.72459685856478018, -1.637169565754161171, 6.109999999999998543 ) ) ;
#129438=ORIENTED_EDGE ( 'NONE', *, *, #4728, .F. ) ;
#129445=AXIS2_PLACEMENT_3D ( 'NONE', #63670, #107829, #34588 ) ;
#129457=CARTESIAN_POINT ( 'NONE',  ( 96.47502705046288440, -5.819803920172572198, 5.819803920172572198 ) ) ;
#129462=CARTESIAN_POINT ( 'NONE',  ( 0.000000000000000000, 9.735942053221458872E-16, -7.950000000000000178 ) ) ;
#129471=CARTESIAN_POINT ( 'NONE',  ( 70.87543019189810423, -5.291415217122920289, -3.055000000000001492 ) ) ;
#129475=CARTESIAN_POINT ( 'NONE',  ( 160.0000000000000000, 6.349999999999997868, 0.000000000000000000 ) ) ;
#129487=CARTESIAN_POINT ( 'NONE',  ( 75.25043019189811844, 3.055000000000002824, -5.291415217122919401 ) ) ;
#129538=ORIENTED_EDGE ( 'NONE', *, *, #71564, .F. ) ;
#129543=CARTESIAN_POINT ( 'NONE',  ( 65.18793019189811844, 6.110000000000002984, -1.637169565754156730 ) ) ;
#129546=ORIENTED_EDGE ( 'NONE', *, *, #54549, .T. ) ;
#129552=CARTESIAN_POINT ( 'NONE',  ( 95.66709685856477563, -3.055000000000000160, -5.291415217122921177 ) ) ;
#129592=CARTESIAN_POINT ( 'NONE',  ( 33.10459685856476852, 1.637169565754164946, -6.109999999999999432 ) ) ;
#129618=CARTESIAN_POINT ( 'NONE',  ( 119.2250270504628986, 5.819803920172573086, -5.819803920172572198 ) ) ;
#129619=CARTESIAN_POINT ( 'NONE',  ( 50.24586038379622011, 3.974999999999996980, 6.884901960086287964 ) ) ;
#129633=CARTESIAN_POINT ( 'NONE',  ( 27.00000000000000355, 0.000000000000000000, 0.000000000000000000 ) ) ;
#129637=DIRECTION ( 'NONE',  ( -1.000000000000000000, -0.000000000000000000, -0.000000000000000000 ) ) ;
#129659=CARTESIAN_POINT ( 'NONE',  ( 102.9587635252314470, 0.000000000000000000, -6.110000000000001208 ) ) ;
#129666=CARTESIAN_POINT ( 'NONE',  ( 74.50000000000000000, 0.000000000000000000, -7.950000000000000178 ) ) ;
#129669=CARTESIAN_POINT ( 'NONE',  ( 99.07876352523145158, -7.482591942790325086E-16, 6.109999999999998543 ) ) ;
#129721=CARTESIAN_POINT ( 'NONE',  ( 26.59959685856477307, -6.109999999999997655, -1.637169565754160283 ) ) ;
#129725=CARTESIAN_POINT ( 'NONE',  ( 127.3129301918981042, -1.637169565754159617, -6.110000000000001208 ) ) ;
#129731=EDGE_CURVE ( 'NONE', #102139, #91497, #96534, .T. ) ;
#129762=CARTESIAN_POINT ( 'NONE',  ( 92.80793019189812298, -6.109999999999999432, 1.637169565754158507 ) ) ;
#129779=DIRECTION ( 'NONE',  ( 0.000000000000000000, 0.000000000000000000, 1.000000000000000000 ) ) ;
#129791=AXIS2_PLACEMENT_3D ( 'NONE', #13360, #111251, #90972 ) ;
#129802=CARTESIAN_POINT ( 'NONE',  ( 46.79166666666666430, 3.975000000000003642, -6.884901960086285300 ) ) ;
#129814=CARTESIAN_POINT ( 'NONE',  ( 108.7708333333333286, -7.949999999999999289, -2.130196079827426203 ) ) ;
#129821=CARTESIAN_POINT ( 'NONE',  ( 89.08333333333332860, 6.884901960086290629, -3.974999999999994316 ) ) ;
#129832=CARTESIAN_POINT ( 'NONE',  ( 103.3962635252314328, 4.472830434245840259, -4.472830434245839371 ) ) ;
#129846=CARTESIAN_POINT ( 'NONE',  ( 31.47916666666665364, -7.950000000000001066, 2.130196079827424427 ) ) ;
#129848=VECTOR ( 'NONE', #79113, 1000.000000000000000 ) ;
#129857=CARTESIAN_POINT ( 'NONE',  ( 126.6412635252314516, 4.472830434245836706, 4.472830434245840259 ) ) ;
#129869=CARTESIAN_POINT ( 'NONE',  ( 43.75043019189810423, 3.055000000000002824, -5.291415217122919401 ) ) ;
#129878=CARTESIAN_POINT ( 'NONE',  ( 41.18293019189811588, -1.637169565754158951, -6.109999999999998543 ) ) ;
#129905=CARTESIAN_POINT ( 'NONE',  ( 59.99543019189810877, 5.291415217122916737, 3.055000000000001936 ) ) ;
#129917=AXIS2_PLACEMENT_3D ( 'NONE', #113644, #34681, #47040 ) ;
#129948=CARTESIAN_POINT ( 'NONE',  ( 120.9537635252314658, -6.109999999999999432, -3.741295971395163529E-16 ) ) ;
#129958=CARTESIAN_POINT ( 'NONE',  ( 1.500000000000000000, 0.000000000000000000, 0.000000000000000000 ) ) ;
#129987=CARTESIAN_POINT ( 'NONE',  ( 34.18293019189809456, -1.637169565754159173, -6.109999999999999432 ) ) ;
#129991=ORIENTED_EDGE ( 'NONE', *, *, #111905, .T. ) ;
#130001=CARTESIAN_POINT ( 'NONE',  ( 81.49999999999998579, 0.000000000000000000, -7.950000000000000178 ) ) ;
#130012=CARTESIAN_POINT ( 'NONE',  ( 54.47502705046288440, -5.819803920172572198, 5.819803920172572198 ) ) ;
#130016=CARTESIAN_POINT ( 'NONE',  ( 57.72916666666665719, 7.950000000000001954, -2.130196079827421762 ) ) ;
#130027=CARTESIAN_POINT ( 'NONE',  ( 45.06293019189811844, 1.637169565754157174, 6.110000000000002984 ) ) ;
#130037=DIRECTION ( 'NONE',  ( -1.000000000000000000, -0.000000000000000000, -0.000000000000000000 ) ) ;
#130047=CARTESIAN_POINT ( 'NONE',  ( 84.43793019189810423, -6.110000000000001208, 1.637169565754158951 ) ) ;
#130057=CARTESIAN_POINT ( 'NONE',  ( 69.18293019189809456, -1.637169565754158951, -6.109999999999998543 ) ) ;
#130088=CARTESIAN_POINT ( 'NONE',  ( 81.28709685856478018, 3.054999999999997495, 5.291415217122919401 ) ) ;
#130110=CARTESIAN_POINT ( 'NONE',  ( 123.8916937171299253, 2.130196079822641142, 7.950000000002760636 ) ) ;
#130117=CARTESIAN_POINT ( 'NONE',  ( 35.29209685856476852, -5.291415217122921177, 3.054999999999999272 ) ) ;
#130120=CARTESIAN_POINT ( 'NONE',  ( 45.91666666666666430, -6.884901960086287076, -3.975000000000000977 ) ) ;
#130157=EDGE_CURVE ( 'NONE', #83079, #96308, #30965, .T. ) ;
#130159=EDGE_CURVE ( 'NONE', #77789, #66568, #66108, .T. ) ;
#130167=CARTESIAN_POINT ( 'NONE',  ( 113.0000000000000000, 0.000000000000000000, -7.950000000000000178 ) ) ;
#130171=CARTESIAN_POINT ( 'NONE',  ( 67.28709685856478018, 3.054999999999997939, 5.291415217122920289 ) ) ;
#130181=ORIENTED_EDGE ( 'NONE', *, *, #95323, .F. ) ;
#130189=CARTESIAN_POINT ( 'NONE',  ( 106.5833333333333286, 6.884901960086290629, -3.974999999999994316 ) ) ;
#130199=CARTESIAN_POINT ( 'NONE',  ( 80.72502705046289861, 5.819803920172573086, -5.819803920172572198 ) ) ;
#130213=CARTESIAN_POINT ( 'NONE',  ( 72.77126352523144703, 4.472830434245839371, 4.472830434245842035 ) ) ;
#130231=CARTESIAN_POINT ( 'NONE',  ( 59.33333333333333570, -6.884901960086287964, 3.974999999999998312 ) ) ;
#130235=CARTESIAN_POINT ( 'NONE',  ( 61.25043019189810423, 3.055000000000002824, -5.291415217122919401 ) ) ;
#130238=DIRECTION ( 'NONE',  ( 0.000000000000000000, 0.000000000000000000, 1.000000000000000000 ) ) ;
#130283=CARTESIAN_POINT ( 'NONE',  ( 58.55836038379621300, -7.949999999999996625, -2.130196079827426203 ) ) ;
#130298=CARTESIAN_POINT ( 'NONE',  ( 66.20876352523144703, -7.482591942790329030E-16, 6.110000000000001208 ) ) ;
#130302=CARTESIAN_POINT ( 'NONE',  ( 97.70876352523144703, -7.482591942790329030E-16, 6.110000000000001208 ) ) ;
#130318=CARTESIAN_POINT ( 'NONE',  ( 120.2245968585647944, -1.637169565754160949, 6.109999999999997655 ) ) ;
#130330=CARTESIAN_POINT ( 'NONE',  ( 12.27285362782770761, -8.650847453065608761, -3.927786684156754582 ) ) ;
#130342=CARTESIAN_POINT ( 'NONE',  ( 27.56293019189811133, 1.637169565754157174, 6.110000000000002984 ) ) ;
#130363=CARTESIAN_POINT ( 'NONE',  ( 94.28752705046289861, 0.000000000000000000, -7.949999999999998401 ) ) ;
#130364=CARTESIAN_POINT ( 'NONE',  ( 109.4541937171295558, 6.884901960086283523, 3.975000000000002753 ) ) ;
#130368=FACE_BOUND ( 'NONE', #71768, .T. ) ;
#130382=CARTESIAN_POINT ( 'NONE',  ( 91.51669371712954160, 7.950000000000000178, -2.130196079827421318 ) ) ;
#130405=CARTESIAN_POINT ( 'NONE',  ( 105.2920968585647756, -5.291415217122921177, 3.054999999999999272 ) ) ;
#130416=CARTESIAN_POINT ( 'NONE',  ( 98.20376352523145158, 6.109999999999998543, 1.122388791418548911E-15 ) ) ;
#130421=CARTESIAN_POINT ( 'NONE',  ( 115.4791666666666572, -7.950000000000000178, 2.130196079827424427 ) ) ;
#130437=EDGE_LOOP ( 'NONE', ( #97879, #75664, #142770, #84212 ) ) ;
#130454=ORIENTED_EDGE ( 'NONE', *, *, #77253, .T. ) ;
#130464=ORIENTED_EDGE ( 'NONE', *, *, #109273, .F. ) ;
#130468=CARTESIAN_POINT ( 'NONE',  ( 29.80793019189811588, -6.109999999999998543, 1.637169565754158507 ) ) ;
#130469=DIRECTION ( 'NONE',  ( -1.000000000000000000, -0.000000000000000000, -0.000000000000000000 ) ) ;
#130506=CARTESIAN_POINT ( 'NONE',  ( 96.01626352523143737, -4.472830434245839371, 4.472830434245839371 ) ) ;
#130507=CARTESIAN_POINT ( 'NONE',  ( 9.174743583335013497, -8.505992269982375120, -4.231105565351911402 ) ) ;
#130529=ORIENTED_EDGE ( 'NONE', *, *, #74032, .T. ) ;
#130537=CARTESIAN_POINT ( 'NONE',  ( 27.12608002228219206, 1.810106405120792683, 7.950000000000001954 ) ) ;
#130552=CARTESIAN_POINT ( 'NONE',  ( 115.4791666666666572, -7.950000000000001066, 2.130196079827424427 ) ) ;
#130565=CARTESIAN_POINT ( 'NONE',  ( 99.60459685856476142, 1.637169565754164946, -6.109999999999999432 ) ) ;
#130582=CARTESIAN_POINT ( 'NONE',  ( 28.99999999999999645, 0.000000000000000000, -7.950000000000000178 ) ) ;
#130595=CARTESIAN_POINT ( 'NONE',  ( 119.3495968585647944, 6.109999999999996767, 1.637169565754163836 ) ) ;
#130608=CARTESIAN_POINT ( 'NONE',  ( 48.27126352523143993, 4.472830434245839371, 4.472830434245842035 ) ) ;
#130619=CARTESIAN_POINT ( 'NONE',  ( 36.07876352523144448, -7.482591942790325086E-16, 6.109999999999998543 ) ) ;
#130648=CARTESIAN_POINT ( 'NONE',  ( 55.18293019189812298, -1.637169565754158951, -6.109999999999998543 ) ) ;
#130653=ORIENTED_EDGE ( 'NONE', *, *, #135623, .F. ) ;
#130682=CARTESIAN_POINT ( 'NONE',  ( 120.6620968585647802, -5.291415217122919401, 3.054999999999998384 ) ) ;
#130689=CARTESIAN_POINT ( 'NONE',  ( 67.60002705046288440, 5.819803920172570422, 5.819803920172575751 ) ) ;
#130719=CARTESIAN_POINT ( 'NONE',  ( 39.49999999999999289, 0.000000000000000000, -7.950000000000000178 ) ) ;
#130724=CARTESIAN_POINT ( 'NONE',  ( 127.0000000000000000, -4.017717506652945580, -5.045834523320674059 ) ) ;
#130725=CARTESIAN_POINT ( 'NONE',  ( 33.45376352523145158, -6.109999999999999432, -3.741295971395163529E-16 ) ) ;
#130749=CARTESIAN_POINT ( 'NONE',  ( 53.60002705046289861, 5.819803920172570422, 5.819803920172574863 ) ) ;
#130754=CARTESIAN_POINT ( 'NONE',  ( 53.79166666666667140, 3.975000000000003642, -6.884901960086285300 ) ) ;
#130755=CARTESIAN_POINT ( 'NONE',  ( 127.0000000000000000, 1.564650039245123914, 6.154215649023822010 ) ) ;
#130766=CARTESIAN_POINT ( 'NONE',  ( 43.60459685856476852, 1.637169565754164946, -6.109999999999999432 ) ) ;
#130783=CARTESIAN_POINT ( 'NONE',  ( 84.72959685856476142, -6.110000000000000320, -1.637169565754161393 ) ) ;
#130793=CARTESIAN_POINT ( 'NONE',  ( 71.80793019189812298, -6.109999999999998543, 1.637169565754158063 ) ) ;
#130823=CARTESIAN_POINT ( 'NONE',  ( 82.30793019189809456, -6.109999999999998543, 1.637169565754158507 ) ) ;
#130841=CARTESIAN_POINT ( 'NONE',  ( 122.8708603837962272, 6.884901960086289741, -3.974999999999993427 ) ) ;
#130848=CARTESIAN_POINT ( 'NONE',  ( 35.58376352523143282, -6.110000000000001208, -3.741295971395164515E-16 ) ) ;
#130850=CARTESIAN_POINT ( 'NONE',  ( 46.35416666666667851, -2.130196079827349376, -7.950000000000045475 ) ) ;
#130851=CARTESIAN_POINT ( 'NONE',  ( 90.05836038379621300, -7.949999999999996625, -2.130196079827426203 ) ) ;
#130866=CARTESIAN_POINT ( 'NONE',  ( 108.7250270504628844, 5.819803920172573974, -5.819803920172573086 ) ) ;
#130887=ORIENTED_EDGE ( 'NONE', *, *, #102832, .F. ) ;
#130893=CARTESIAN_POINT ( 'NONE',  ( 52.62499999999999289, -7.950000000000000178, -4.867971026610729436E-16 ) ) ;
#130895=CARTESIAN_POINT ( 'NONE',  ( 64.51626352523143737, -4.472830434245839371, 4.472830434245839371 ) ) ;
#130896=EDGE_CURVE ( 'NONE', #83228, #140445, #111373, .T. ) ;
#130917=CARTESIAN_POINT ( 'NONE',  ( 0.000000000000000000, 0.000000000000000000, 7.950000000000000178 ) ) ;
#130921=CARTESIAN_POINT ( 'NONE',  ( 84.80836038379621300, 7.949999999999997513, 2.130196079827431088 ) ) ;
#130937=CARTESIAN_POINT ( 'NONE',  ( 77.14626352523143282, -4.472830434245840259, 4.472830434245839371 ) ) ;
#130946=CARTESIAN_POINT ( 'NONE',  ( 0.000000000000000000, 0.000000000000000000, 7.950000000000000178 ) ) ;
#130951=CARTESIAN_POINT ( 'NONE',  ( 76.97916666666665719, -7.950000000000000178, 2.130196079827424427 ) ) ;
#130955=CARTESIAN_POINT ( 'NONE',  ( 67.95876352523144703, 0.000000000000000000, -6.110000000000001208 ) ) ;
#130984=CARTESIAN_POINT ( 'NONE',  ( 116.1412635252314374, 4.472830434245835818, 4.472830434245840259 ) ) ;
#130999=CARTESIAN_POINT ( 'NONE',  ( 50.87499999999999289, 7.950000000000000178, 1.460391307983218535E-15 ) ) ;
#131004=CARTESIAN_POINT ( 'NONE',  ( 59.79209685856477563, -5.291415217122921177, 3.054999999999999272 ) ) ;
#131008=CARTESIAN_POINT ( 'NONE',  ( 101.7920968585647756, -5.291415217122921177, 3.054999999999999272 ) ) ;
#131013=ORIENTED_EDGE ( 'NONE', *, *, #49164, .F. ) ;
#131018=CARTESIAN_POINT ( 'NONE',  ( 76.93336038379621300, 2.130196079827431532, -7.949999999999996625 ) ) ;
#131019=ORIENTED_EDGE ( 'NONE', *, *, #109794, .F. ) ;
#131023=CARTESIAN_POINT ( 'NONE',  ( 123.4329301918981088, 1.637169565754156508, 6.110000000000000320 ) ) ;
#131044=CYLINDRICAL_SURFACE ( 'NONE', #129445, 7.950000000000000178 ) ;
#131045=CARTESIAN_POINT ( 'NONE',  ( 29.60459685856477563, 1.637169565754164946, -6.109999999999999432 ) ) ;
#131055=CARTESIAN_POINT ( 'NONE',  ( 41.54166666666665719, -3.975000000000002753, 6.884901960086286188 ) ) ;
#131064=CARTESIAN_POINT ( 'NONE',  ( 115.1416937171295558, -2.130196079827424871, -7.949999999999999289 ) ) ;
#131079=EDGE_CURVE ( 'NONE', #74755, #93941, #45791, .T. ) ;
#131098=CARTESIAN_POINT ( 'NONE',  ( 40.81250000000000000, 5.819803920172571310, 5.819803920172576639 ) ) ;
#131099=CARTESIAN_POINT ( 'NONE',  ( 69.39583333333332860, -2.130196079827427091, 7.949999999999998401 ) ) ;
#131109=CARTESIAN_POINT ( 'NONE',  ( 95.95876352523144703, 0.000000000000000000, -6.110000000000001208 ) ) ;
#131115=CARTESIAN_POINT ( 'NONE',  ( 83.93336038379621300, 2.130196079827431532, -7.949999999999996625 ) ) ;
#131119=CARTESIAN_POINT ( 'NONE',  ( 48.83333333333332860, -6.884901960086287964, 3.974999999999998312 ) ) ;
#131120=CARTESIAN_POINT ( 'NONE',  ( 92.51626352523146579, -4.472830434245839371, 4.472830434245839371 ) ) ;
#131199=CARTESIAN_POINT ( 'NONE',  ( 94.99543019189812298, 5.291415217122917625, 3.055000000000002380 ) ) ;
#131249=CARTESIAN_POINT ( 'NONE',  ( 97.97916666666668561, -7.950000000000001066, 2.130196079827424427 ) ) ;
#131256=CARTESIAN_POINT ( 'NONE',  ( 89.95833333333332860, 3.974999999999997424, 6.884901960086288852 ) ) ;
#131270=CARTESIAN_POINT ( 'NONE',  ( 31.28752705046289151, 0.000000000000000000, -7.949999999999998401 ) ) ;
#131275=CARTESIAN_POINT ( 'NONE',  ( 117.2504301918981042, 3.055000000000002824, -5.291415217122919401 ) ) ;
#131286=CARTESIAN_POINT ( 'NONE',  ( 122.8495968585647518, 6.109999999999996767, 1.637169565754163836 ) ) ;
#131295=CARTESIAN_POINT ( 'NONE',  ( 47.25043019189810423, 3.055000000000002824, -5.291415217122919401 ) ) ;
#131305=CARTESIAN_POINT ( 'NONE',  ( 38.41209685856478018, 5.291415217122921177, -3.054999999999994831 ) ) ;
#131334=CARTESIAN_POINT ( 'NONE',  ( 57.22459685856477307, -1.637169565754160949, 6.109999999999997655 ) ) ;
#131375=CARTESIAN_POINT ( 'NONE',  ( 124.0162635252314658, -4.472830434245839371, 4.472830434245839371 ) ) ;
#131413=DIRECTION ( 'NONE',  ( -1.000000000000000000, -0.000000000000000000, -0.000000000000000000 ) ) ;
#131421=CARTESIAN_POINT ( 'NONE',  ( 39.87043019189810877, -3.055000000000001936, 5.291415217122918513 ) ) ;
#131447=CARTESIAN_POINT ( 'NONE',  ( 57.97502705046289151, -5.819803920172572198, 5.819803920172572198 ) ) ;
#131453=CARTESIAN_POINT ( 'NONE',  ( 55.68749999999999289, -5.819803920172573086, 5.819803920172572198 ) ) ;
#131461=CARTESIAN_POINT ( 'NONE',  ( 44.04209685856477563, 5.291415217122923842, -3.054999999999996163 ) ) ;
#131476=CARTESIAN_POINT ( 'NONE',  ( 80.20876352523143282, -7.482591942790329030E-16, 6.110000000000001208 ) ) ;
#131483=CARTESIAN_POINT ( 'NONE',  ( 70.49543019189810877, 5.291415217122916737, 3.055000000000001936 ) ) ;
#131491=ORIENTED_EDGE ( 'NONE', *, *, #88741, .F. ) ;
#131496=LINE ( 'NONE', #33631, #136996 ) ;
#131508=CARTESIAN_POINT ( 'NONE',  ( 52.14169371712954870, -2.130196079827424871, -7.949999999999998401 ) ) ;
#131515=CARTESIAN_POINT ( 'NONE',  ( 88.28709685856478018, 3.054999999999997495, 5.291415217122919401 ) ) ;
#131534=CARTESIAN_POINT ( 'NONE',  ( 38.06293019189810423, 1.637169565754157174, 6.110000000000002984 ) ) ;
#131544=CYLINDRICAL_SURFACE ( 'NONE', #34168, 7.950000000000000178 ) ;
#131579=ORIENTED_EDGE ( 'NONE', *, *, #118122, .T. ) ;
#131591=CARTESIAN_POINT ( 'NONE',  ( 63.93293019189812298, 1.637169565754156730, 6.110000000000001208 ) ) ;
#131596=ORIENTED_EDGE ( 'NONE', *, *, #26008, .T. ) ;
#131614=LINE ( 'NONE', #130917, #141226 ) ;
#131622=CARTESIAN_POINT ( 'NONE',  ( 88.89169371712954160, 2.130196079827421762, 7.950000000000001066 ) ) ;
#131626=CARTESIAN_POINT ( 'NONE',  ( 85.43750000000001421, 5.819803920172573974, -5.819803920172572198 ) ) ;
#131637=CARTESIAN_POINT ( 'NONE',  ( 79.33376352523144703, 6.110000000000001208, 1.122388791418549305E-15 ) ) ;
#131657=CARTESIAN_POINT ( 'NONE',  ( 62.41709685856476852, 3.054999999999998828, 5.291415217122922066 ) ) ;
#131685=CARTESIAN_POINT ( 'NONE',  ( 109.8704301918981230, -3.055000000000001492, 5.291415217122917625 ) ) ;
#131708=CARTESIAN_POINT ( 'NONE',  ( 64.89626352523143282, 4.472830434245840259, -4.472830434245838482 ) ) ;
#131715=CARTESIAN_POINT ( 'NONE',  ( 95.52126352523141861, -4.472830434245838482, -4.472830434245840259 ) ) ;
#131725=( BOUNDED_CURVE ( )  B_SPLINE_CURVE ( 2, ( #21624, #120924, #54980, #52791, #87591, #120174, #76001, #65880, #75305, #63718, #20886, #131099, #64406 ),
 .UNSPECIFIED., .F., .F. ) 
 B_SPLINE_CURVE_WITH_KNOTS ( ( 3, 2, 2, 2, 2, 2, 3 ),
 ( 0.5333333333333334370, 0.5361111111111112049, 0.5388888888888889728, 0.5416666666666667407, 0.5444444444444443976, 0.5472222222222222765, 0.5500000000000000444 ),
 .UNSPECIFIED. ) 
 CURVE ( )  GEOMETRIC_REPRESENTATION_ITEM ( )  RATIONAL_B_SPLINE_CURVE ( ( 0.9999999999999986677, 0.9659258262890696445, 1.000000000000000000, 0.9659258262890683122, 1.000000000000000000, 0.9659258262890683122, 1.000000000000000000, 0.9659258262890683122, 1.000000000000000000, 0.9659258262890683122, 1.000000000000000000, 0.9659258262890683122, 1.000000000000000000 ) ) 
 REPRESENTATION_ITEM ( '' )  );
#131734=CARTESIAN_POINT ( 'NONE',  ( 126.6412635252314516, 4.472830434245835818, 4.472830434245840259 ) ) ;
#131737=( BOUNDED_CURVE ( )  B_SPLINE_CURVE ( 2, ( #121796, #1437, #66735, #78328, #47180, #91362, #110911, #11594, #56620, #55878, #100079, #89203, #122519 ),
 .UNSPECIFIED., .F., .T. ) 
 B_SPLINE_CURVE_WITH_KNOTS ( ( 3, 2, 2, 2, 2, 2, 3 ),
 ( 0.4000000000000000222, 0.4027777777777777901, 0.4055555555555555580, 0.4083333333333333259, 0.4111111111111110938, 0.4138888888888888618, 0.4166666666666666852 ),
 .UNSPECIFIED. ) 
 CURVE ( )  GEOMETRIC_REPRESENTATION_ITEM ( )  RATIONAL_B_SPLINE_CURVE ( ( 1.000000000000000000, 0.9659258262890683122, 1.000000000000000000, 0.9659258262890683122, 1.000000000000000000, 0.9659258262890683122, 1.000000000000000000, 0.9659258262890683122, 1.000000000000000000, 0.9659258262890683122, 1.000000000000000000, 0.9659258262890683122, 1.000000000000000000 ) ) 
 REPRESENTATION_ITEM ( '' )  );
#131751=B_SPLINE_CURVE_WITH_KNOTS ( 'NONE', 1,
 ( #68922, #123302 ),
 .UNSPECIFIED., .F., .F.,
 ( 2, 2 ),
 ( 0.000000000000000000, 0.1304347826086980078 ),
 .UNSPECIFIED. ) ;
#131753=CARTESIAN_POINT ( 'NONE',  ( 37.74999999999999289, -9.735942053221458872E-16, 7.950000000000000178 ) ) ;
#131757=CARTESIAN_POINT ( 'NONE',  ( 58.02083333333332149, 7.949999999999998401, 2.130196079827431532 ) ) ;
#131764=CARTESIAN_POINT ( 'NONE',  ( 32.22959685856477563, -6.110000000000000320, -1.637169565754161393 ) ) ;
#131785=CARTESIAN_POINT ( 'NONE',  ( 110.1833603837962130, -2.130196079827426203, 7.949999999999997513 ) ) ;
#131824=CARTESIAN_POINT ( 'NONE',  ( 95.52126352523141861, -4.472830434245839371, -4.472830434245840259 ) ) ;
#131835=CARTESIAN_POINT ( 'NONE',  ( 83.03709685856478018, -3.054999999999998828, -5.291415217122919401 ) ) ;
#131925=CARTESIAN_POINT ( 'NONE',  ( 92.66209685856479439, -5.291415217122919401, 3.054999999999998384 ) ) ;
#131927=CARTESIAN_POINT ( 'NONE',  ( 6.342504469876894646, -9.325618364798961224, -1.816862207259552608 ) ) ;
#131930=ORIENTED_EDGE ( 'NONE', *, *, #71435, .F. ) ;
#131967=CARTESIAN_POINT ( 'NONE',  ( 31.04166666666666075, -3.975000000000002753, 6.884901960086286188 ) ) ;
#131970=CYLINDRICAL_SURFACE ( 'NONE', #83110, 7.950000000000000178 ) ;
#131977=CARTESIAN_POINT ( 'NONE',  ( 101.2875270504628986, 0.000000000000000000, -7.949999999999998401 ) ) ;
#131980=CARTESIAN_POINT ( 'NONE',  ( 101.7708333333333428, -7.949999999999999289, -2.130196079827426203 ) ) ;
#132000=CARTESIAN_POINT ( 'NONE',  ( 27.20419371712955225, -6.884901960086285300, -3.975000000000000089 ) ) ;
#132004=CARTESIAN_POINT ( 'NONE',  ( 121.7712635252314328, 4.472830434245839371, 4.472830434245842035 ) ) ;
#132013=CARTESIAN_POINT ( 'NONE',  ( 113.5162635252314516, -4.472830434245839371, 4.472830434245839371 ) ) ;
#132016=CARTESIAN_POINT ( 'NONE',  ( 69.78752705046289861, 0.000000000000000000, -7.949999999999998401 ) ) ;
#132024=CARTESIAN_POINT ( 'NONE',  ( 40.68793019189811133, 6.110000000000002984, -1.637169565754156730 ) ) ;
#132033=CARTESIAN_POINT ( 'NONE',  ( 41.91209685856478728, 5.291415217122921177, -3.054999999999994831 ) ) ;
#132062=EDGE_CURVE ( 'NONE', #129167, #133316, #133714, .T. ) ;
#132065=CARTESIAN_POINT ( 'NONE',  ( 48.91209685856478018, 5.291415217122921177, -3.054999999999994831 ) ) ;
#132083=ORIENTED_EDGE ( 'NONE', *, *, #106068, .F. ) ;
#132103=CARTESIAN_POINT ( 'NONE',  ( 124.4537635252314516, -6.109999999999999432, -3.741295971395163529E-16 ) ) ;
#132136=LINE ( 'NONE', #74912, #73683 ) ;
#132145=CARTESIAN_POINT ( 'NONE',  ( 41.03709685856478728, -3.054999999999999272, -5.291415217122919401 ) ) ;
#132150=CARTESIAN_POINT ( 'NONE',  ( 125.8333333333333286, -6.884901960086287964, 3.974999999999998312 ) ) ;
#132163=CARTESIAN_POINT ( 'NONE',  ( 117.8337635252314470, 6.110000000000001208, 1.122388791418549305E-15 ) ) ;
#132173=CARTESIAN_POINT ( 'NONE',  ( 55.64169371712955581, -2.130196079827424871, -7.949999999999999289 ) ) ;
#132178=CARTESIAN_POINT ( 'NONE',  ( 48.10416666666665009, 2.130196079827422206, 7.950000000000001954 ) ) ;
#132185=CARTESIAN_POINT ( 'NONE',  ( 44.62543019189810423, 5.291415217122919401, 3.055000000000002824 ) ) ;
#132195=CYLINDRICAL_SURFACE ( 'NONE', #9316, 7.950000000000000178 ) ;
#132196=ADVANCED_FACE ( 'NONE', ( #32257 ), #120659, .F. ) ;
#132204=CARTESIAN_POINT ( 'NONE',  ( 82.39626352523143282, 4.472830434245840259, -4.472830434245838482 ) ) ;
#132215=CARTESIAN_POINT ( 'NONE',  ( 64.95376352523145158, -6.109999999999998543, -3.741295971395162543E-16 ) ) ;
#132222=( NAMED_UNIT ( * ) PLANE_ANGLE_UNIT ( ) SI_UNIT ( $, .RADIAN. ) );
#132241=CARTESIAN_POINT ( 'NONE',  ( 41.05836038379621300, -7.949999999999996625, -2.130196079827426203 ) ) ;
#132244=CARTESIAN_POINT ( 'NONE',  ( 51.99586038379622011, -3.974999999999998312, -6.884901960086286188 ) ) ;
#132251=CARTESIAN_POINT ( 'NONE',  ( 76.76626352523142316, 4.472830434245838482, -4.472830434245837594 ) ) ;
#132298=DIRECTION ( 'NONE',  ( 0.000000000000000000, 1.224646799147353454E-16, 1.000000000000000000 ) ) ;
#132331=CARTESIAN_POINT ( 'NONE',  ( 62.76626352523144448, 4.472830434245839371, -4.472830434245839371 ) ) ;
#132333=DIRECTION ( 'NONE',  ( 0.000000000000000000, 0.000000000000000000, 1.000000000000000000 ) ) ;
#132338=CARTESIAN_POINT ( 'NONE',  ( 83.39583333333334281, -2.130196079827351596, 7.950000000000043698 ) ) ;
#132344=VECTOR ( 'NONE', #98430, 1000.000000000000000 ) ;
#132362=CARTESIAN_POINT ( 'NONE',  ( 83.35002705046287019, -5.819803920172572198, -5.819803920172572198 ) ) ;
#132366=CARTESIAN_POINT ( 'NONE',  ( 76.54166666666667140, -3.975000000000002753, 6.884901960086286188 ) ) ;
#132376=CARTESIAN_POINT ( 'NONE',  ( 71.60459685856477563, 1.637169565754164946, -6.109999999999999432 ) ) ;
#132396=ADVANCED_FACE ( 'NONE', ( #64000 ), #95180, .T. ) ;
#132399=CARTESIAN_POINT ( 'NONE',  ( 68.97959685856477563, 6.109999999999999432, 1.637169565754164280 ) ) ;
#132435=CARTESIAN_POINT ( 'NONE',  ( 106.5162635252314658, -4.472830434245838482, 4.472830434245838482 ) ) ;
#132438=CARTESIAN_POINT ( 'NONE',  ( 0.000000000000000000, 0.000000000000000000, 0.000000000000000000 ) ) ;
#132447=CARTESIAN_POINT ( 'NONE',  ( 36.29166666666666430, 3.975000000000003642, -6.884901960086285300 ) ) ;
#132457=CARTESIAN_POINT ( 'NONE',  ( 87.33333333333332860, -6.884901960086287964, 3.974999999999998312 ) ) ;
#132462=CARTESIAN_POINT ( 'NONE',  ( 66.64626352523144703, -4.472830434245840259, 4.472830434245838482 ) ) ;
#132467=CARTESIAN_POINT ( 'NONE',  ( 102.2295968585647614, -6.110000000000000320, -1.637169565754161393 ) ) ;
#132485=CARTESIAN_POINT ( 'NONE',  ( 120.9537635252314658, -6.109999999999998543, -3.741295971395162543E-16 ) ) ;
#132517=ORIENTED_EDGE ( 'NONE', *, *, #139990, .F. ) ;
#132532=CARTESIAN_POINT ( 'NONE',  ( 113.2458603837962272, 3.974999999999996980, 6.884901960086287964 ) ) ;
#132570=CARTESIAN_POINT ( 'NONE',  ( 96.97959685856478984, 6.109999999999999432, 1.637169565754164280 ) ) ;
#132579=CARTESIAN_POINT ( 'NONE',  ( 49.27083333333333570, -7.949999999999998401, -2.130196079827426203 ) ) ;
#132581=CARTESIAN_POINT ( 'NONE',  ( 82.01626352523142316, -4.472830434245839371, 4.472830434245839371 ) ) ;
#132616=CARTESIAN_POINT ( 'NONE',  ( 118.2500000000000000, -9.735942053221458872E-16, 7.950000000000000178 ) ) ;
#132622=CARTESIAN_POINT ( 'NONE',  ( 116.7458603837962272, 3.974999999999996980, 6.884901960086287964 ) ) ;
#132667=CARTESIAN_POINT ( 'NONE',  ( 85.07876352523143737, -7.482591942790327058E-16, 6.109999999999999432 ) ) ;
#132668=CARTESIAN_POINT ( 'NONE',  ( 6.403482346239627532, -9.299335578761299459, 1.960683619075200390 ) ) ;
#132674=ORIENTED_EDGE ( 'NONE', *, *, #97777, .T. ) ;
#132718=CARTESIAN_POINT ( 'NONE',  ( 100.1666666666666714, 6.884901960086285300, 3.975000000000003642 ) ) ;
#132740=CARTESIAN_POINT ( 'NONE',  ( 120.3129301918980758, -1.637169565754159617, -6.110000000000001208 ) ) ;
#132744=AXIS2_PLACEMENT_3D ( 'NONE', #114449, #48487, #89840 ) ;
#132751=CARTESIAN_POINT ( 'NONE',  ( 116.5787635252314516, -7.482591942790325086E-16, 6.109999999999998543 ) ) ;
#132756=CARTESIAN_POINT ( 'NONE',  ( 98.27083333333332860, -7.949999999999998401, -2.130196079827426203 ) ) ;
#132760=CARTESIAN_POINT ( 'NONE',  ( 39.08376352523143282, -6.110000000000001208, -3.741295971395164515E-16 ) ) ;
#132768=CARTESIAN_POINT ( 'NONE',  ( 30.39126352523144448, -4.472830434245839371, -4.472830434245839371 ) ) ;
#132771=EDGE_LOOP ( 'NONE', ( #17196, #63019, #42810, #115216 ) ) ;
#132799=CARTESIAN_POINT ( 'NONE',  ( 50.51626352523143737, -4.472830434245838482, 4.472830434245838482 ) ) ;
#132832=CARTESIAN_POINT ( 'NONE',  ( 107.5370968585647944, -3.054999999999999272, -5.291415217122919401 ) ) ;
#132862=CARTESIAN_POINT ( 'NONE',  ( 26.99999999999998579, -7.850927237173508821, -1.251176053402193178 ) ) ;
#132869=CARTESIAN_POINT ( 'NONE',  ( 26.89126352523144092, -4.472830434245839371, -4.472830434245839371 ) ) ;
#132875=CARTESIAN_POINT ( 'NONE',  ( 126.1250000000000142, -7.950000000000000178, -4.867971026610729436E-16 ) ) ;
#132890=CARTESIAN_POINT ( 'NONE',  ( 122.2087635252314328, -7.482591942790329030E-16, 6.110000000000001208 ) ) ;
#132901=CARTESIAN_POINT ( 'NONE',  ( 47.47502705046288440, -5.819803920172572198, 5.819803920172572198 ) ) ;
#132907=CARTESIAN_POINT ( 'NONE',  ( 47.08333333333332149, 6.884901960086290629, -3.974999999999994316 ) ) ;
#132917=CARTESIAN_POINT ( 'NONE',  ( 37.77126352523144703, 4.472830434245839371, 4.472830434245842035 ) ) ;
#132931=ORIENTED_EDGE ( 'NONE', *, *, #56539, .T. ) ;
#132932=CARTESIAN_POINT ( 'NONE',  ( 79.77126352523143282, 4.472830434245838482, 4.472830434245842035 ) ) ;
#132941=CARTESIAN_POINT ( 'NONE',  ( 58.53709685856478728, -3.054999999999998828, -5.291415217122919401 ) ) ;
#132952=LINE ( 'NONE', #119172, #14356 ) ;
#132970=CARTESIAN_POINT ( 'NONE',  ( 78.51626352523143737, -4.472830434245838482, 4.472830434245838482 ) ) ;
#133043=CARTESIAN_POINT ( 'NONE',  ( 54.59959685856476597, -6.109999999999998543, -1.637169565754160727 ) ) ;
#133048=CARTESIAN_POINT ( 'NONE',  ( 32.01669371712954160, 7.950000000000000178, -2.130196079827421318 ) ) ;
#133069=CARTESIAN_POINT ( 'NONE',  ( 81.01669371712955581, 7.950000000000001066, -2.130196079827421318 ) ) ;
#133073=CARTESIAN_POINT ( 'NONE',  ( 77.41666666666665719, -6.884901960086287076, -3.975000000000000977 ) ) ;
#133085=CARTESIAN_POINT ( 'NONE',  ( 67.95876352523144703, 0.000000000000000000, -6.110000000000001208 ) ) ;
#133103=CARTESIAN_POINT ( 'NONE',  ( 68.39626352523141861, 4.472830434245840259, -4.472830434245839371 ) ) ;
#133132=CARTESIAN_POINT ( 'NONE',  ( 105.6412635252314516, 4.472830434245835818, 4.472830434245840259 ) ) ;
#133140=ADVANCED_FACE ( 'NONE', ( #70295 ), #134085, .T. ) ;
#133157=CARTESIAN_POINT ( 'NONE',  ( 55.12543019189811133, 5.291415217122919401, 3.055000000000002824 ) ) ;
#133162=CARTESIAN_POINT ( 'NONE',  ( 90.56293019189810423, 1.637169565754157174, 6.110000000000002984 ) ) ;
#133174=ORIENTED_EDGE ( 'NONE', *, *, #16296, .F. ) ;
#133177=CARTESIAN_POINT ( 'NONE',  ( 122.9954301918981230, 5.291415217122916737, 3.055000000000001936 ) ) ;
#133203=EDGE_CURVE ( 'NONE', #106661, #83402, #137659, .T. ) ;
#133212=CARTESIAN_POINT ( 'NONE',  ( 125.5000000000000000, -3.441786896390352624, 7.166352137582667758 ) ) ;
#133230=CARTESIAN_POINT ( 'NONE',  ( 114.4125270504628986, -7.949999999999998401, -4.867971026610728450E-16 ) ) ;
#133244=CARTESIAN_POINT ( 'NONE',  ( 102.2295968585647614, -6.110000000000000320, -1.637169565754161393 ) ) ;
#133267=CARTESIAN_POINT ( 'NONE',  ( 90.70876352523143282, -7.482591942790329030E-16, 6.110000000000001208 ) ) ;
#133278=CARTESIAN_POINT ( 'NONE',  ( 81.72459685856476597, -1.637169565754160949, 6.109999999999997655 ) ) ;
#133302=AXIS2_PLACEMENT_3D ( 'NONE', #65836, #19424, #142639 ) ;
#133307=CARTESIAN_POINT ( 'NONE',  ( 56.07919371712956291, 3.975000000000002753, -6.884901960086283523 ) ) ;
#133311=CARTESIAN_POINT ( 'NONE',  ( 119.7083333333333286, -3.974999999999999201, -6.884901960086287964 ) ) ;
#133316=VERTEX_POINT ( 'NONE', #54928 ) ;
#133327=CARTESIAN_POINT ( 'NONE',  ( 119.2920968585647756, -5.291415217122921177, 3.054999999999999272 ) ) ;
#133354=CARTESIAN_POINT ( 'NONE',  ( 84.05793019189810877, 6.110000000000001208, -1.637169565754156286 ) ) ;
#133374=DIRECTION ( 'NONE',  ( -1.000000000000000000, -0.000000000000000000, -0.000000000000000000 ) ) ;
#133406=ORIENTED_EDGE ( 'NONE', *, *, #65445, .F. ) ;
#133407=CARTESIAN_POINT ( 'NONE',  ( 105.5624999999999858, -5.819803920172572198, -5.819803920172573086 ) ) ;
#133411=ADVANCED_FACE ( 'NONE', ( #52751 ), #118731, .T. ) ;
#133431=CARTESIAN_POINT ( 'NONE',  ( 117.6879301918981184, 6.110000000000002984, -1.637169565754156730 ) ) ;
#133439=CARTESIAN_POINT ( 'NONE',  ( 114.8287635252314516, 0.000000000000000000, -6.109999999999998543 ) ) ;
#133449=CARTESIAN_POINT ( 'NONE',  ( 39.52126352523143282, -4.472830434245839371, -4.472830434245840259 ) ) ;
#133456=CARTESIAN_POINT ( 'NONE',  ( 28.78709685856477307, 3.054999999999997495, 5.291415217122919401 ) ) ;
#133461=VERTEX_POINT ( 'NONE', #104095 ) ;
#133487=CARTESIAN_POINT ( 'NONE',  ( 50.95376352523145158, -6.109999999999998543, -3.741295971395162543E-16 ) ) ;
#133519=CARTESIAN_POINT ( 'NONE',  ( 113.8079301918981230, -6.109999999999999432, 1.637169565754158507 ) ) ;
#133564=CARTESIAN_POINT ( 'NONE',  ( 126.1802896944664525, -7.122564593600495542, 1.486291407750432114 ) ) ;
#133565=CARTESIAN_POINT ( 'NONE',  ( 32.28709685856477307, 3.054999999999997939, 5.291415217122920289 ) ) ;
#133582=CARTESIAN_POINT ( 'NONE',  ( 121.3337635252314328, 6.110000000000001208, 1.122388791418549305E-15 ) ) ;
#133594=CARTESIAN_POINT ( 'NONE',  ( 44.85002705046287730, -5.819803920172572198, -5.819803920172572198 ) ) ;
#133601=CARTESIAN_POINT ( 'NONE',  ( 42.41666666666665719, -6.884901960086287076, -3.975000000000000977 ) ) ;
#133609=CARTESIAN_POINT ( 'NONE',  ( 42.00043019189809712, -3.055000000000002380, 5.291415217122920289 ) ) ;
#133630=CARTESIAN_POINT ( 'NONE',  ( 62.18293019189812298, -1.637169565754158951, -6.109999999999998543 ) ) ;
#133635=ORIENTED_EDGE ( 'NONE', *, *, #16007, .T. ) ;
#133637=( LENGTH_UNIT ( ) NAMED_UNIT ( * ) SI_UNIT ( .MILLI., .METRE. ) );
#133657=CARTESIAN_POINT ( 'NONE',  ( 79.24543019189810877, -5.291415217122918513, -3.055000000000000160 ) ) ;
#133681=CARTESIAN_POINT ( 'NONE',  ( 28.14626352523143638, -4.472830434245840259, 4.472830434245838482 ) ) ;
#133714=LINE ( 'NONE', #66323, #7464 ) ;
#133737=CARTESIAN_POINT ( 'NONE',  ( 53.87043019189811588, -3.055000000000001936, 5.291415217122918513 ) ) ;
#133757=CARTESIAN_POINT ( 'NONE',  ( 78.39169371712955581, 2.130196079827421762, 7.950000000000001066 ) ) ;
#133763=CARTESIAN_POINT ( 'NONE',  ( 78.00000000000000000, 0.000000000000000000, -7.950000000000000178 ) ) ;
#133771=CARTESIAN_POINT ( 'NONE',  ( 63.43793019189811133, -6.110000000000001208, 1.637169565754158951 ) ) ;
#133792=CARTESIAN_POINT ( 'NONE',  ( 56.14626352523143282, -4.472830434245840259, 4.472830434245839371 ) ) ;
#133799=CARTESIAN_POINT ( 'NONE',  ( 54.22916666666666430, 7.950000000000001954, -2.130196079827421762 ) ) ;
#133822=CARTESIAN_POINT ( 'NONE',  ( 106.8079301918981230, -6.109999999999998543, 1.637169565754158507 ) ) ;
#133835=CARTESIAN_POINT ( 'NONE',  ( 160.0000000000000000, 0.000000000000000000, 0.000000000000000000 ) ) ;
#133846=CARTESIAN_POINT ( 'NONE',  ( 54.10459685856476852, 1.637169565754164946, -6.109999999999999432 ) ) ;
#133852=CARTESIAN_POINT ( 'NONE',  ( 93.91709685856477563, 3.054999999999998828, 5.291415217122922066 ) ) ;
#133865=DIRECTION ( 'NONE',  ( -0.000000000000000000, 1.000000000000000000, -0.000000000000000000 ) ) ;
#133896=CARTESIAN_POINT ( 'NONE',  ( 7.652374387692081115, 8.843121118309934303, -3.475427755405318120 ) ) ;
#133902=DIRECTION ( 'NONE',  ( -1.000000000000000000, -0.000000000000000000, -0.000000000000000000 ) ) ;
#133905=VERTEX_POINT ( 'NONE', #142144 ) ;
#133915=VERTEX_POINT ( 'NONE', #131977 ) ;
#133920=CARTESIAN_POINT ( 'NONE',  ( 99.82919371712955581, -3.975000000000001865, 6.884901960086284411 ) ) ;
#133937=CARTESIAN_POINT ( 'NONE',  ( 94.35459685856476142, -1.637169565754161615, 6.110000000000000320 ) ) ;
#133957=CARTESIAN_POINT ( 'NONE',  ( 95.81293019189807580, -1.637169565754159617, -6.110000000000001208 ) ) ;
#133967=CARTESIAN_POINT ( 'NONE',  ( 88.72459685856478018, -1.637169565754160949, 6.109999999999997655 ) ) ;
#134033=CARTESIAN_POINT ( 'NONE',  ( 115.2087635252314470, -7.482591942790329030E-16, 6.110000000000001208 ) ) ;
#134048=ORIENTED_EDGE ( 'NONE', *, *, #88489, .F. ) ;
#134064=CARTESIAN_POINT ( 'NONE',  ( 86.68293019189813720, -1.637169565754159173, -6.109999999999999432 ) ) ;
#134085=CYLINDRICAL_SURFACE ( 'NONE', #132744, 6.349999999999999645 ) ;
#134102=CARTESIAN_POINT ( 'NONE',  ( 47.76669371712955581, -7.949999999999998401, 2.130196079827423983 ) ) ;
#134117=CARTESIAN_POINT ( 'NONE',  ( 105.4166666666666572, -6.884901960086287076, -3.975000000000000977 ) ) ;
#134124=CARTESIAN_POINT ( 'NONE',  ( 14.69992816670506208, 9.499966918880492273, -0.1465975642050108829 ) ) ;
#134145=CARTESIAN_POINT ( 'NONE',  ( 122.6462635252314328, -4.472830434245840259, 4.472830434245839371 ) ) ;
#134147=CARTESIAN_POINT ( 'NONE',  ( 99.43749999999998579, 5.819803920172574863, -5.819803920172573086 ) ) ;
#134152=CARTESIAN_POINT ( 'NONE',  ( 117.5995968585647944, -6.109999999999997655, -1.637169565754160283 ) ) ;
#134157=ORIENTED_EDGE ( 'NONE', *, *, #67563, .F. ) ;
#134165=CARTESIAN_POINT ( 'NONE',  ( 32.14126352523144448, 4.472830434245836706, 4.472830434245840259 ) ) ;
#134200=CARTESIAN_POINT ( 'NONE',  ( 49.05793019189810877, 6.110000000000000320, -1.637169565754156064 ) ) ;
#134204=LINE ( 'NONE', #70420, #91336 ) ;
#134210=AXIS2_PLACEMENT_3D ( 'NONE', #142527, #22135, #55516 ) ;
#134236=CARTESIAN_POINT ( 'NONE',  ( 106.8079301918981230, -6.109999999999999432, 1.637169565754158507 ) ) ;
#134274=CARTESIAN_POINT ( 'NONE',  ( 125.9076131992937775, -6.355826491133410805, 4.106188095953474892 ) ) ;
#134298=CARTESIAN_POINT ( 'NONE',  ( 119.4379301918981042, -6.110000000000001208, 1.637169565754158951 ) ) ;
#134309=CARTESIAN_POINT ( 'NONE',  ( 45.57919371712955581, 3.975000000000002753, -6.884901960086283523 ) ) ;
#134314=CARTESIAN_POINT ( 'NONE',  ( 43.00000000000000000, 0.000000000000000000, -7.950000000000000178 ) ) ;
#134319=CARTESIAN_POINT ( 'NONE',  ( 127.0000000000000568, -4.122959376248258145, -4.874446087595273092 ) ) ;
#134323=CARTESIAN_POINT ( 'NONE',  ( 41.12543019189809712, 5.291415217122919401, 3.055000000000002824 ) ) ;
#134337=CARTESIAN_POINT ( 'NONE',  ( 39.30836038379622011, 7.949999999999996625, 2.130196079827431088 ) ) ;
#134346=CARTESIAN_POINT ( 'NONE',  ( 87.28752705046288440, 0.000000000000000000, -7.949999999999998401 ) ) ;
#134347=CARTESIAN_POINT ( 'NONE',  ( 58.97459685856478018, 1.637169565754164058, -6.109999999999996767 ) ) ;
#134377=ORIENTED_EDGE ( 'NONE', *, *, #64308, .T. ) ;
#134378=CARTESIAN_POINT ( 'NONE',  ( 71.37043019189812298, -3.055000000000001492, 5.291415217122917625 ) ) ;
#134404=CARTESIAN_POINT ( 'NONE',  ( 30.47959685856476852, 6.109999999999999432, 1.637169565754164280 ) ) ;
#134454=CARTESIAN_POINT ( 'NONE',  ( 53.43293019189810167, 1.637169565754156730, 6.110000000000001208 ) ) ;
#134479=CARTESIAN_POINT ( 'NONE',  ( 116.6458333333333570, 2.130196079827470168, -7.949999999999977973 ) ) ;
#134480=CARTESIAN_POINT ( 'NONE',  ( 76.78752705046289861, 0.000000000000000000, -7.949999999999998401 ) ) ;
#134484=CARTESIAN_POINT ( 'NONE',  ( 70.85416666666667140, -2.130196079827425315, -7.950000000000001066 ) ) ;
#134495=CARTESIAN_POINT ( 'NONE',  ( 65.47959685856477563, 6.109999999999999432, 1.637169565754164280 ) ) ;
#134504=CARTESIAN_POINT ( 'NONE',  ( 44.45833333333332149, 3.974999999999997424, 6.884901960086288852 ) ) ;
#134516=CARTESIAN_POINT ( 'NONE',  ( 55.70876352523143282, -7.482591942790329030E-16, 6.110000000000001208 ) ) ;
#134525=CARTESIAN_POINT ( 'NONE',  ( 125.5000000000000568, -3.922572014496796822, -6.914906274931464480 ) ) ;
#134526=CARTESIAN_POINT ( 'NONE',  ( 55.24999999999999289, -9.735942053221458872E-16, 7.950000000000000178 ) ) ;
#134547=CARTESIAN_POINT ( 'NONE',  ( 36.97502705046289151, -5.819803920172573086, 5.819803920172573086 ) ) ;
#134553=CARTESIAN_POINT ( 'NONE',  ( 102.2870968585647802, 3.054999999999997495, 5.291415217122919401 ) ) ;
#134559=CYLINDRICAL_SURFACE ( 'NONE', #26190, 7.950000000000000178 ) ;
#134570=CARTESIAN_POINT ( 'NONE',  ( 27.20419371712955225, -6.884901960086285300, -3.975000000000000089 ) ) ;
#134581=CARTESIAN_POINT ( 'NONE',  ( 56.72959685856476142, -6.110000000000000320, -1.637169565754161393 ) ) ;
#134588=CARTESIAN_POINT ( 'NONE',  ( 92.60459685856477563, 1.637169565754164946, -6.109999999999999432 ) ) ;
#134597=CARTESIAN_POINT ( 'NONE',  ( 127.2245968585647660, -1.637169565754161171, 6.109999999999998543 ) ) ;
#134602=EDGE_LOOP ( 'NONE', ( #85829, #47974, #28690, #137891 ) ) ;
#134630=CARTESIAN_POINT ( 'NONE',  ( 8.122631387037495543, 8.712540773999728927, 3.790917003805983843 ) ) ;
#134656=CARTESIAN_POINT ( 'NONE',  ( 106.8291937171295700, -3.975000000000001865, 6.884901960086284411 ) ) ;
#134659=ORIENTED_EDGE ( 'NONE', *, *, #120413, .T. ) ;
#134670=VERTEX_POINT ( 'NONE', #19120 ) ;
#134674=CARTESIAN_POINT ( 'NONE',  ( 96.97959685856478984, 6.109999999999999432, 1.637169565754164280 ) ) ;
#134700=CARTESIAN_POINT ( 'NONE',  ( 84.87543019189810423, -5.291415217122920289, -3.055000000000001492 ) ) ;
#134717=CARTESIAN_POINT ( 'NONE',  ( 82.89126352523142316, -4.472830434245839371, -4.472830434245839371 ) ) ;
#134732=PLANE ( 'NONE',  #129917 ) ;
#134770=CARTESIAN_POINT ( 'NONE',  ( 120.6045968585647756, 1.637169565754164946, -6.109999999999999432 ) ) ;
#134799=CARTESIAN_POINT ( 'NONE',  ( 84.64126352523145158, 4.472830434245837594, 4.472830434245841147 ) ) ;
#134800=CARTESIAN_POINT ( 'NONE',  ( 8.902796541008825670, -8.547859821797413105, 4.147131456889309398 ) ) ;
#134846=DIRECTION ( 'NONE',  ( 0.000000000000000000, 0.000000000000000000, 1.000000000000000000 ) ) ;
#134852=CARTESIAN_POINT ( 'NONE',  ( 93.75000000000000000, -9.735942053221458872E-16, 7.950000000000000178 ) ) ;
#134861=CARTESIAN_POINT ( 'NONE',  ( 13.21932050955820692, 8.913545539526866790, -3.292927883844741110 ) ) ;
#134879=CARTESIAN_POINT ( 'NONE',  ( 113.6045968585647614, 1.637169565754164946, -6.109999999999999432 ) ) ;
#134884=CARTESIAN_POINT ( 'NONE',  ( 99.29166666666667140, 3.975000000000003642, -6.884901960086285300 ) ) ;
#134889=CARTESIAN_POINT ( 'NONE',  ( 109.4329301918981088, 1.637169565754156508, 6.110000000000000320 ) ) ;
#134895=CARTESIAN_POINT ( 'NONE',  ( 97.39583333333332860, -2.130196079827427091, 7.949999999999998401 ) ) ;
#134904=CARTESIAN_POINT ( 'NONE',  ( 29.66209685856477307, -5.291415217122919401, 3.054999999999997939 ) ) ;
#134938=CARTESIAN_POINT ( 'NONE',  ( 34.47459685856478728, 1.637169565754164280, -6.109999999999996767 ) ) ;
#134969=CARTESIAN_POINT ( 'NONE',  ( 110.5995968585647802, -6.109999999999998543, -1.637169565754160727 ) ) ;
#134995=EDGE_LOOP ( 'NONE', ( #10239, #27322, #51341, #10634 ) ) ;
#135001=VERTEX_POINT ( 'NONE', #113990 ) ;
#135021=CARTESIAN_POINT ( 'NONE',  ( 115.6250000000000000, -7.950000000000000178, -4.867971026610729436E-16 ) ) ;
#135037=CARTESIAN_POINT ( 'NONE',  ( 123.9587635252314470, 0.000000000000000000, -6.110000000000001208 ) ) ;
#135047=CARTESIAN_POINT ( 'NONE',  ( 50.68336038379622011, -2.130196079827426203, 7.949999999999997513 ) ) ;
#135053=CARTESIAN_POINT ( 'NONE',  ( 45.77083333333332149, -7.949999999999999289, -2.130196079827426203 ) ) ;
#135061=CARTESIAN_POINT ( 'NONE',  ( 39.52126352523143282, -4.472830434245839371, -4.472830434245840259 ) ) ;
#135076=CARTESIAN_POINT ( 'NONE',  ( 38.87086038379622721, 6.884901960086289741, -3.974999999999993427 ) ) ;
#135083=VECTOR ( 'NONE', #44610, 1000.000000000000000 ) ;
#135085=CARTESIAN_POINT ( 'NONE',  ( 55.32876352523144448, 0.000000000000000000, -6.109999999999998543 ) ) ;
#135114=CARTESIAN_POINT ( 'NONE',  ( 75.45376352523145158, -6.109999999999998543, -3.741295971395162543E-16 ) ) ;
#135120=CARTESIAN_POINT ( 'NONE',  ( 122.1875000000000000, -5.819803920172573974, 5.819803920172573086 ) ) ;
#135136=CARTESIAN_POINT ( 'NONE',  ( 26.39626352523142927, 4.472830434245840259, -4.472830434245838482 ) ) ;
#135138=CARTESIAN_POINT ( 'NONE',  ( 44.89583333333332149, -2.130196079827427091, 7.949999999999998401 ) ) ;
#135150=ORIENTED_EDGE ( 'NONE', *, *, #52449, .T. ) ;
#135167=CARTESIAN_POINT ( 'NONE',  ( 114.7500000000000000, -9.735942053221458872E-16, 7.950000000000000178 ) ) ;
#135188=CARTESIAN_POINT ( 'NONE',  ( 58.68293019189811588, -1.637169565754159173, -6.109999999999999432 ) ) ;
#135211=CARTESIAN_POINT ( 'NONE',  ( 71.39169371712955581, 2.130196079827421762, 7.950000000000001066 ) ) ;
#135216=CARTESIAN_POINT ( 'NONE',  ( 74.50000000000000000, 0.000000000000000000, -7.950000000000000178 ) ) ;
#135224=CARTESIAN_POINT ( 'NONE',  ( 66.50043019189810423, -3.055000000000002380, 5.291415217122920289 ) ) ;
#135227=EDGE_LOOP ( 'NONE', ( #45587, #69543, #49964, #9023 ) ) ;
#135242=CARTESIAN_POINT ( 'NONE',  ( 51.62543019189811133, 5.291415217122919401, 3.055000000000002824 ) ) ;
#135249=CARTESIAN_POINT ( 'NONE',  ( 53.79166666666667140, 3.975000000000003642, -6.884901960086285300 ) ) ;
#135258=VECTOR ( 'NONE', #45203, 1000.000000000000000 ) ;
#135277=CARTESIAN_POINT ( 'NONE',  ( 102.4329301918980946, 1.637169565754156508, 6.110000000000000320 ) ) ;
#135281=DIRECTION ( 'NONE',  ( -1.000000000000000000, -0.000000000000000000, -0.000000000000000000 ) ) ;
#135300=ORIENTED_EDGE ( 'NONE', *, *, #64308, .F. ) ;
#135302=CARTESIAN_POINT ( 'NONE',  ( 53.22959685856476852, -6.110000000000000320, -1.637169565754161393 ) ) ;
#135305=CARTESIAN_POINT ( 'NONE',  ( 93.04209685856476142, 5.291415217122923842, -3.054999999999996163 ) ) ;
#135317=CARTESIAN_POINT ( 'NONE',  ( 125.4745968585647944, 1.637169565754164280, -6.109999999999997655 ) ) ;
#135374=CARTESIAN_POINT ( 'NONE',  ( 106.5375270504628844, -9.735942053221456900E-16, 7.949999999999998401 ) ) ;
#135391=CARTESIAN_POINT ( 'NONE',  ( 90.27126352523143282, 4.472830434245839371, 4.472830434245842035 ) ) ;
#135415=CARTESIAN_POINT ( 'NONE',  ( 78.60459685856477563, 1.637169565754164946, -6.109999999999999432 ) ) ;
#135422=CARTESIAN_POINT ( 'NONE',  ( 104.1041666666666572, 2.130196079827460398, 7.949999999999981526 ) ) ;
#135426=CARTESIAN_POINT ( 'NONE',  ( 78.95376352523145158, -6.109999999999998543, -3.741295971395162543E-16 ) ) ;
#135471=CARTESIAN_POINT ( 'NONE',  ( 115.6462635252314328, -4.472830434245840259, 4.472830434245838482 ) ) ;
#135498=CARTESIAN_POINT ( 'NONE',  ( 10.32500000000000107, -8.432637487761466488, 4.375000000000001776 ) ) ;
#135518=VERTEX_POINT ( 'NONE', #86004 ) ;
#135549=CARTESIAN_POINT ( 'NONE',  ( 88.64583333333334281, 2.130196079827431976, -7.949999999999999289 ) ) ;
#135556=CARTESIAN_POINT ( 'NONE',  ( 10.61825861377528035, 8.432637487761462936, 4.375000000000001776 ) ) ;
#135561=CARTESIAN_POINT ( 'NONE',  ( 126.4161154897344943, 7.034615505666292457, -0.2322217439817755857 ) ) ;
#135566=CARTESIAN_POINT ( 'NONE',  ( 27.00000000000000711, 5.307397310025502080, 4.669168585031851393 ) ) ;
#135577=CARTESIAN_POINT ( 'NONE',  ( 114.4795968585647614, 6.109999999999999432, 1.637169565754164280 ) ) ;
#135586=CARTESIAN_POINT ( 'NONE',  ( 109.1412635252314374, 4.472830434245836706, 4.472830434245840259 ) ) ;
#135592=ORIENTED_EDGE ( 'NONE', *, *, #108429, .T. ) ;
#135596=CARTESIAN_POINT ( 'NONE',  ( 29.22459685856478018, -1.637169565754160949, 6.109999999999997655 ) ) ;
#135604=CARTESIAN_POINT ( 'NONE',  ( 78.82919371712957002, -3.975000000000001865, 6.884901960086284411 ) ) ;
#135623=EDGE_CURVE ( 'NONE', #67893, #135518, #32345, .T. ) ;
#135625=CARTESIAN_POINT ( 'NONE',  ( 39.72459685856477307, -1.637169565754160949, 6.109999999999997655 ) ) ;
#135659=CARTESIAN_POINT ( 'NONE',  ( 111.9120968585647944, 5.291415217122922066, -3.054999999999995275 ) ) ;
#135662=VECTOR ( 'NONE', #93653, 1000.000000000000000 ) ;
#135708=CARTESIAN_POINT ( 'NONE',  ( 118.8333333333333286, -6.884901960086287964, 3.974999999999998312 ) ) ;
#135710=ORIENTED_EDGE ( 'NONE', *, *, #38464, .F. ) ;
#135719=CARTESIAN_POINT ( 'NONE',  ( 114.4795968585647614, 6.109999999999999432, 1.637169565754164280 ) ) ;
#135729=CARTESIAN_POINT ( 'NONE',  ( 48.05836038379621300, -7.949999999999997513, -2.130196079827425759 ) ) ;
#135736=CARTESIAN_POINT ( 'NONE',  ( 34.83333333333332860, -6.884901960086287964, 3.974999999999998312 ) ) ;
#135746=CARTESIAN_POINT ( 'NONE',  ( 39.95876352523143282, 0.000000000000000000, -6.110000000000001208 ) ) ;
#135759=CARTESIAN_POINT ( 'NONE',  ( 39.74586038379622721, 3.974999999999996980, 6.884901960086287964 ) ) ;
#135766=CARTESIAN_POINT ( 'NONE',  ( 59.12043019189810877, 3.055000000000001936, -5.291415217122916737 ) ) ;
#135782=EDGE_CURVE ( 'NONE', #54290, #75139, #76258, .T. ) ;
#135793=CARTESIAN_POINT ( 'NONE',  ( 63.05793019189810877, 6.110000000000000320, -1.637169565754156064 ) ) ;
#135809=VERTEX_POINT ( 'NONE', #47550 ) ;
#135821=EDGE_CURVE ( 'NONE', #49011, #92088, #101218, .T. ) ;
#135838=EDGE_CURVE ( 'NONE', #46474, #77939, #58428, .T. ) ;
#135848=EDGE_CURVE ( 'NONE', #74997, #68687, #64046, .T. ) ;
#135870=CARTESIAN_POINT ( 'NONE',  ( 51.68293019189811588, -1.637169565754159173, -6.109999999999999432 ) ) ;
#135891=CARTESIAN_POINT ( 'NONE',  ( 75.62086038379622721, -6.884901960086286188, 3.974999999999997424 ) ) ;
#135896=CARTESIAN_POINT ( 'NONE',  ( 64.00000000000000000, 0.000000000000000000, -7.950000000000000178 ) ) ;
#135900=AXIS2_PLACEMENT_3D ( 'NONE', #14053, #47467, #33708 ) ;
#135906=CARTESIAN_POINT ( 'NONE',  ( 65.91709685856477563, 3.054999999999998828, 5.291415217122922066 ) ) ;
#135929=DIRECTION ( 'NONE',  ( -1.000000000000000000, -0.000000000000000000, -0.000000000000000000 ) ) ;
#135932=ORIENTED_EDGE ( 'NONE', *, *, #71435, .T. ) ;
#135955=CARTESIAN_POINT ( 'NONE',  ( 96.16209685856478018, -5.291415217122919401, 3.054999999999997939 ) ) ;
#135970=CARTESIAN_POINT ( 'NONE',  ( 68.81250000000000000, 5.819803920172571310, 5.819803920172576639 ) ) ;
#135982=CARTESIAN_POINT ( 'NONE',  ( 52.93793019189809712, -6.110000000000001208, 1.637169565754158951 ) ) ;
#135998=CARTESIAN_POINT ( 'NONE',  ( 125.0370968585647944, -3.054999999999999272, -5.291415217122919401 ) ) ;
#136027=CARTESIAN_POINT ( 'NONE',  ( 80.77083333333331439, -7.949999999999998401, -2.130196079827426203 ) ) ;
#136041=ORIENTED_EDGE ( 'NONE', *, *, #12988, .F. ) ;
#136054=CARTESIAN_POINT ( 'NONE',  ( 104.3500270504628844, -5.819803920172572198, -5.819803920172572198 ) ) ;
#136070=CARTESIAN_POINT ( 'NONE',  ( 91.58376352523144703, -6.110000000000001208, -3.741295971395164515E-16 ) ) ;
#136092=CARTESIAN_POINT ( 'NONE',  ( 85.02126352523144703, -4.472830434245839371, -4.472830434245840259 ) ) ;
#136104=CARTESIAN_POINT ( 'NONE',  ( 77.34959685856478018, 6.109999999999996767, 1.637169565754163836 ) ) ;
#136122=ORIENTED_EDGE ( 'NONE', *, *, #83237, .T. ) ;
#136157=CARTESIAN_POINT ( 'NONE',  ( 119.5837635252314470, -6.110000000000001208, -3.741295971395164515E-16 ) ) ;
#136163=CARTESIAN_POINT ( 'NONE',  ( 0.000000000000000000, 0.000000000000000000, 0.000000000000000000 ) ) ;
#136188=CARTESIAN_POINT ( 'NONE',  ( 98.22502705046288440, 5.819803920172573974, -5.819803920172573086 ) ) ;
#136212=CARTESIAN_POINT ( 'NONE',  ( 106.0000000000000000, 0.000000000000000000, -7.950000000000000178 ) ) ;
#136218=CARTESIAN_POINT ( 'NONE',  ( 127.2458603837962272, 3.974999999999996980, 6.884901960086287964 ) ) ;
#136232=CARTESIAN_POINT ( 'NONE',  ( 92.43749999999998579, 5.819803920172573974, -5.819803920172572198 ) ) ;
#136238=CARTESIAN_POINT ( 'NONE',  ( 0.000000000000000000, 0.000000000000000000, 0.000000000000000000 ) ) ;
#136246=CARTESIAN_POINT ( 'NONE',  ( 126.9643883377496962, 2.362378534332376212, 6.061514835086926567 ) ) ;
#136261=CARTESIAN_POINT ( 'NONE',  ( 115.0629301918981042, 1.637169565754157174, 6.110000000000002984 ) ) ;
#136272=CARTESIAN_POINT ( 'NONE',  ( 102.7245968585647802, -1.637169565754160949, 6.109999999999997655 ) ) ;
#136317=CARTESIAN_POINT ( 'NONE',  ( 42.05793019189811588, 6.110000000000000320, -1.637169565754156064 ) ) ;
#136355=CARTESIAN_POINT ( 'NONE',  ( 98.64126352523145158, 4.472830434245837594, 4.472830434245841147 ) ) ;
#136396=CARTESIAN_POINT ( 'NONE',  ( 126.4628116846214851, -6.884920636358014434, -1.229062542668005742 ) ) ;
#136402=CARTESIAN_POINT ( 'NONE',  ( 118.5416666666666714, -3.975000000000002753, 6.884901960086286188 ) ) ;
#136412=CARTESIAN_POINT ( 'NONE',  ( 113.1670968585647756, -3.055000000000000160, -5.291415217122921177 ) ) ;
#136424=CARTESIAN_POINT ( 'NONE',  ( 35.51669371712954870, 7.950000000000001066, -2.130196079827421318 ) ) ;
#136428=CARTESIAN_POINT ( 'NONE',  ( 40.22916666666666430, 7.950000000000001954, -2.130196079827421762 ) ) ;
#136438=CARTESIAN_POINT ( 'NONE',  ( 31.35459685856476497, -1.637169565754161615, 6.110000000000000320 ) ) ;
#136458=CARTESIAN_POINT ( 'NONE',  ( 44.97459685856478018, 1.637169565754164058, -6.109999999999996767 ) ) ;
#136460=EDGE_CURVE ( 'NONE', #87171, #93941, #762, .T. ) ;
#136489=VERTEX_POINT ( 'NONE', #34866 ) ;
#136491=CARTESIAN_POINT ( 'NONE',  ( 61.59959685856478018, -6.109999999999997655, -1.637169565754160283 ) ) ;
#136499=CARTESIAN_POINT ( 'NONE',  ( 34.24999999999998579, -9.735942053221458872E-16, 7.950000000000000178 ) ) ;
#136562=CARTESIAN_POINT ( 'NONE',  ( 46.43293019189811588, 1.637169565754156730, 6.110000000000001208 ) ) ;
#136589=CARTESIAN_POINT ( 'NONE',  ( 79.26669371712955581, -7.949999999999999289, 2.130196079827424427 ) ) ;
#136595=CARTESIAN_POINT ( 'NONE',  ( 60.79166666666665719, 3.975000000000003642, -6.884901960086285300 ) ) ;
#136605=CARTESIAN_POINT ( 'NONE',  ( 54.83376352523143282, 6.110000000000001208, 1.122388791418549305E-15 ) ) ;
#136606=FACE_OUTER_BOUND ( 'NONE', #63062, .T. ) ;
#136631=CARTESIAN_POINT ( 'NONE',  ( 71.68336038379621300, -2.130196079827426203, 7.949999999999996625 ) ) ;
#136660=CARTESIAN_POINT ( 'NONE',  ( 93.39126352523143737, -4.472830434245838482, -4.472830434245838482 ) ) ;
#136684=ORIENTED_EDGE ( 'NONE', *, *, #4728, .T. ) ;
#136687=CARTESIAN_POINT ( 'NONE',  ( 42.43793019189809712, -6.110000000000001208, 1.637169565754158951 ) ) ;
#136723=LINE ( 'NONE', #105515, #116145 ) ;
#136733=CARTESIAN_POINT ( 'NONE',  ( 7.430803446455462868, 8.913522578092118565, 3.292921844800691389 ) ) ;
#136761=CARTESIAN_POINT ( 'NONE',  ( 100.9958603837962272, -3.974999999999998312, -6.884901960086286188 ) ) ;
#136783=CARTESIAN_POINT ( 'NONE',  ( 81.08376352523144703, -6.110000000000001208, -3.741295971395164515E-16 ) ) ;
#136803=CARTESIAN_POINT ( 'NONE',  ( 0.000000000000000000, 0.000000000000000000, 0.000000000000000000 ) ) ;
#136807=CARTESIAN_POINT ( 'NONE',  ( 86.62543019189811844, 5.291415217122919401, 3.055000000000002824 ) ) ;
#136816=CARTESIAN_POINT ( 'NONE',  ( 103.8125000000000000, 5.819803920172571310, 5.819803920172576639 ) ) ;
#136818=CARTESIAN_POINT ( 'NONE',  ( 76.47459685856476597, 1.637169565754164058, -6.109999999999996767 ) ) ;
#136836=ORIENTED_EDGE ( 'NONE', *, *, #38363, .T. ) ;
#136866=CARTESIAN_POINT ( 'NONE',  ( 70.87543019189810423, -5.291415217122920289, -3.055000000000001492 ) ) ;
#136871=CARTESIAN_POINT ( 'NONE',  ( 107.6254301918981042, 5.291415217122919401, 3.055000000000002824 ) ) ;
#136876=CARTESIAN_POINT ( 'NONE',  ( 87.28752705046288440, 0.000000000000000000, -7.949999999999998401 ) ) ;
#136878=DIRECTION ( 'NONE',  ( 0.000000000000000000, 0.000000000000000000, 1.000000000000000000 ) ) ;
#136906=CARTESIAN_POINT ( 'NONE',  ( 14.55628666580615693, -9.434540764276121649, -1.149137486816687481 ) ) ;
#136939=CARTESIAN_POINT ( 'NONE',  ( 126.9541937171295700, 6.884901960086283523, 3.975000000000002753 ) ) ;
#136958=CARTESIAN_POINT ( 'NONE',  ( 96.08333333333332860, 6.884901960086290629, -3.974999999999994316 ) ) ;
#136967=CARTESIAN_POINT ( 'NONE',  ( 14.47215708364651121, 9.396720740463704757, 1.422595638764767134 ) ) ;
#136974=CARTESIAN_POINT ( 'NONE',  ( 125.5000000000000568, -3.922572014496796822, -6.914906274931464480 ) ) ;
#136987=CARTESIAN_POINT ( 'NONE',  ( 107.9170968585647756, 3.054999999999998828, 5.291415217122922066 ) ) ;
#136996=VECTOR ( 'NONE', #118456, 1000.000000000000000 ) ;
#136997=CARTESIAN_POINT ( 'NONE',  ( 102.2870968585647802, 3.054999999999997495, 5.291415217122919401 ) ) ;
#137043=CARTESIAN_POINT ( 'NONE',  ( 38.12043019189811588, 3.055000000000001936, -5.291415217122916737 ) ) ;
#137055=CIRCLE ( 'NONE', #23632, 9.500000000000000000 ) ;
#137067=STYLED_ITEM ( 'NONE', ( #26814 ), #70809 ) ;
#137083=CARTESIAN_POINT ( 'NONE',  ( 104.3287635252314658, 0.000000000000000000, -6.109999999999999432 ) ) ;
#137136=CARTESIAN_POINT ( 'NONE',  ( 118.2500000000000000, -9.735942053221458872E-16, 7.950000000000000178 ) ) ;
#137149=CARTESIAN_POINT ( 'NONE',  ( 108.6462635252314186, -4.472830434245840259, 4.472830434245839371 ) ) ;
#137160=CARTESIAN_POINT ( 'NONE',  ( 41.64169371712954870, -2.130196079827424871, -7.949999999999999289 ) ) ;
#137166=CARTESIAN_POINT ( 'NONE',  ( 33.08333333333332860, 6.884901960086290629, -3.974999999999994316 ) ) ;
#137181=CARTESIAN_POINT ( 'NONE',  ( 31.93793019189809712, -6.110000000000001208, 1.637169565754158951 ) ) ;
#137202=CARTESIAN_POINT ( 'NONE',  ( 44.24543019189810877, -5.291415217122918513, -3.055000000000000160 ) ) ;
#137204=CARTESIAN_POINT ( 'NONE',  ( 125.2500000000000000, -9.735942053221458872E-16, 7.950000000000000178 ) ) ;
#137210=AXIS2_PLACEMENT_3D ( 'NONE', #93889, #17056, #50405 ) ;
#137227=CARTESIAN_POINT ( 'NONE',  ( 64.07876352523145158, -7.482591942790325086E-16, 6.109999999999998543 ) ) ;
#137247=ORIENTED_EDGE ( 'NONE', *, *, #54848, .F. ) ;
#137266=ORIENTED_EDGE ( 'NONE', *, *, #14540, .F. ) ;
#137272=CARTESIAN_POINT ( 'NONE',  ( 108.7708333333333286, -7.949999999999998401, -2.130196079827426203 ) ) ;
#137273=ADVANCED_FACE ( 'NONE', ( #41625 ), #96686, .T. ) ;
#137306=CARTESIAN_POINT ( 'NONE',  ( 42.93293019189812298, 1.637169565754156730, 6.110000000000001208 ) ) ;
#137333=CARTESIAN_POINT ( 'NONE',  ( 64.53752705046289861, -9.735942053221456900E-16, 7.949999999999998401 ) ) ;
#137337=CARTESIAN_POINT ( 'NONE',  ( 67.20833333333332860, -3.974999999999999201, -6.884901960086287964 ) ) ;
#137348=CARTESIAN_POINT ( 'NONE',  ( 60.95876352523143993, 0.000000000000000000, -6.110000000000001208 ) ) ;
#137367=ADVANCED_FACE ( 'NONE', ( #77839 ), #90874, .T. ) ;
#137394=SHAPE_DEFINITION_REPRESENTATION ( #38839, #58954 ) ;
#137398=CARTESIAN_POINT ( 'NONE',  ( 97.03709685856479439, -3.054999999999998828, -5.291415217122919401 ) ) ;
#137420=ORIENTED_EDGE ( 'NONE', *, *, #83332, .F. ) ;
#137424=CARTESIAN_POINT ( 'NONE',  ( 47.25043019189810423, 3.055000000000002824, -5.291415217122919401 ) ) ;
#137469=CARTESIAN_POINT ( 'NONE',  ( 95.45419371712957002, 6.884901960086283523, 3.975000000000002753 ) ) ;
#137474=CARTESIAN_POINT ( 'NONE',  ( 70.49543019189810877, 5.291415217122917625, 3.055000000000002380 ) ) ;
#137499=CARTESIAN_POINT ( 'NONE',  ( 98.22502705046289861, 5.819803920172573086, -5.819803920172572198 ) ) ;
#137515=CARTESIAN_POINT ( 'NONE',  ( 88.66709685856477563, -3.055000000000000160, -5.291415217122921177 ) ) ;
#137535=ORIENTED_EDGE ( 'NONE', *, *, #115701, .T. ) ;
#137538=CARTESIAN_POINT ( 'NONE',  ( 81.37543019189810423, -5.291415217122920289, -3.055000000000001492 ) ) ;
#137584=ORIENTED_EDGE ( 'NONE', *, *, #44311, .T. ) ;
#137593=CARTESIAN_POINT ( 'NONE',  ( 71.16709685856477563, -3.055000000000000160, -5.291415217122921177 ) ) ;
#137602=CARTESIAN_POINT ( 'NONE',  ( 105.8754301918981042, -5.291415217122920289, -3.055000000000001492 ) ) ;
#137648=( BOUNDED_CURVE ( )  B_SPLINE_CURVE ( 2, ( #104854, #27279, #71534, #115689, #16390, #60691, #91830, #5519, #83114, #127316, #72286, #17140, #105549 ),
 .UNSPECIFIED., .F., .F. ) 
 B_SPLINE_CURVE_WITH_KNOTS ( ( 3, 2, 2, 2, 2, 2, 3 ),
 ( 0.5166666666666667185, 0.5194444444444444864, 0.5222222222222222543, 0.5250000000000001332, 0.5277777777777779011, 0.5305555555555556690, 0.5333333333333334370 ),
 .UNSPECIFIED. ) 
 CURVE ( )  GEOMETRIC_REPRESENTATION_ITEM ( )  RATIONAL_B_SPLINE_CURVE ( ( 1.000000000000000000, 0.9659258262890683122, 1.000000000000000000, 0.9659258262890683122, 1.000000000000000000, 0.9659258262890683122, 1.000000000000000000, 0.9659258262890683122, 1.000000000000000000, 0.9659258262890683122, 1.000000000000000000, 0.9659258262890669799, 1.000000000000001332 ) ) 
 REPRESENTATION_ITEM ( '' )  );
#137659=LINE ( 'NONE', #38333, #70249 ) ;
#137676=CARTESIAN_POINT ( 'NONE',  ( 29.51626352523143737, -4.472830434245839371, 4.472830434245839371 ) ) ;
#137691=CARTESIAN_POINT ( 'NONE',  ( 89.08333333333332860, 6.884901960086290629, -3.974999999999994316 ) ) ;
#137702=CARTESIAN_POINT ( 'NONE',  ( 126.1800681914572522, 6.167271031922632041, -3.881961135379007111 ) ) ;
#137716=CARTESIAN_POINT ( 'NONE',  ( 111.5629301918981184, 1.637169565754157174, 6.110000000000002984 ) ) ;
#137725=CARTESIAN_POINT ( 'NONE',  ( 106.2245968585647802, -1.637169565754160949, 6.109999999999997655 ) ) ;
#137773=CARTESIAN_POINT ( 'NONE',  ( 36.95376352523144448, -6.109999999999998543, -3.741295971395162543E-16 ) ) ;
#137810=CARTESIAN_POINT ( 'NONE',  ( 98.93293019189812298, 1.637169565754156730, 6.110000000000001208 ) ) ;
#137855=CARTESIAN_POINT ( 'NONE',  ( 26.19059147121573972, 3.175000000000004263, -5.499261314031186565 ) ) ;
#137861=CARTESIAN_POINT ( 'NONE',  ( 117.3750000000000000, 7.950000000000000178, 1.460391307983218535E-15 ) ) ;
#137873=CARTESIAN_POINT ( 'NONE',  ( 112.8754301918981042, -5.291415217122920289, -3.055000000000001492 ) ) ;
#137879=CARTESIAN_POINT ( 'NONE',  ( 82.18336038379619879, -2.130196079827426203, 7.949999999999996625 ) ) ;
#137882=CARTESIAN_POINT ( 'NONE',  ( 42.37086038379622721, 6.884901960086289741, -3.974999999999993427 ) ) ;
#137887=CARTESIAN_POINT ( 'NONE',  ( 36.29166666666666430, 3.975000000000003642, -6.884901960086285300 ) ) ;
#137891=ORIENTED_EDGE ( 'NONE', *, *, #116290, .F. ) ;
#137896=CARTESIAN_POINT ( 'NONE',  ( 128.0995968585647802, -6.109999999999997655, -1.637169565754160283 ) ) ;
#137907=CARTESIAN_POINT ( 'NONE',  ( 55.27126352523143282, 4.472830434245839371, 4.472830434245842035 ) ) ;
#137914=CARTESIAN_POINT ( 'NONE',  ( 50.07876352523145158, -7.482591942790325086E-16, 6.109999999999998543 ) ) ;
#137945=CARTESIAN_POINT ( 'NONE',  ( 66.26626352523145158, 4.472830434245838482, -4.472830434245837594 ) ) ;
#138015=CARTESIAN_POINT ( 'NONE',  ( 44.39126352523143737, -4.472830434245839371, -4.472830434245839371 ) ) ;
#138037=CARTESIAN_POINT ( 'NONE',  ( 65.12086038379621300, -6.884901960086286188, 3.974999999999997424 ) ) ;
#138038=AXIS2_PLACEMENT_3D ( 'NONE', #136238, #36926, #81175 ) ;
#138042=CARTESIAN_POINT ( 'NONE',  ( 67.35416666666664298, -2.130196079827425315, -7.950000000000001066 ) ) ;
#138046=LINE ( 'NONE', #40701, #89102 ) ;
#138052=CARTESIAN_POINT ( 'NONE',  ( 54.10459685856476852, 1.637169565754164946, -6.109999999999999432 ) ) ;
#138066=CYLINDRICAL_SURFACE ( 'NONE', #31549, 7.950000000000000178 ) ;
#138075=CARTESIAN_POINT ( 'NONE',  ( 110.4750270504628702, -5.819803920172573086, 5.819803920172573086 ) ) ;
#138080=FACE_OUTER_BOUND ( 'NONE', #120652, .T. ) ;
#138083=( BOUNDED_CURVE ( )  B_SPLINE_CURVE ( 2, ( #30951, #75872, #119339, #11278, #109195, #9879, #55552, #54149, #32363, #21489, #98339, #76607, #88905 ),
 .UNSPECIFIED., .F., .F. ) 
 B_SPLINE_CURVE_WITH_KNOTS ( ( 3, 2, 2, 2, 2, 2, 3 ),
 ( 0.6166666666666666963, 0.6194444444444444642, 0.6222222222222222321, 0.6250000000000000000, 0.6277777777777777679, 0.6305555555555555358, 0.6333333333333333037 ),
 .UNSPECIFIED. ) 
 CURVE ( )  GEOMETRIC_REPRESENTATION_ITEM ( )  RATIONAL_B_SPLINE_CURVE ( ( 1.000000000000000000, 0.9659258262890683122, 1.000000000000000000, 0.9659258262890683122, 1.000000000000000000, 0.9659258262890683122, 1.000000000000000000, 0.9659258262890683122, 1.000000000000000000, 0.9659258262890683122, 1.000000000000000000, 0.9659258262890683122, 1.000000000000000000 ) ) 
 REPRESENTATION_ITEM ( '' )  );
#138087=CARTESIAN_POINT ( 'NONE',  ( 62.35002705046287730, -5.819803920172573086, -5.819803920172573086 ) ) ;
#138103=CARTESIAN_POINT ( 'NONE',  ( 95.72459685856476597, -1.637169565754160949, 6.109999999999997655 ) ) ;
#138132=CARTESIAN_POINT ( 'NONE',  ( 48.41709685856476852, 3.054999999999998828, 5.291415217122922066 ) ) ;
#138152=FACE_OUTER_BOUND ( 'NONE', #2712, .T. ) ;
#138178=CARTESIAN_POINT ( 'NONE',  ( 94.57919371712955581, 3.975000000000002753, -6.884901960086283523 ) ) ;
#138184=CARTESIAN_POINT ( 'NONE',  ( 76.76626352523142316, 4.472830434245839371, -4.472830434245839371 ) ) ;
#138186=FACE_OUTER_BOUND ( 'NONE', #5207, .T. ) ;
#138206=CARTESIAN_POINT ( 'NONE',  ( 90.64169371712954160, -2.130196079827424871, -7.949999999999999289 ) ) ;
#138220=CARTESIAN_POINT ( 'NONE',  ( 83.41709685856477563, 3.054999999999998828, 5.291415217122922066 ) ) ;
#138244=CARTESIAN_POINT ( 'NONE',  ( 76.70876352523144703, -7.482591942790329030E-16, 6.110000000000001208 ) ) ;
#138258=CARTESIAN_POINT ( 'NONE',  ( 34.20419371712955581, -6.884901960086285300, -3.975000000000000089 ) ) ;
#138270=CARTESIAN_POINT ( 'NONE',  ( 53.01669371712955581, 7.950000000000000178, -2.130196079827421318 ) ) ;
#138303=CARTESIAN_POINT ( 'NONE',  ( 77.29209685856477563, -5.291415217122921177, 3.054999999999999272 ) ) ;
#138308=CARTESIAN_POINT ( 'NONE',  ( 108.3545968585647614, -1.637169565754161615, 6.110000000000000320 ) ) ;
#138338=CARTESIAN_POINT ( 'NONE',  ( 90.64169371712954160, -2.130196079827424871, -7.949999999999998401 ) ) ;
#138370=CARTESIAN_POINT ( 'NONE',  ( 117.9125270504628986, -7.949999999999998401, -4.867971026610728450E-16 ) ) ;
#138384=CARTESIAN_POINT ( 'NONE',  ( 79.31250000000000000, 5.819803920172571310, 5.819803920172575751 ) ) ;
#138414=CARTESIAN_POINT ( 'NONE',  ( 104.5629301918981184, 1.637169565754157174, 6.110000000000002984 ) ) ;
#138421=ORIENTED_EDGE ( 'NONE', *, *, #112470, .T. ) ;
#138426=CARTESIAN_POINT ( 'NONE',  ( 107.0995968585648086, -6.109999999999997655, -1.637169565754160283 ) ) ;
#138452=ADVANCED_FACE ( 'NONE', ( #136606, #13386 ), #38739, .T. ) ;
#138453=CARTESIAN_POINT ( 'NONE',  ( 113.8079301918981088, -6.109999999999998543, 1.637169565754158507 ) ) ;
#138479=CARTESIAN_POINT ( 'NONE',  ( 30.09959685856477662, -6.109999999999997655, -1.637169565754160283 ) ) ;
#138491=CARTESIAN_POINT ( 'NONE',  ( 76.25000000000000000, -9.735942053221458872E-16, 7.950000000000000178 ) ) ;
#138499=ORIENTED_EDGE ( 'NONE', *, *, #15485, .T. ) ;
#138512=CARTESIAN_POINT ( 'NONE',  ( 105.3495968585647944, 6.109999999999997655, 1.637169565754163836 ) ) ;
#138528=EDGE_CURVE ( 'NONE', #44417, #38530, #49648, .T. ) ;
#138562=CARTESIAN_POINT ( 'NONE',  ( 110.2291666666666714, 7.950000000000001954, -2.130196079827421762 ) ) ;
#138577=CARTESIAN_POINT ( 'NONE',  ( 114.6254301918981042, 5.291415217122919401, 3.055000000000002824 ) ) ;
#138586=CARTESIAN_POINT ( 'NONE',  ( 38.43336038379620589, 2.130196079827431532, -7.949999999999997513 ) ) ;
#138591=ORIENTED_EDGE ( 'NONE', *, *, #31583, .T. ) ;
#138593=CARTESIAN_POINT ( 'NONE',  ( 33.22916666666665719, 7.950000000000001954, -2.130196079827421762 ) ) ;
#138607=CARTESIAN_POINT ( 'NONE',  ( 32.08376352523143993, -6.110000000000001208, -3.741295971395164515E-16 ) ) ;
#138616=CARTESIAN_POINT ( 'NONE',  ( 64.00000000000000000, 0.000000000000000000, -7.950000000000000178 ) ) ;
#138618=CARTESIAN_POINT ( 'NONE',  ( 50.89626352523143993, 4.472830434245840259, -4.472830434245839371 ) ) ;
#138627=CARTESIAN_POINT ( 'NONE',  ( 47.89126352523143737, -4.472830434245839371, -4.472830434245839371 ) ) ;
#138660=CARTESIAN_POINT ( 'NONE',  ( 63.64126352523144448, 4.472830434245835818, 4.472830434245840259 ) ) ;
#138662=DIRECTION ( 'NONE',  ( 0.000000000000000000, 0.000000000000000000, 1.000000000000000000 ) ) ;
#138669=CARTESIAN_POINT ( 'NONE',  ( 35.41666666666666430, -6.884901960086287076, -3.975000000000000977 ) ) ;
#138689=CARTESIAN_POINT ( 'NONE',  ( 29.87500000000000000, 7.950000000000000178, 1.460391307983218535E-15 ) ) ;
#138712=DIRECTION ( 'NONE',  ( -1.000000000000000000, -0.000000000000000000, -0.000000000000000000 ) ) ;
#138734=CARTESIAN_POINT ( 'NONE',  ( 43.80793019189810877, -6.109999999999999432, 1.637169565754158507 ) ) ;
#138737=CARTESIAN_POINT ( 'NONE',  ( 31.43336038379622366, 2.130196079827431532, -7.949999999999996625 ) ) ;
#138759=CARTESIAN_POINT ( 'NONE',  ( 65.85002705046288440, -5.819803920172572198, -5.819803920172572198 ) ) ;
#138764=CARTESIAN_POINT ( 'NONE',  ( 62.54166666666666430, -3.975000000000002753, 6.884901960086286188 ) ) ;
#138776=CARTESIAN_POINT ( 'NONE',  ( 55.70876352523143282, -7.482591942790329030E-16, 6.110000000000001208 ) ) ;
#138782=AXIS2_PLACEMENT_3D ( 'NONE', #1744, #38015, #48161 ) ;
#138829=CARTESIAN_POINT ( 'NONE',  ( 92.07876352523145158, -7.482591942790325086E-16, 6.109999999999998543 ) ) ;
#138856=CARTESIAN_POINT ( 'NONE',  ( 40.68793019189811133, 6.110000000000002984, -1.637169565754156730 ) ) ;
#138898=CARTESIAN_POINT ( 'NONE',  ( 95.50000000000000000, 0.000000000000000000, -7.950000000000000178 ) ) ;
#138908=CARTESIAN_POINT ( 'NONE',  ( 76.32876352523145158, 0.000000000000000000, -6.109999999999999432 ) ) ;
#138928=CLOSED_SHELL ( 'NONE', ( #85908, #87219, #124334, #137367, #142677, #4446, #17831, #78953, #65850, #61288, #19000, #86701, #100539, #58688, #141866, #22071, #13097, #94684, #92682, #29445, #123605, #124041, #94396, #31608, #75928, #111728, #89958, #90577, #38755, #2275, #49831, #62442, #67274, #56047, #25138, #7080, #24951, #137273, #121572, #56986, #109933, #2957, #96325, #45085, #143442, #133411, #60067, #81849, #23415, #56976, #64122, #75942, #32378, #46297, #109292, #4835, #113684, #24776, #128267, #73004, #61469, #71541, #20896, #133140, #29561, #42337, #94385, #85360, #112298, #97082, #132196, #138452, #14749, #132396, #142841, #55171, #31085, #112888, #23266, #119162, #69094, #5358, #107662, #41295, #33562, #45052 ) ) ;
#138930=CARTESIAN_POINT ( 'NONE',  ( 89.91252705046289861, -7.949999999999998401, -4.867971026610728450E-16 ) ) ;
#138946=CARTESIAN_POINT ( 'NONE',  ( 85.02126352523144703, -4.472830434245839371, -4.472830434245840259 ) ) ;
#138965=CARTESIAN_POINT ( 'NONE',  ( 59.77083333333332860, -7.949999999999998401, -2.130196079827426203 ) ) ;
#138968=CARTESIAN_POINT ( 'NONE',  ( 74.81293019189809002, -1.637169565754159617, -6.110000000000001208 ) ) ;
#138981=CIRCLE ( 'NONE', #51013, 6.350000000000008527 ) ;
#138994=EDGE_CURVE ( 'NONE', #2806, #37814, #142989, .T. ) ;
#139010=CARTESIAN_POINT ( 'NONE',  ( 27.00000000000000711, -6.919509820621859042, -2.766677502517353116 ) ) ;
#139020=CARTESIAN_POINT ( 'NONE',  ( 69.12543019189809002, 5.291415217122919401, 3.055000000000002824 ) ) ;
#139025=CARTESIAN_POINT ( 'NONE',  ( 111.1254301918981042, 5.291415217122919401, 3.055000000000002824 ) ) ;
#139034=CARTESIAN_POINT ( 'NONE',  ( 77.07919371712957002, 3.975000000000002753, -6.884901960086283523 ) ) ;
#139096=CARTESIAN_POINT ( 'NONE',  ( 124.0375270504628986, -9.735942053221456900E-16, 7.949999999999998401 ) ) ;
#139105=VECTOR ( 'NONE', #95592, 1000.000000000000000 ) ;
#139114=CARTESIAN_POINT ( 'NONE',  ( 85.72916666666664298, 7.950000000000001954, -2.130196079827421762 ) ) ;
#139119=CARTESIAN_POINT ( 'NONE',  ( 31.14169371712956291, -2.130196079827424871, -7.949999999999998401 ) ) ;
#139140=CARTESIAN_POINT ( 'NONE',  ( 100.3337635252314328, 6.110000000000001208, 1.122388791418549305E-15 ) ) ;
#139153=CARTESIAN_POINT ( 'NONE',  ( 90.91209685856478018, 5.291415217122921177, -3.054999999999994831 ) ) ;
#139185=CARTESIAN_POINT ( 'NONE',  ( 115.2662635252314374, 4.472830434245838482, -4.472830434245837594 ) ) ;
#139209=CARTESIAN_POINT ( 'NONE',  ( 27.91209685856478728, 5.291415217122921177, -3.054999999999994831 ) ) ;
#139247=CARTESIAN_POINT ( 'NONE',  ( 98.78709685856479439, 3.054999999999997939, 5.291415217122920289 ) ) ;
#139301=CARTESIAN_POINT ( 'NONE',  ( 110.5208333333333428, 7.949999999999999289, 2.130196079827431532 ) ) ;
#139317=CARTESIAN_POINT ( 'NONE',  ( 101.2087635252314470, -7.482591942790329030E-16, 6.110000000000001208 ) ) ;
#139322=CARTESIAN_POINT ( 'NONE',  ( 82.32919371712955581, -3.975000000000001865, 6.884901960086284411 ) ) ;
#139326=CARTESIAN_POINT ( 'NONE',  ( 38.87086038379622721, 6.884901960086289741, -3.974999999999993427 ) ) ;
#139331=CARTESIAN_POINT ( 'NONE',  ( 127.1670968585647756, -3.055000000000000160, -5.291415217122921177 ) ) ;
#139342=CARTESIAN_POINT ( 'NONE',  ( 122.1204301918981230, 3.055000000000001936, -5.291415217122916737 ) ) ;
#139355=CARTESIAN_POINT ( 'NONE',  ( 47.10459685856477563, 1.637169565754164946, -6.109999999999999432 ) ) ;
#139363=CARTESIAN_POINT ( 'NONE',  ( 50.80793019189810167, -6.109999999999998543, 1.637169565754158063 ) ) ;
#139395=CARTESIAN_POINT ( 'NONE',  ( 52.41209685856478018, 5.291415217122921177, -3.054999999999994831 ) ) ;
#139443=CARTESIAN_POINT ( 'NONE',  ( 109.3541666666666714, -2.130196079827425759, -7.950000000000000178 ) ) ;
#139475=CARTESIAN_POINT ( 'NONE',  ( 43.51626352523143737, -4.472830434245839371, 4.472830434245839371 ) ) ;
#139498=FACE_OUTER_BOUND ( 'NONE', #134995, .T. ) ;
#139501=CARTESIAN_POINT ( 'NONE',  ( 67.16252705046288440, 7.949999999999998401, 1.460391307983218338E-15 ) ) ;
#139505=CARTESIAN_POINT ( 'NONE',  ( 54.66666666666667140, 6.884901960086285300, 3.975000000000003642 ) ) ;
#139512=CARTESIAN_POINT ( 'NONE',  ( 60.08376352523143993, -6.110000000000001208, -3.741295971395164515E-16 ) ) ;
#139525=CARTESIAN_POINT ( 'NONE',  ( 99.68336038379621300, -2.130196079827426203, 7.949999999999996625 ) ) ;
#139537=CARTESIAN_POINT ( 'NONE',  ( 73.99543019189810877, 5.291415217122916737, 3.055000000000001936 ) ) ;
#139545=CARTESIAN_POINT ( 'NONE',  ( 0.000000000000000000, 9.735942053221458872E-16, -7.950000000000000178 ) ) ;
#139557=DIRECTION ( 'NONE',  ( 0.000000000000000000, 0.000000000000000000, 1.000000000000000000 ) ) ;
#139563=CARTESIAN_POINT ( 'NONE',  ( 83.76626352523145158, 4.472830434245838482, -4.472830434245837594 ) ) ;
#139590=CARTESIAN_POINT ( 'NONE',  ( 45.35459685856476142, -1.637169565754161615, 6.110000000000000320 ) ) ;
#139602=DIRECTION ( 'NONE',  ( 0.000000000000000000, 0.000000000000000000, 1.000000000000000000 ) ) ;
#139644=CARTESIAN_POINT ( 'NONE',  ( 72.53709685856478018, -3.054999999999999272, -5.291415217122919401 ) ) ;
#139667=CARTESIAN_POINT ( 'NONE',  ( 95.01669371712955581, 7.950000000000001066, -2.130196079827421318 ) ) ;
#139681=CARTESIAN_POINT ( 'NONE',  ( 88.22959685856474721, -6.110000000000000320, -1.637169565754161393 ) ) ;
#139687=ORIENTED_EDGE ( 'NONE', *, *, #112470, .F. ) ;
#139695=EDGE_CURVE ( 'NONE', #8484, #14445, #73706, .T. ) ;
#139700=VERTEX_POINT ( 'NONE', #8517 ) ;
#139701=CARTESIAN_POINT ( 'NONE',  ( 72.77126352523144703, 4.472830434245839371, 4.472830434245842035 ) ) ;
#139725=CARTESIAN_POINT ( 'NONE',  ( 52.28752705046288440, 0.000000000000000000, -7.949999999999998401 ) ) ;
#139730=VECTOR ( 'NONE', #90364, 1000.000000000000000 ) ;
#139746=CARTESIAN_POINT ( 'NONE',  ( 50.29166666666666430, 3.975000000000003642, -6.884901960086285300 ) ) ;
#139751=VERTEX_POINT ( 'NONE', #99860 ) ;
#139753=CARTESIAN_POINT ( 'NONE',  ( 75.10459685856476142, 1.637169565754164946, -6.109999999999999432 ) ) ;
#139754=ORIENTED_EDGE ( 'NONE', *, *, #63442, .T. ) ;
#139760=CARTESIAN_POINT ( 'NONE',  ( 112.0004301918981042, -3.055000000000002380, 5.291415217122920289 ) ) ;
#139767=EDGE_CURVE ( 'NONE', #85083, #10004, #20753, .T. ) ;
#139770=CARTESIAN_POINT ( 'NONE',  ( 77.66252705046289861, 7.949999999999998401, 1.460391307983218338E-15 ) ) ;
#139793=CARTESIAN_POINT ( 'NONE',  ( 14.11557571622218532, -9.244271043508256014, 2.203030002273714594 ) ) ;
#139807=CARTESIAN_POINT ( 'NONE',  ( 27.70876352523143993, -7.482591942790329030E-16, 6.110000000000001208 ) ) ;
#139830=CARTESIAN_POINT ( 'NONE',  ( 124.4750270504628844, -5.819803920172572198, 5.819803920172572198 ) ) ;
#139844=CARTESIAN_POINT ( 'NONE',  ( 79.16666666666665719, 6.884901960086285300, 3.975000000000003642 ) ) ;
#139847=CARTESIAN_POINT ( 'NONE',  ( 90.78752705046288440, 0.000000000000000000, -7.949999999999998401 ) ) ;
#139865=CARTESIAN_POINT ( 'NONE',  ( 101.3545968585647614, -1.637169565754161615, 6.110000000000000320 ) ) ;
#139874=CARTESIAN_POINT ( 'NONE',  ( 99.80793019189812298, -6.109999999999998543, 1.637169565754158063 ) ) ;
#139877=VERTEX_POINT ( 'NONE', #59253 ) ;
#139919=ORIENTED_EDGE ( 'NONE', *, *, #113563, .F. ) ;
#139922=CARTESIAN_POINT ( 'NONE',  ( 31.99543019189811233, 5.291415217122916737, 3.055000000000001936 ) ) ;
#139933=EDGE_CURVE ( 'NONE', #105597, #69571, #137648, .T. ) ;
#139958=CARTESIAN_POINT ( 'NONE',  ( 90.62043019189810877, 3.055000000000002380, -5.291415217122917625 ) ) ;
#139990=EDGE_CURVE ( 'NONE', #78734, #85083, #141795, .T. ) ;
#139996=CARTESIAN_POINT ( 'NONE',  ( 31.33333333333332504, -6.884901960086287964, 3.974999999999998312 ) ) ;
#140006=CARTESIAN_POINT ( 'NONE',  ( 110.3750000000000000, 7.950000000000000178, 1.460391307983218535E-15 ) ) ;
#140018=CARTESIAN_POINT ( 'NONE',  ( 101.5004301918981042, -3.055000000000002380, 5.291415217122920289 ) ) ;
#140033=CARTESIAN_POINT ( 'NONE',  ( 29.14583333333332504, 2.130196079827431976, -7.949999999999999289 ) ) ;
#140042=CARTESIAN_POINT ( 'NONE',  ( 122.4120968585647802, 5.291415217122921177, -3.054999999999994831 ) ) ;
#140052=CARTESIAN_POINT ( 'NONE',  ( 41.85459685856477563, -1.637169565754161615, 6.110000000000000320 ) ) ;
#140062=CARTESIAN_POINT ( 'NONE',  ( 37.97459685856477307, 1.637169565754164058, -6.109999999999996767 ) ) ;
#140076=CARTESIAN_POINT ( 'NONE',  ( 52.28752705046288440, 0.000000000000000000, -7.949999999999998401 ) ) ;
#140078=CARTESIAN_POINT ( 'NONE',  ( 0.000000000000000000, 9.735942053221458872E-16, -7.950000000000000178 ) ) ;
#140091=CARTESIAN_POINT ( 'NONE',  ( 60.43293019189810877, 1.637169565754156508, 6.110000000000000320 ) ) ;
#140125=CARTESIAN_POINT ( 'NONE',  ( 122.1204301918981230, 3.055000000000002380, -5.291415217122917625 ) ) ;
#140134=CARTESIAN_POINT ( 'NONE',  ( 76.64169371712954160, -2.130196079827424871, -7.949999999999998401 ) ) ;
#140142=ORIENTED_EDGE ( 'NONE', *, *, #54990, .T. ) ;
#140161=CARTESIAN_POINT ( 'NONE',  ( 38.84959685856477307, 6.109999999999997655, 1.637169565754163836 ) ) ;
#140180=CARTESIAN_POINT ( 'NONE',  ( 104.3500270504628844, -5.819803920172573086, -5.819803920172573086 ) ) ;
#140181=CARTESIAN_POINT ( 'NONE',  ( 70.37086038379622721, 6.884901960086289741, -3.974999999999993427 ) ) ;
#140186=CARTESIAN_POINT ( 'NONE',  ( 56.56250000000000711, -5.819803920172572198, -5.819803920172573086 ) ) ;
#140194=CARTESIAN_POINT ( 'NONE',  ( 46.08376352523143993, -6.110000000000001208, -3.741295971395164515E-16 ) ) ;
#140216=ORIENTED_EDGE ( 'NONE', *, *, #26786, .F. ) ;
#140220=CARTESIAN_POINT ( 'NONE',  ( 77.93293019189812298, 1.637169565754156508, 6.110000000000000320 ) ) ;
#140241=CARTESIAN_POINT ( 'NONE',  ( 40.47502705046289151, -5.819803920172573086, 5.819803920172573086 ) ) ;
#140250=CARTESIAN_POINT ( 'NONE',  ( 85.80793019189810877, -6.109999999999998543, 1.637169565754158507 ) ) ;
#140271=CARTESIAN_POINT ( 'NONE',  ( 31.93793019189809712, -6.110000000000001208, 1.637169565754158951 ) ) ;
#140319=CARTESIAN_POINT ( 'NONE',  ( 69.62043019189812298, 3.055000000000002380, -5.291415217122917625 ) ) ;
#140343=CARTESIAN_POINT ( 'NONE',  ( 92.68336038379624142, -2.130196079827426203, 7.949999999999997513 ) ) ;
#140355=CARTESIAN_POINT ( 'NONE',  ( 79.91709685856476142, 3.054999999999998828, 5.291415217122922066 ) ) ;
#140367=CARTESIAN_POINT ( 'NONE',  ( 38.28752705046288440, 0.000000000000000000, -7.949999999999998401 ) ) ;
#140374=CARTESIAN_POINT ( 'NONE',  ( 78.02126352523146124, -4.472830434245839371, -4.472830434245840259 ) ) ;
#140400=CARTESIAN_POINT ( 'NONE',  ( 27.00000000000000355, 0.000000000000000000, 0.000000000000000000 ) ) ;
#140415=CARTESIAN_POINT ( 'NONE',  ( 68.91252705046288440, -7.949999999999998401, -4.867971026610728450E-16 ) ) ;
#140429=CARTESIAN_POINT ( 'NONE',  ( 62.56293019189811133, 1.637169565754157174, 6.110000000000002984 ) ) ;
#140436=CARTESIAN_POINT ( 'NONE',  ( 95.81293019189809002, -1.637169565754159617, -6.110000000000001208 ) ) ;
#140445=VERTEX_POINT ( 'NONE', #108753 ) ;
#140453=CARTESIAN_POINT ( 'NONE',  ( 160.0000000000000000, 0.000000000000000000, 0.000000000000000000 ) ) ;
#140477=CARTESIAN_POINT ( 'NONE',  ( 31.35459685856476497, -1.637169565754161615, 6.110000000000000320 ) ) ;
#140490=LINE ( 'NONE', #62974, #132344 ) ;
#140495=CARTESIAN_POINT ( 'NONE',  ( 93.41252705046289861, -7.949999999999998401, -4.867971026610728450E-16 ) ) ;
#140497=CARTESIAN_POINT ( 'NONE',  ( 124.7666937171295558, -7.949999999999999289, 2.130196079827424427 ) ) ;
#140535=CARTESIAN_POINT ( 'NONE',  ( 105.0004301918981184, -3.055000000000002380, 5.291415217122920289 ) ) ;
#140547=CARTESIAN_POINT ( 'NONE',  ( 93.09959685856479439, -6.109999999999997655, -1.637169565754160283 ) ) ;
#140596=CARTESIAN_POINT ( 'NONE',  ( 30.24543019189811233, -5.291415217122918513, -3.055000000000000160 ) ) ;
#140615=( BOUNDED_CURVE ( )  B_SPLINE_CURVE ( 2, ( #119540, #129725, #22370, #20237, #9337, #120990, #631, #65948, #76075, #30432, #74666, #118855, #120242, #65224, #66635, #110805, #107945, #109408, #76818, #110106, #20960, #8617, #10090, #52862, #98531, #142757, #87661, #32582, #99217, #143456, #44173, #47764, #100690, #4145, #123881, #35460, #91933, #2033, #46340, #124573, #23078, #89792, #90526, #102120, #1337, #80383, #57927, #134770, #15076, #69503, #79698, #2780, #78229, #89107, #136157, #12225, #133327, #78958, #24539, #14382, #67356, #59349, #47080, #102835, #68794, #112975, #91260, #103506, #34010, #101387, #36839, #122412, #13644, #70244, #45620, #58665, #111548, #56515, #68101, #25248, #81086, #135471, #36151, #113689, #134033, #114403, #125289, #34718, #3476, #123164, #25979, #23837, #112284, #12933, #57210, #29520, #62913, #84641, #117935, #94069, #81819, #16497, #82501, #18631, #73758, #126015, #139760, #28117, #116550, #93370, #38284, #107089, #139025, #73078, #40441, #106348, #128160, #126691, #15750, #92633, #117230, #27372, #7023, #60047, #72381, #17908, #60789, #51307, #48438, #128844, #49891, #138308, #95495, #49176, #26685, #17234, #136871, #61496, #37578, #70928, #71631, #104950, #115079, #105644, #104212, #6300, #115789, #4879, #137602, #5618, #127415, #38990, #83956, #83214, #94773, #50581, #39729, #28836, #62184, #75904, #142597, #119376, #10616, #7765, #96895, #54189, #141898, #9917, #76642, #118685, #20067, #41850, #121531, #132467, #85328, #99051, #131008, #120076, #52705, #141141, #22208, #96197, #19376, #86791, #54883, #43996, #109947, #31686, #98376, #43287, #86069, #65789, #63630, #20792, #120818, #64316, #143293, #66471, #88217, #9163, #97643, #33156, #107790, #52014, #130302, #42592, #21525, #8452, #75215, #30992, #108483, #77368, #65045, #53430, #109236, #87496, #41127, #140436, #129552, #131715, #32409, #30246, #74498, #46905, #56342, #1164, #112801, #67928, #122977, #91084, #133852, #34542, #123713, #458, #33844, #14198, #135305, #68618, #22908, #134588, #100520, #25065, #13461, #78768, #1851, #55595, #110636, #35986, #78060, #11313, #45446, #12762, #101932, #133162, #69321, #67172, #89626, #23659, #88943, #2595, #112115, #80215, #46158, #57743, #124399, #57037, #99783, #111364, #101210, #90337, #35285, #113506, #79526, #44751, #24371, #122237, #12054, #64074, #121993, #44497, #97377, #111110, #85809, #11801, #55350, #19833, #96650, #86551, #43049, #21978, #30749, #33610, #108241, #130783, #20536, #130047, #66227, #42341, #53938, #99525, #21281, #41592, #76387, #77810, #53178, #110400, #74977, #22662, #75669, #132204, #194, #121296, #10381, #9668, #64794, #141642, #31447, #32902, #109711, #140895, #119841, #87962, #108973, #98133, #131476, #66932, #119149, #132932, #8908, #142359, #87252, #11077, #32155, #120550, #65538, #54634, #98821, #77122, #143053, #88696, #43744, #28112, #4138, #70922, #138303, #106343, #95491, #17901, #38982, #6294, #50575, #93366, #117225, #26678, #83208, #28830, #27366, #62178, #73749, #139753, #60785, #115074, #7014, #15744, #117928, #104205, #49882, #128154, #60040, #126684, #4874, #71625, #51303, #72376, #49170, #116544, #38276, #92628, #40433, #84634, #127409, #128838, #59345, #29514, #103501, #82497, #137593, #48431, #136866, #94765, #37573, #115781, #17228, #81812, #126006, #16491, #104946, #5612, #61490, #94064, #139020, #105635, #39726, #83951, #73073, #98371, #77363, #88211, #64310, #52006, #43281, #8445, #18625, #54874, #52698, #63623, #9911, #132462, #65038, #20061, #130298, #109232, #87491, #10610, #76636, #142590, #96888, #129543, #62905, #131708, #33150, #107084, #21520, #141135, #7758, #41841, #109941, #43990, #99046, #32403, #54183, #120813, #19370, #96189, #42586, #140429, #86784, #41121, #143288, #86063, #65782, #30984, #85321, #75209, #30239, #119369, #108475, #74492, #118678, #97636, #107782, #9156, #53424, #141892, #131004, #31682, #75898, #120069, #20786, #67921, #124393, #34535, #78760, #13458, #55589, #88939, #36658, #69317, #2591, #122232, #123708, #23655, #47594, #101927, #122972, #134581, #110629, #121524, #80208, #44745, #22201, #111359, #112110, #46900, #99777, #58488, #133157, #12049, #45440, #11308, #91079, #91754, #66465, #133846, #25061, #453, #101204, #102661, #78053, #135302, #33836, #135982, #100514, #57737, #113500, #35981, #35281, #12756, #89618, #22902, #56335, #67166, #14192, #1158, #46151, #112795, #57031, #1844, #90332, #3305, #79520, #24364, #68610, #125102, #104779, #70064, #117066, #70757, #83777, #93191, #106175, #92451, #138132, #59861, #114227, #127991, #17741, #16313, #38116, #116375, #137424, #127233, #4692, #27207, #6849, #115608, #60607, #71452, #28672, #82335, #126517, #14905, #48258, #139590, #72920, #105473, #81635, #83038, #15582, #49721, #5439, #27935, #17065, #80903, #62016, #25785, #51132, #93896, #95327, #59179, #72205, #103330, #3977, #136687, #114904, #48991, #37391, #50415, #26513, #38818, #125838, #61331, #6136, #104035, #94601, #138856, #39551, #74313, #118501, #8285, #119904, #43112, #64863, #97455, #96717, #107624, #85158, #19202, #20609, #53239, #54702, #63459, #109045, #131534, #52534, #87319, #40274, #129373, #86621, #30815, #42412, #73590, #9734, #30061, #98882, #76458, #140962, #41663, #31510, #10445, #130848, #85878, #130117, #8979, #128677, #51845, #119213, #32224, #120627, #142425, #19894, #54004, #109775, #84483, #21345, #75043, #29346, #64142, #65606, #117759, #18446, #98198, #75732, #96034, #62729, #140271, #40956, #106909, #7589, #108308, #141707, #35823, #101753, #122795, #90158, #134404, #33673, #57567, #110462, #23478, #112633, #111182, #2412, #14009, #80049, #992, #89447, #46727, #269, #77185, #67742, #133681, #68455, #55412, #66998, #99590, #11868, #90906, #12594, #11135, #56872, #122061, #32968, #135136, #124223, #78586, #100340, #35103, #56156, #45977, #45276, #44566, #24899 ),
 .UNSPECIFIED., .F., .T. ) 
 B_SPLINE_CURVE_WITH_KNOTS ( ( 3, 2, 2, 2, 2, 2, 2, 2, 2, 2, 2, 2, 2, 2, 2, 2, 2, 2, 2, 2, 2, 2, 2, 2, 2, 2, 2, 2, 2, 2, 2, 2, 2, 2, 2, 2, 2, 2, 2, 2, 2, 2, 2, 2, 2, 2, 2, 2, 2, 2, 2, 2, 2, 2, 2, 2, 2, 2, 2, 2, 2, 2, 2, 2, 2, 2, 2, 2, 2, 2, 2, 2, 2, 2, 2, 2, 2, 2, 2, 2, 2, 2, 2, 2, 2, 2, 2, 2, 2, 2, 2, 2, 2, 2, 2, 2, 2, 2, 2, 2, 2, 2, 2, 2, 2, 2, 2, 2, 2, 2, 2, 2, 2, 2, 2, 2, 2, 2, 2, 2, 2, 2, 2, 2, 2, 2, 2, 2, 2, 2, 2, 2, 2, 2, 2, 2, 2, 2, 2, 2, 2, 2, 2, 2, 2, 2, 2, 2, 2, 2, 2, 2, 2, 2, 2, 2, 2, 2, 2, 2, 2, 2, 2, 2, 2, 2, 2, 2, 2, 2, 2, 2, 2, 2, 2, 2, 2, 2, 2, 2, 2, 2, 2, 2, 2, 2, 2, 2, 2, 2, 2, 2, 2, 2, 2, 2, 2, 2, 2, 2, 2, 2, 2, 2, 2, 2, 2, 2, 2, 2, 2, 2, 2, 2, 2, 2, 2, 2, 2, 2, 2, 2, 2, 2, 2, 2, 2, 2, 2, 2, 2, 2, 2, 2, 2, 2, 2, 2, 2, 2, 2, 2, 2, 2, 2, 2, 2, 2, 2, 2, 2, 2, 2, 2, 2, 2, 2, 2, 2, 2, 2, 2, 2, 2, 2, 2, 2, 2, 2, 2, 2, 2, 2, 2, 2, 2, 2, 2, 2, 2, 2, 2, 2, 2, 2, 2, 2, 2, 2, 2, 2, 2, 2, 2, 2, 2, 2, 2, 2, 2, 2, 2, 2, 2, 2, 2, 2, 2, 2, 2, 2, 2, 2, 2, 2, 2, 2, 2, 2, 2, 2, 2, 2, 2, 2, 2, 2, 2, 2, 2, 2, 2, 2, 2, 2, 2, 2, 2, 2, 2, 2, 2, 2, 2, 2, 2, 2, 2, 2, 2, 2, 3 ),
 ( 0.000000000000000000, 0.002777777777777777884, 0.005555555555555555768, 0.008333333333333333218, 0.01111111111111111154, 0.01388888888888888812, 0.01666666666666666644, 0.01944444444444444475, 0.02222222222222222307, 0.02500000000000000139, 0.02777777777777777624, 0.03055555555555555455, 0.03333333333333333287, 0.03611111111111110772, 0.03888888888888888951, 0.04166666666666666435, 0.04444444444444444614, 0.04722222222222222099, 0.05000000000000000278, 0.05277777777777777762, 0.05555555555555555247, 0.05833333333333333426, 0.06111111111111110911, 0.06388888888888888395, 0.06666666666666666574, 0.06944444444444444753, 0.07222222222222221544, 0.07499999999999999722, 0.07777777777777777901, 0.08055555555555556080, 0.08333333333333332871, 0.08611111111111111049, 0.08888888888888889228, 0.09166666666666666019, 0.09444444444444444198, 0.09722222222222222376, 0.1000000000000000056, 0.1027777777777777735, 0.1055555555555555552, 0.1083333333333333370, 0.1111111111111111049, 0.1138888888888888867, 0.1166666666666666685, 0.1194444444444444503, 0.1222222222222222182, 0.1250000000000000000, 0.1277777777777777679, 0.1305555555555555636, 0.1333333333333333315, 0.1361111111111110994, 0.1388888888888888951, 0.1416666666666666630, 0.1444444444444444309, 0.1472222222222222265, 0.1499999999999999944, 0.1527777777777777901, 0.1555555555555555580, 0.1583333333333333259, 0.1611111111111111216, 0.1638888888888888895, 0.1666666666666666574, 0.1694444444444444531, 0.1722222222222222210, 0.1750000000000000167, 0.1777777777777777846, 0.1805555555555555525, 0.1833333333333333204, 0.1861111111111111160, 0.1888888888888888840, 0.1916666666666666796, 0.1944444444444444475, 0.1972222222222222154, 0.2000000000000000111, 0.2027777777777777790, 0.2055555555555555469, 0.2083333333333333426, 0.2111111111111111105, 0.2138888888888888784, 0.2166666666666666741, 0.2194444444444444420, 0.2222222222222222099, 0.2249999999999999778, 0.2277777777777777735, 0.2305555555555555691, 0.2333333333333333370, 0.2361111111111111049, 0.2388888888888889006, 0.2416666666666666685, 0.2444444444444444364, 0.2472222222222222321, 0.2500000000000000000, 0.2527777777777777679, 0.2555555555555555358, 0.2583333333333333592, 0.2611111111111111271, 0.2638888888888888951, 0.2666666666666666630, 0.2694444444444444309, 0.2722222222222221988, 0.2750000000000000222, 0.2777777777777777901, 0.2805555555555555580, 0.2833333333333333259, 0.2861111111111110938, 0.2888888888888888618, 0.2916666666666666852, 0.2944444444444444531, 0.2972222222222222210, 0.2999999999999999889, 0.3027777777777777568, 0.3055555555555555802, 0.3083333333333333481, 0.3111111111111111160, 0.3138888888888888840, 0.3166666666666666519, 0.3194444444444444198, 0.3222222222222222432, 0.3250000000000000111, 0.3277777777777777790, 0.3305555555555555469, 0.3333333333333333148, 0.3361111111111111382, 0.3388888888888889062, 0.3416666666666666741, 0.3444444444444444420, 0.3472222222222222099, 0.3500000000000000333, 0.3527777777777778012, 0.3555555555555555691, 0.3583333333333333370, 0.3611111111111111049, 0.3638888888888888729, 0.3666666666666666408, 0.3694444444444444642, 0.3722222222222222321, 0.3750000000000000000, 0.3777777777777777679, 0.3805555555555555358, 0.3833333333333333592, 0.3861111111111111271, 0.3888888888888888951, 0.3916666666666666630, 0.3944444444444444309, 0.3972222222222221988, 0.4000000000000000222, 0.4027777777777777901, 0.4055555555555555580, 0.4083333333333333259, 0.4111111111111110938, 0.4138888888888888618, 0.4166666666666666852, 0.4194444444444444531, 0.4222222222222222210, 0.4249999999999999889, 0.4277777777777777568, 0.4305555555555555802, 0.4333333333333333481, 0.4361111111111111160, 0.4388888888888888840, 0.4416666666666666519, 0.4444444444444444198, 0.4472222222222222432, 0.4499999999999999556, 0.4527777777777777790, 0.4555555555555555469, 0.4583333333333333148, 0.4611111111111111382, 0.4638888888888889062, 0.4666666666666666741, 0.4694444444444444420, 0.4722222222222222099, 0.4749999999999999778, 0.4777777777777778012, 0.4805555555555555691, 0.4833333333333333370, 0.4861111111111111049, 0.4888888888888888729, 0.4916666666666666408, 0.4944444444444444642, 0.4972222222222222321, 0.5000000000000000000, 0.5027777777777777679, 0.5055555555555555358, 0.5083333333333333037, 0.5111111111111110716, 0.5138888888888888395, 0.5166666666666667185, 0.5194444444444444864, 0.5222222222222222543, 0.5250000000000000222, 0.5277777777777777901, 0.5305555555555555580, 0.5333333333333333259, 0.5361111111111110938, 0.5388888888888888618, 0.5416666666666666297, 0.5444444444444443976, 0.5472222222222222765, 0.5500000000000000444, 0.5527777777777778123, 0.5555555555555555802, 0.5583333333333333481, 0.5611111111111111160, 0.5638888888888888840, 0.5666666666666666519, 0.5694444444444444198, 0.5722222222222221877, 0.5749999999999999556, 0.5777777777777777235, 0.5805555555555556024, 0.5833333333333333703, 0.5861111111111112493, 0.5888888888888889062, 0.5916666666666666741, 0.5944444444444444420, 0.5972222222222222099, 0.5999999999999999778, 0.6027777777777777457, 0.6055555555555555136, 0.6083333333333332815, 0.6111111111111111605, 0.6138888888888889284, 0.6166666666666666963, 0.6194444444444444642, 0.6222222222222222321, 0.6250000000000000000, 0.6277777777777777679, 0.6305555555555555358, 0.6333333333333333037, 0.6361111111111110716, 0.6388888888888888395, 0.6416666666666667185, 0.6444444444444444864, 0.6472222222222222543, 0.6500000000000000222, 0.6527777777777777901, 0.6555555555555555580, 0.6583333333333333259, 0.6611111111111110938, 0.6638888888888888618, 0.6666666666666666297, 0.6694444444444443976, 0.6722222222222222765, 0.6750000000000000444, 0.6777777777777778123, 0.6805555555555555802, 0.6833333333333333481, 0.6861111111111111160, 0.6888888888888888840, 0.6916666666666666519, 0.6944444444444444198, 0.6972222222222221877, 0.7000000000000000666, 0.7027777777777777235, 0.7055555555555556024, 0.7083333333333333703, 0.7111111111111111382, 0.7138888888888889062, 0.7166666666666666741, 0.7194444444444444420, 0.7222222222222222099, 0.7249999999999999778, 0.7277777777777777457, 0.7305555555555555136, 0.7333333333333332815, 0.7361111111111111605, 0.7388888888888889284, 0.7416666666666666963, 0.7444444444444444642, 0.7472222222222222321, 0.7500000000000000000, 0.7527777777777777679, 0.7555555555555555358, 0.7583333333333333037, 0.7611111111111110716, 0.7638888888888888395, 0.7666666666666667185, 0.7694444444444444864, 0.7722222222222222543, 0.7750000000000000222, 0.7777777777777777901, 0.7805555555555555580, 0.7833333333333333259, 0.7861111111111110938, 0.7888888888888888618, 0.7916666666666666297, 0.7944444444444443976, 0.7972222222222222765, 0.8000000000000000444, 0.8027777777777778123, 0.8055555555555555802, 0.8083333333333333481, 0.8111111111111111160, 0.8138888888888888840, 0.8166666666666666519, 0.8194444444444444198, 0.8222222222222221877, 0.8249999999999999556, 0.8277777777777777235, 0.8305555555555556024, 0.8333333333333333703, 0.8361111111111111382, 0.8388888888888889062, 0.8416666666666666741, 0.8444444444444444420, 0.8472222222222222099, 0.8499999999999999778, 0.8527777777777777457, 0.8555555555555555136, 0.8583333333333332815, 0.8611111111111111605, 0.8638888888888889284, 0.8666666666666666963, 0.8694444444444444642, 0.8722222222222222321, 0.8750000000000000000, 0.8777777777777777679, 0.8805555555555555358, 0.8833333333333333037, 0.8861111111111110716, 0.8888888888888888395, 0.8916666666666667185, 0.8944444444444444864, 0.8972222222222222543, 0.8999999999999999112, 0.9027777777777777901, 0.9055555555555555580, 0.9083333333333333259, 0.9111111111111110938, 0.9138888888888888618, 0.9166666666666666297, 0.9194444444444443976, 0.9222222222222222765, 0.9250000000000000444, 0.9277777777777778123, 0.9305555555555555802, 0.9333333333333333481, 0.9361111111111111160, 0.9388888888888888840, 0.9416666666666666519, 0.9444444444444444198, 0.9472222222222221877, 0.9499999999999999556, 0.9527777777777777235, 0.9555555555555556024, 0.9583333333333333703, 0.9611111111111111382, 0.9638888888888889062, 0.9666666666666666741, 0.9694444444444444420, 0.9722222222222222099, 0.9749999999999999778 ),
 .UNSPECIFIED. ) 
 CURVE ( )  GEOMETRIC_REPRESENTATION_ITEM ( )  RATIONAL_B_SPLINE_CURVE ( ( 1.000000000000000000, 0.9659258262890683122, 1.000000000000000000, 0.9659258262890683122, 1.000000000000000000, 0.9659258262890683122, 1.000000000000000000, 0.9659258262890683122, 1.000000000000000000, 0.9659258262890683122, 1.000000000000000000, 0.9659258262890683122, 1.000000000000000000, 0.9659258262890683122, 1.000000000000000000, 0.9659258262890683122, 1.000000000000000000, 0.9659258262890683122, 1.000000000000000000, 0.9659258262890683122, 1.000000000000000000, 0.9659258262890683122, 1.000000000000000000, 0.9659258262890683122, 1.000000000000000000, 0.9659258262890683122, 1.000000000000000000, 0.9659258262890683122, 1.000000000000000000, 0.9659258262890683122, 1.000000000000000000, 0.9659258262890683122, 1.000000000000000000, 0.9659258262890683122, 1.000000000000000000, 0.9659258262890683122, 1.000000000000000000, 0.9659258262890683122, 1.000000000000000000, 0.9659258262890683122, 1.000000000000000000, 0.9659258262890683122, 1.000000000000000000, 0.9659258262890683122, 1.000000000000000000, 0.9659258262890683122, 1.000000000000000000, 0.9659258262890683122, 1.000000000000000000, 0.9659258262890683122, 1.000000000000000000, 0.9659258262890683122, 1.000000000000000000, 0.9659258262890683122, 1.000000000000000000, 0.9659258262890683122, 1.000000000000000000, 0.9659258262890683122, 1.000000000000000000, 0.9659258262890683122, 1.000000000000000000, 0.9659258262890683122, 1.000000000000000000, 0.9659258262890683122, 1.000000000000000000, 0.9659258262890683122, 1.000000000000000000, 0.9659258262890683122, 1.000000000000000000, 0.9659258262890683122, 1.000000000000000000, 0.9659258262890683122, 1.000000000000000000, 0.9659258262890683122, 1.000000000000000000, 0.9659258262890683122, 1.000000000000000000, 0.9659258262890683122, 1.000000000000000000, 0.9659258262890683122, 1.000000000000000000, 0.9659258262890683122, 1.000000000000000000, 0.9659258262890683122, 1.000000000000000000, 0.9659258262890683122, 1.000000000000000000, 0.9659258262890683122, 1.000000000000000000, 0.9659258262890683122, 1.000000000000000000, 0.9659258262890683122, 1.000000000000000000, 0.9659258262890683122, 1.000000000000000000, 0.9659258262890683122, 1.000000000000000000, 0.9659258262890683122, 1.000000000000000000, 0.9659258262890683122, 1.000000000000000000, 0.9659258262890683122, 1.000000000000000000, 0.9659258262890683122, 1.000000000000000000, 0.9659258262890683122, 1.000000000000000000, 0.9659258262890683122, 1.000000000000000000, 0.9659258262890683122, 1.000000000000000000, 0.9659258262890683122, 1.000000000000000000, 0.9659258262890683122, 1.000000000000000000, 0.9659258262890683122, 1.000000000000000000, 0.9659258262890683122, 1.000000000000000000, 0.9659258262890683122, 1.000000000000000000, 0.9659258262890683122, 1.000000000000000000, 0.9659258262890683122, 1.000000000000000000, 0.9659258262890683122, 1.000000000000000000, 0.9659258262890683122, 1.000000000000000000, 0.9659258262890683122, 1.000000000000000000, 0.9659258262890683122, 1.000000000000000000, 0.9659258262890683122, 1.000000000000000000, 0.9659258262890683122, 1.000000000000000000, 0.9659258262890683122, 1.000000000000000000, 0.9659258262890683122, 1.000000000000000000, 0.9659258262890683122, 1.000000000000000000, 0.9659258262890683122, 1.000000000000000000, 0.9659258262890683122, 1.000000000000000000, 0.9659258262890683122, 1.000000000000000000, 0.9659258262890683122, 1.000000000000000000, 0.9659258262890683122, 1.000000000000000000, 0.9659258262890683122, 1.000000000000000000, 0.9659258262890683122, 1.000000000000000000, 0.9659258262890683122, 1.000000000000000000, 0.9659258262890683122, 1.000000000000000000, 0.9659258262890683122, 1.000000000000000000, 0.9659258262890683122, 1.000000000000000000, 0.9659258262890683122, 1.000000000000000000, 0.9659258262890683122, 1.000000000000000000, 0.9659258262890683122, 1.000000000000000000, 0.9659258262890683122, 1.000000000000000000, 0.9659258262890683122, 1.000000000000000000, 0.9659258262890683122, 1.000000000000000000, 0.9659258262890683122, 1.000000000000000000, 0.9659258262890683122, 1.000000000000000000, 0.9659258262890683122, 1.000000000000000000, 0.9659258262890683122, 1.000000000000000000, 0.9659258262890683122, 1.000000000000000000, 0.9659258262890683122, 1.000000000000000000, 0.9659258262890683122, 1.000000000000000000, 0.9659258262890683122, 1.000000000000000000, 0.9659258262890683122, 1.000000000000000000, 0.9659258262890683122, 1.000000000000000000, 0.9659258262890683122, 1.000000000000000000, 0.9659258262890683122, 1.000000000000000000, 0.9659258262890683122, 1.000000000000000000, 0.9659258262890683122, 1.000000000000000000, 0.9659258262890683122, 1.000000000000000000, 0.9659258262890683122, 1.000000000000000000, 0.9659258262890683122, 1.000000000000000000, 0.9659258262890683122, 1.000000000000000000, 0.9659258262890683122, 1.000000000000000000, 0.9659258262890683122, 1.000000000000000000, 0.9659258262890683122, 1.000000000000000000, 0.9659258262890683122, 1.000000000000000000, 0.9659258262890683122, 1.000000000000000000, 0.9659258262890683122, 1.000000000000000000, 0.9659258262890683122, 1.000000000000000000, 0.9659258262890683122, 1.000000000000000000, 0.9659258262890683122, 1.000000000000000000, 0.9659258262890683122, 1.000000000000000000, 0.9659258262890683122, 1.000000000000000000, 0.9659258262890683122, 1.000000000000000000, 0.9659258262890683122, 1.000000000000000000, 0.9659258262890683122, 1.000000000000000000, 0.9659258262890683122, 1.000000000000000000, 0.9659258262890683122, 1.000000000000000000, 0.9659258262890683122, 1.000000000000000000, 0.9659258262890683122, 1.000000000000000000, 0.9659258262890683122, 1.000000000000000000, 0.9659258262890683122, 1.000000000000000000, 0.9659258262890683122, 1.000000000000000000, 0.9659258262890683122, 1.000000000000000000, 0.9659258262890683122, 1.000000000000000000, 0.9659258262890683122, 1.000000000000000000, 0.9659258262890683122, 1.000000000000000000, 0.9659258262890683122, 1.000000000000000000, 0.9659258262890683122, 1.000000000000000000, 0.9659258262890683122, 1.000000000000000000, 0.9659258262890683122, 1.000000000000000000, 0.9659258262890683122, 1.000000000000000000, 0.9659258262890683122, 1.000000000000000000, 0.9659258262890683122, 1.000000000000000000, 0.9659258262890683122, 1.000000000000000000, 0.9659258262890683122, 1.000000000000000000, 0.9659258262890683122, 1.000000000000000000, 0.9659258262890683122, 1.000000000000000000, 0.9659258262890683122, 1.000000000000000000, 0.9659258262890683122, 1.000000000000000000, 0.9659258262890683122, 1.000000000000000000, 0.9659258262890683122, 1.000000000000000000, 0.9659258262890683122, 1.000000000000000000, 0.9659258262890683122, 1.000000000000000000, 0.9659258262890683122, 1.000000000000000000, 0.9659258262890683122, 1.000000000000000000, 0.9659258262890683122, 1.000000000000000000, 0.9659258262890683122, 1.000000000000000000, 0.9659258262890683122, 1.000000000000000000, 0.9659258262890683122, 1.000000000000000000, 0.9659258262890683122, 1.000000000000000000, 0.9659258262890683122, 1.000000000000000000, 0.9659258262890683122, 1.000000000000000000, 0.9659258262890683122, 1.000000000000000000, 0.9659258262890683122, 1.000000000000000000, 0.9659258262890683122, 1.000000000000000000, 0.9659258262890683122, 1.000000000000000000, 0.9659258262890683122, 1.000000000000000000, 0.9659258262890683122, 1.000000000000000000, 0.9659258262890683122, 1.000000000000000000, 0.9659258262890683122, 1.000000000000000000, 0.9659258262890683122, 1.000000000000000000, 0.9659258262890683122, 1.000000000000000000, 0.9659258262890683122, 1.000000000000000000, 0.9659258262890683122, 1.000000000000000000, 0.9659258262890683122, 1.000000000000000000, 0.9659258262890683122, 1.000000000000000000, 0.9659258262890683122, 1.000000000000000000, 0.9659258262890683122, 1.000000000000000000, 0.9659258262890683122, 1.000000000000000000, 0.9659258262890683122, 1.000000000000000000, 0.9659258262890683122, 1.000000000000000000, 0.9659258262890683122, 1.000000000000000000, 0.9659258262890683122, 1.000000000000000000, 0.9659258262890683122, 1.000000000000000000, 0.9659258262890683122, 1.000000000000000000, 0.9659258262890683122, 1.000000000000000000, 0.9659258262890683122, 1.000000000000000000, 0.9659258262890683122, 1.000000000000000000, 0.9659258262890683122, 1.000000000000000000, 0.9659258262890683122, 1.000000000000000000, 0.9659258262890683122, 1.000000000000000000, 0.9659258262890683122, 1.000000000000000000, 0.9659258262890683122, 1.000000000000000000, 0.9659258262890683122, 1.000000000000000000, 0.9659258262890683122, 1.000000000000000000, 0.9659258262890683122, 1.000000000000000000, 0.9659258262890683122, 1.000000000000000000, 0.9659258262890683122, 1.000000000000000000, 0.9659258262890683122, 1.000000000000000000, 0.9659258262890683122, 1.000000000000000000, 0.9659258262890683122, 1.000000000000000000, 0.9659258262890683122, 1.000000000000000000, 0.9659258262890683122, 1.000000000000000000, 0.9659258262890683122, 1.000000000000000000, 0.9659258262890683122, 1.000000000000000000, 0.9659258262890683122, 1.000000000000000000, 0.9659258262890683122, 1.000000000000000000, 0.9659258262890683122, 1.000000000000000000, 0.9659258262890683122, 1.000000000000000000, 0.9659258262890683122, 1.000000000000000000, 0.9659258262890683122, 1.000000000000000000, 0.9659258262890683122, 1.000000000000000000, 0.9659258262890683122, 1.000000000000000000, 0.9659258262890683122, 1.000000000000000000, 0.9659258262890683122, 1.000000000000000000, 0.9659258262890683122, 1.000000000000000000, 0.9659258262890683122, 1.000000000000000000, 0.9659258262890683122, 1.000000000000000000, 0.9659258262890683122, 1.000000000000000000, 0.9659258262890683122, 1.000000000000000000, 0.9659258262890683122, 1.000000000000000000, 0.9659258262890683122, 1.000000000000000000, 0.9659258262890683122, 1.000000000000000000, 0.9659258262890683122, 1.000000000000000000, 0.9659258262890683122, 1.000000000000000000, 0.9659258262890683122, 1.000000000000000000, 0.9659258262890683122, 1.000000000000000000, 0.9659258262890683122, 1.000000000000000000, 0.9659258262890683122, 1.000000000000000000, 0.9659258262890683122, 1.000000000000000000, 0.9659258262890683122, 1.000000000000000000, 0.9659258262890683122, 1.000000000000000000, 0.9659258262890683122, 1.000000000000000000, 0.9659258262890683122, 1.000000000000000000, 0.9659258262890683122, 1.000000000000000000, 0.9659258262890683122, 1.000000000000000000, 0.9659258262890683122, 1.000000000000000000, 0.9659258262890683122, 1.000000000000000000, 0.9659258262890683122, 1.000000000000000000, 0.9659258262890683122, 1.000000000000000000, 0.9659258262890683122, 1.000000000000000000, 0.9659258262890683122, 1.000000000000000000, 0.9659258262890683122, 1.000000000000000000, 0.9659258262890683122, 1.000000000000000000, 0.9659258262890683122, 1.000000000000000000, 0.9659258262890683122, 1.000000000000000000, 0.9659258262890683122, 1.000000000000000000, 0.9659258262890683122, 1.000000000000000000, 0.9659258262890683122, 1.000000000000000000, 0.9659258262890683122, 1.000000000000000000, 0.9659258262890683122, 1.000000000000000000, 0.9659258262890683122, 1.000000000000000000, 0.9659258262890683122, 1.000000000000000000, 0.9659258262890683122, 1.000000000000000000, 0.9659258262890683122, 1.000000000000000000, 0.9659258262890683122, 1.000000000000000000, 0.9659258262890683122, 1.000000000000000000, 0.9659258262890683122, 1.000000000000000000, 0.9659258262890683122, 1.000000000000000000, 0.9659258262890683122, 1.000000000000000000, 0.9659258262890683122, 1.000000000000000000, 0.9659258262890683122, 1.000000000000000000, 0.9659258262890683122, 1.000000000000000000, 0.9659258262890683122, 1.000000000000000000, 0.9659258262890683122, 1.000000000000000000, 0.9659258262890683122, 1.000000000000000000, 0.9659258262890683122, 1.000000000000000000, 0.9659258262890683122, 1.000000000000000000, 0.9659258262890683122, 1.000000000000000000, 0.9659258262890683122, 1.000000000000000000, 0.9659258262890683122, 1.000000000000000000, 0.9659258262890683122, 1.000000000000000000, 0.9659258262890683122, 1.000000000000000000, 0.9659258262890683122, 1.000000000000000000, 0.9659258262890683122, 1.000000000000000000, 0.9659258262890683122, 1.000000000000000000, 0.9659258262890683122, 1.000000000000000000, 0.9659258262890683122, 1.000000000000000000, 0.9659258262890683122, 1.000000000000000000, 0.9659258262890683122, 1.000000000000000000, 0.9659258262890683122, 1.000000000000000000, 0.9659258262890683122, 1.000000000000000000, 0.9659258262890683122, 1.000000000000000000, 0.9659258262890683122, 1.000000000000000000, 0.9659258262890683122, 1.000000000000000000, 0.9659258262890683122, 1.000000000000000000, 0.9659258262890683122, 1.000000000000000000, 0.9659258262890683122, 1.000000000000000000, 0.9659258262890683122, 1.000000000000000000, 0.9659258262890683122, 1.000000000000000000, 0.9659258262890683122, 1.000000000000000000, 0.9659258262890683122, 1.000000000000000000, 0.9659258262890683122, 1.000000000000000000, 0.9659258262890683122, 1.000000000000000000, 0.9659258262890683122, 1.000000000000000000, 0.9659258262890683122, 1.000000000000000000, 0.9659258262890683122, 1.000000000000000000, 0.9659258262890683122, 1.000000000000000000, 0.9659258262890683122, 1.000000000000000000, 0.9659258262890683122, 1.000000000000000000, 0.9659258262890683122, 1.000000000000000000, 0.9659258262890683122, 1.000000000000000000, 0.9659258262890683122, 1.000000000000000000, 0.9659258262890683122, 1.000000000000000000, 0.9659258262890683122, 1.000000000000000000, 0.9659258262890683122, 1.000000000000000000, 0.9659258262890683122, 1.000000000000000000, 0.9659258262890683122, 1.000000000000000000, 0.9659258262890683122, 1.000000000000000000, 0.9659258262890683122, 1.000000000000000000, 0.9659258262890683122, 1.000000000000000000, 0.9659258262890683122, 1.000000000000000000, 0.9659258262890683122, 1.000000000000000000, 0.9659258262890683122, 1.000000000000000000, 0.9659258262890683122, 1.000000000000000000, 0.9659258262890683122, 1.000000000000000000, 0.9659258262890683122, 1.000000000000000000, 0.9659258262890683122, 1.000000000000000000, 0.9659258262890683122, 1.000000000000000000, 0.9659258262890683122, 1.000000000000000000, 0.9659258262890683122, 1.000000000000000000, 0.9659258262890683122, 1.000000000000000000, 0.9659258262890683122, 1.000000000000000000, 0.9659258262890683122, 1.000000000000000000, 0.9659258262890683122, 1.000000000000000000, 0.9659258262890683122, 1.000000000000000000, 0.9659258262890683122, 1.000000000000000000, 0.9659258262890683122, 1.000000000000000000, 0.9659258262890683122, 1.000000000000000000, 0.9659258262890683122, 1.000000000000000000, 0.9659258262890683122, 1.000000000000000000, 0.9659258262890683122, 1.000000000000000000, 0.9659258262890683122, 1.000000000000000000, 0.9659258262890683122, 1.000000000000000000, 0.9659258262890683122, 1.000000000000000000, 0.9659258262890683122, 1.000000000000000000, 0.9659258262890683122, 1.000000000000000000, 0.9659258262890683122, 1.000000000000000000, 0.9659258262890683122, 1.000000000000000000, 0.9659258262890683122, 1.000000000000000000, 0.9659258262890683122, 1.000000000000000000, 0.9659258262890683122, 1.000000000000000000, 0.9659258262890683122, 1.000000000000000000, 0.9659258262890683122, 1.000000000000000000, 0.9659258262890683122, 1.000000000000000000, 0.9659258262890683122, 1.000000000000000000, 0.9659258262890683122, 1.000000000000000000, 0.9659258262890683122, 1.000000000000000000, 0.9659258262890683122, 1.000000000000000000, 0.9659258262890683122, 1.000000000000000000, 0.9659258262890683122, 1.000000000000000000, 0.9659258262890683122, 1.000000000000000000, 0.9659258262890683122, 1.000000000000000000, 0.9659258262890683122, 1.000000000000000000, 0.9659258262890683122, 1.000000000000000000, 0.9659258262890683122, 1.000000000000000000 ) ) 
 REPRESENTATION_ITEM ( '' )  );
#140630=CARTESIAN_POINT ( 'NONE',  ( 89.45376352523146579, -6.109999999999999432, -3.741295971395163529E-16 ) ) ;
#140633=CARTESIAN_POINT ( 'NONE',  ( 10.32500000000000107, 8.432637487761466488, -4.375000000000001776 ) ) ;
#140657=DIRECTION ( 'NONE',  ( -1.000000000000000000, -0.000000000000000000, -0.000000000000000000 ) ) ;
#140680=CARTESIAN_POINT ( 'NONE',  ( 111.8333333333333428, -6.884901960086287964, 3.974999999999998312 ) ) ;
#140682=EDGE_LOOP ( 'NONE', ( #54896, #52506, #141037, #63359 ) ) ;
#140693=CARTESIAN_POINT ( 'NONE',  ( 107.3337635252314470, 6.110000000000001208, 1.122388791418549305E-15 ) ) ;
#140702=CARTESIAN_POINT ( 'NONE',  ( 27.49586038379622721, -3.974999999999998312, -6.884901960086286188 ) ) ;
#140708=CARTESIAN_POINT ( 'NONE',  ( 24.91666666666665719, -6.884901960086287076, -3.975000000000000977 ) ) ;
#140718=CARTESIAN_POINT ( 'NONE',  ( 120.6620968585647802, -5.291415217122919401, 3.054999999999997939 ) ) ;
#140722=CARTESIAN_POINT ( 'NONE',  ( 71.53752705046289861, -9.735942053221456900E-16, 7.949999999999998401 ) ) ;
#140726=CARTESIAN_POINT ( 'NONE',  ( 42.72959685856476142, -6.110000000000000320, -1.637169565754161393 ) ) ;
#140736=CARTESIAN_POINT ( 'NONE',  ( 42.34959685856478018, 6.109999999999996767, 1.637169565754163836 ) ) ;
#140762=CARTESIAN_POINT ( 'NONE',  ( 60.87043019189810877, -3.055000000000001492, 5.291415217122917625 ) ) ;
#140782=CIRCLE ( 'NONE', #115297, 9.500000000000001776 ) ;
#140796=CARTESIAN_POINT ( 'NONE',  ( 115.7037635252314516, 6.109999999999999432, 1.122388791418549108E-15 ) ) ;
#140836=CARTESIAN_POINT ( 'NONE',  ( 38.41209685856478018, 5.291415217122922066, -3.054999999999995275 ) ) ;
#140862=CARTESIAN_POINT ( 'NONE',  ( 59.87086038379622721, 6.884901960086289741, -3.974999999999993427 ) ) ;
#140866=CARTESIAN_POINT ( 'NONE',  ( 55.39583333333331439, -2.130196079827427091, 7.949999999999999289 ) ) ;
#140874=EDGE_CURVE ( 'NONE', #53423, #139751, #33918, .T. ) ;
#140875=CARTESIAN_POINT ( 'NONE',  ( 45.35459685856476852, -1.637169565754161615, 6.110000000000000320 ) ) ;
#140885=CARTESIAN_POINT ( 'NONE',  ( 82.03752705046288440, -9.735942053221456900E-16, 7.949999999999998401 ) ) ;
#140895=CARTESIAN_POINT ( 'NONE',  ( 80.93793019189809002, -6.110000000000001208, 1.637169565754158951 ) ) ;
#140906=CARTESIAN_POINT ( 'NONE',  ( 66.12043019189812298, 3.055000000000001936, -5.291415217122916737 ) ) ;
#140941=CARTESIAN_POINT ( 'NONE',  ( 82.16209685856479439, -5.291415217122919401, 3.054999999999997939 ) ) ;
#140962=CARTESIAN_POINT ( 'NONE',  ( 36.16709685856476852, -3.055000000000000160, -5.291415217122921177 ) ) ;
#140996=CARTESIAN_POINT ( 'NONE',  ( 67.35416666666664298, -2.130196079827425759, -7.950000000000000178 ) ) ;
#141015=CARTESIAN_POINT ( 'NONE',  ( 61.30793019189810877, -6.109999999999999432, 1.637169565754158507 ) ) ;
#141037=ORIENTED_EDGE ( 'NONE', *, *, #60056, .T. ) ;
#141039=CARTESIAN_POINT ( 'NONE',  ( 127.0000000000000568, -4.172191364199829167, -4.786994800550450790 ) ) ;
#141045=CARTESIAN_POINT ( 'NONE',  ( 81.16252705046289861, 7.949999999999998401, 1.460391307983218338E-15 ) ) ;
#141058=CARTESIAN_POINT ( 'NONE',  ( 79.47959685856477563, 6.109999999999999432, 1.637169565754164280 ) ) ;
#141071=CARTESIAN_POINT ( 'NONE',  ( 77.70833333333332860, -3.974999999999999201, -6.884901960086287964 ) ) ;
#141076=CARTESIAN_POINT ( 'NONE',  ( 71.31293019189810423, -1.637169565754159617, -6.110000000000001208 ) ) ;
#141077=ORIENTED_EDGE ( 'NONE', *, *, #46899, .T. ) ;
#141086=CARTESIAN_POINT ( 'NONE',  ( 125.5000000000000568, -3.922572014496796822, -6.914906274931464480 ) ) ;
#141103=EDGE_CURVE ( 'NONE', #135001, #33848, #2520, .T. ) ;
#141112=CARTESIAN_POINT ( 'NONE',  ( 1.500000000000000000, 0.000000000000000000, 9.500000000000001776 ) ) ;
#141134=ORIENTED_EDGE ( 'NONE', *, *, #635, .F. ) ;
#141135=CARTESIAN_POINT ( 'NONE',  ( 64.31293019189810423, -1.637169565754159617, -6.110000000000001208 ) ) ;
#141141=CARTESIAN_POINT ( 'NONE',  ( 101.3545968585647614, -1.637169565754161615, 6.110000000000000320 ) ) ;
#141150=VERTEX_POINT ( 'NONE', #114325 ) ;
#141156=CARTESIAN_POINT ( 'NONE',  ( 119.2037635252314658, 6.109999999999998543, 1.122388791418548911E-15 ) ) ;
#141159=DIRECTION ( 'NONE',  ( -1.000000000000000000, -0.000000000000000000, -0.000000000000000000 ) ) ;
#141172=CARTESIAN_POINT ( 'NONE',  ( 39.20833333333332860, -3.974999999999999201, -6.884901960086287964 ) ) ;
#141185=CARTESIAN_POINT ( 'NONE',  ( 30.18793019189809357, 6.110000000000002984, -1.637169565754156730 ) ) ;
#141196=CARTESIAN_POINT ( 'NONE',  ( 41.97916666666665719, -7.950000000000000178, 2.130196079827424427 ) ) ;
#141208=CARTESIAN_POINT ( 'NONE',  ( 119.0791937171295700, 3.975000000000002753, -6.884901960086283523 ) ) ;
#141226=VECTOR ( 'NONE', #143193, 1000.000000000000000 ) ;
#141228=CARTESIAN_POINT ( 'NONE',  ( 20.65000000000000213, 0.000000000000000000, 6.350000000000008527 ) ) ;
#141235=CARTESIAN_POINT ( 'NONE',  ( 92.00000000000000000, 0.000000000000000000, -7.950000000000000178 ) ) ;
#141237=FACE_OUTER_BOUND ( 'NONE', #119345, .T. ) ;
#141247=ORIENTED_EDGE ( 'NONE', *, *, #107335, .T. ) ;
#141249=CARTESIAN_POINT ( 'NONE',  ( 102.3754301918981184, -5.291415217122920289, -3.055000000000001492 ) ) ;
#141259=CARTESIAN_POINT ( 'NONE',  ( 94.55793019189810877, 6.110000000000000320, -1.637169565754156064 ) ) ;
#141316=CARTESIAN_POINT ( 'NONE',  ( 31.26626352523144448, 4.472830434245838482, -4.472830434245837594 ) ) ;
#141352=CARTESIAN_POINT ( 'NONE',  ( 95.87043019189810877, -3.055000000000001936, 5.291415217122918513 ) ) ;
#141392=CARTESIAN_POINT ( 'NONE',  ( 31.62500000000000000, -7.950000000000000178, -4.867971026610729436E-16 ) ) ;
#141407=CARTESIAN_POINT ( 'NONE',  ( 115.0416666666666714, -3.975000000000002753, 6.884901960086286188 ) ) ;
#141425=CARTESIAN_POINT ( 'NONE',  ( 100.6254301918981042, 5.291415217122919401, 3.055000000000002824 ) ) ;
#141439=CARTESIAN_POINT ( 'NONE',  ( 28.41666666666666075, -6.884901960086287076, -3.975000000000000977 ) ) ;
#141451=CARTESIAN_POINT ( 'NONE',  ( 119.4954301918981230, 5.291415217122916737, 3.055000000000001936 ) ) ;
#141463=CARTESIAN_POINT ( 'NONE',  ( 46.52126352523142572, -4.472830434245839371, -4.472830434245840259 ) ) ;
#141471=CARTESIAN_POINT ( 'NONE',  ( 40.74543019189810877, -5.291415217122918513, -3.055000000000000160 ) ) ;
#141485=( BOUNDED_CURVE ( )  B_SPLINE_CURVE ( 2, ( #85123, #60002, #49849, #58624, #60750, #4834, #15711, #115747, #25937, #85832, #8244, #103466, #30019 ),
 .UNSPECIFIED., .F., .T. ) 
 B_SPLINE_CURVE_WITH_KNOTS ( ( 3, 2, 2, 2, 2, 2, 3 ),
 ( 0.5833333333333333703, 0.5861111111111111382, 0.5888888888888889062, 0.5916666666666666741, 0.5944444444444444420, 0.5972222222222222099, 0.5999999999999999778 ),
 .UNSPECIFIED. ) 
 CURVE ( )  GEOMETRIC_REPRESENTATION_ITEM ( )  RATIONAL_B_SPLINE_CURVE ( ( 1.000000000000000000, 0.9659258262890683122, 1.000000000000000000, 0.9659258262890683122, 1.000000000000000000, 0.9659258262890683122, 1.000000000000000000, 0.9659258262890683122, 1.000000000000000000, 0.9659258262890683122, 1.000000000000000000, 0.9659258262890683122, 1.000000000000000000 ) ) 
 REPRESENTATION_ITEM ( '' )  );
#141502=CARTESIAN_POINT ( 'NONE',  ( 56.05793019189811588, 6.110000000000000320, -1.637169565754156064 ) ) ;
#141540=CARTESIAN_POINT ( 'NONE',  ( 122.2662635252314374, 4.472830434245839371, -4.472830434245839371 ) ) ;
#141584=CARTESIAN_POINT ( 'NONE',  ( 126.5615712523421053, -6.570126589092502911, -2.091773665023263451 ) ) ;
#141585=CARTESIAN_POINT ( 'NONE',  ( 36.22459685856478728, -1.637169565754161171, 6.109999999999998543 ) ) ;
#141610=CARTESIAN_POINT ( 'NONE',  ( 57.82919371712954870, -3.975000000000001865, 6.884901960086284411 ) ) ;
#141615=CARTESIAN_POINT ( 'NONE',  ( 57.87499999999999289, 7.950000000000000178, 1.460391307983218535E-15 ) ) ;
#141624=CARTESIAN_POINT ( 'NONE',  ( 48.12543019189810423, 5.291415217122919401, 3.055000000000002824 ) ) ;
#141630=AXIS2_PLACEMENT_3D ( 'NONE', #129633, #41940, #75290 ) ;
#141642=CARTESIAN_POINT ( 'NONE',  ( 81.52126352523141861, -4.472830434245838482, -4.472830434245840259 ) ) ;
#141651=CARTESIAN_POINT ( 'NONE',  ( 69.32876352523145158, 0.000000000000000000, -6.109999999999998543 ) ) ;
#141658=DIRECTION ( 'NONE',  ( 0.000000000000000000, 0.000000000000000000, 1.000000000000000000 ) ) ;
#141680=CARTESIAN_POINT ( 'NONE',  ( 85.07876352523143737, -7.482591942790325086E-16, 6.109999999999998543 ) ) ;
#141707=CARTESIAN_POINT ( 'NONE',  ( 31.20876352523144348, -7.482591942790329030E-16, 6.110000000000001208 ) ) ;
#141736=ORIENTED_EDGE ( 'NONE', *, *, #99361, .F. ) ;
#141743=EDGE_CURVE ( 'NONE', #114577, #107625, #51054, .T. ) ;
#141767=CARTESIAN_POINT ( 'NONE',  ( 65.82876352523145158, 0.000000000000000000, -6.109999999999999432 ) ) ;
#141783=CARTESIAN_POINT ( 'NONE',  ( 106.8750000000000000, 7.950000000000000178, 1.460391307983218535E-15 ) ) ;
#141794=CARTESIAN_POINT ( 'NONE',  ( 83.93336038379621300, 2.130196079827431532, -7.949999999999997513 ) ) ;
#141795=LINE ( 'NONE', #51926, #48607 ) ;
#141808=CARTESIAN_POINT ( 'NONE',  ( 73.93793019189809002, -6.110000000000001208, 1.637169565754158951 ) ) ;
#141823=CARTESIAN_POINT ( 'NONE',  ( 77.56250000000000000, -5.819803920172573086, -5.819803920172573974 ) ) ;
#141827=CARTESIAN_POINT ( 'NONE',  ( 63.29209685856476852, -5.291415217122921177, 3.054999999999999272 ) ) ;
#141864=CARTESIAN_POINT ( 'NONE',  ( 112.7870968585647802, 3.054999999999997495, 5.291415217122919401 ) ) ;
#141866=ADVANCED_FACE ( 'NONE', ( #46652 ), #132195, .T. ) ;
#141878=CARTESIAN_POINT ( 'NONE',  ( 57.97502705046289151, -5.819803920172573086, 5.819803920172573086 ) ) ;
#141892=CARTESIAN_POINT ( 'NONE',  ( 59.93793019189810423, -6.110000000000001208, 1.637169565754158951 ) ) ;
#141898=CARTESIAN_POINT ( 'NONE',  ( 103.2504301918981184, 3.055000000000002824, -5.291415217122919401 ) ) ;
#141909=CARTESIAN_POINT ( 'NONE',  ( 78.10002705046289861, 5.819803920172570422, 5.819803920172575751 ) ) ;
#141917=CARTESIAN_POINT ( 'NONE',  ( 124.8912635252314516, -4.472830434245838482, -4.472830434245838482 ) ) ;
#141920=( BOUNDED_CURVE ( )  B_SPLINE_CURVE ( 2, ( #97800, #10762, #133311, #42738, #99198, #20942, #65206, #54337, #143438, #99951, #44154, #88377, #132616 ),
 .UNSPECIFIED., .F., .T. ) 
 B_SPLINE_CURVE_WITH_KNOTS ( ( 3, 2, 2, 2, 2, 2, 3 ),
 ( 0.06666666666666672125, 0.06944444444444450304, 0.07222222222222228483, 0.07500000000000006661, 0.07777777777777784840, 0.08055555555555564407, 0.08333333333333341197 ),
 .UNSPECIFIED. ) 
 CURVE ( )  GEOMETRIC_REPRESENTATION_ITEM ( )  RATIONAL_B_SPLINE_CURVE ( ( 0.9999999999999993339, 0.9659258262890689783, 1.000000000000000000, 0.9659258262890683122, 1.000000000000000000, 0.9659258262890683122, 1.000000000000000000, 0.9659258262890683122, 1.000000000000000000, 0.9659258262890683122, 1.000000000000000000, 0.9659258262890673130, 1.000000000000001110 ) ) 
 REPRESENTATION_ITEM ( '' )  );
#141936=CYLINDRICAL_SURFACE ( 'NONE', #92696, 7.950000000000000178 ) ;
#141945=CARTESIAN_POINT ( 'NONE',  ( 32.37543019189810423, -5.291415217122920289, -3.055000000000001492 ) ) ;
#141967=CARTESIAN_POINT ( 'NONE',  ( 108.5791937171295700, 3.975000000000002753, -6.884901960086283523 ) ) ;
#141977=VECTOR ( 'NONE', #96728, 1000.000000000000000 ) ;
#142003=CARTESIAN_POINT ( 'NONE',  ( 95.37543019189810423, -5.291415217122920289, -3.055000000000001492 ) ) ;
#142006=MANIFOLD_SOLID_BREP ( 'Cut-Extrude1', #138928 ) ;
#142012=CARTESIAN_POINT ( 'NONE',  ( 48.68749999999998579, -5.819803920172573974, 5.819803920172573086 ) ) ;
#142013=CARTESIAN_POINT ( 'NONE',  ( 98.93293019189812298, 1.637169565754156508, 6.110000000000000320 ) ) ;
#142018=CARTESIAN_POINT ( 'NONE',  ( 115.3333333333333286, -6.884901960086287964, 3.974999999999998312 ) ) ;
#142051=ORIENTED_EDGE ( 'NONE', *, *, #7958, .F. ) ;
#142079=VERTEX_POINT ( 'NONE', #56464 ) ;
#142099=CARTESIAN_POINT ( 'NONE',  ( 89.89126352523143737, -4.472830434245839371, -4.472830434245839371 ) ) ;
#142144=CARTESIAN_POINT ( 'NONE',  ( 76.78752705046289861, 0.000000000000000000, -7.949999999999998401 ) ) ;
#142150=CARTESIAN_POINT ( 'NONE',  ( 98.70833333333332860, -3.974999999999999201, -6.884901960086287964 ) ) ;
#142170=CARTESIAN_POINT ( 'NONE',  ( 31.87086038379621655, 6.884901960086289741, -3.974999999999993427 ) ) ;
#142175=CARTESIAN_POINT ( 'NONE',  ( 26.22916666666666075, 7.950000000000001954, -2.130196079827421762 ) ) ;
#142184=CARTESIAN_POINT ( 'NONE',  ( 127.6620968585647802, -5.291415217122919401, 3.054999999999997939 ) ) ;
#142194=CARTESIAN_POINT ( 'NONE',  ( 44.04209685856477563, 5.291415217122923842, -3.054999999999996163 ) ) ;
#142203=CARTESIAN_POINT ( 'NONE',  ( 40.45376352523144448, -6.109999999999998543, -3.741295971395162543E-16 ) ) ;
#142235=CARTESIAN_POINT ( 'NONE',  ( 58.09959685856477307, -6.109999999999997655, -1.637169565754160283 ) ) ;
#142269=CARTESIAN_POINT ( 'NONE',  ( 118.7662635252314516, 4.472830434245839371, -4.472830434245839371 ) ) ;
#142278=CARTESIAN_POINT ( 'NONE',  ( 76.78752705046289861, 0.000000000000000000, -7.949999999999998401 ) ) ;
#142284=CARTESIAN_POINT ( 'NONE',  ( 0.000000000000000000, 0.000000000000000000, 7.950000000000000178 ) ) ;
#142291=ORIENTED_EDGE ( 'NONE', *, *, #141103, .T. ) ;
#142309=CARTESIAN_POINT ( 'NONE',  ( 33.16209685856478018, -5.291415217122919401, 3.054999999999998384 ) ) ;
#142334=CARTESIAN_POINT ( 'NONE',  ( 55.05836038379620589, -7.949999999999997513, -2.130196079827425759 ) ) ;
#142338=CARTESIAN_POINT ( 'NONE',  ( 50.72916666666665719, 7.950000000000001954, -2.130196079827421762 ) ) ;
#142347=CARTESIAN_POINT ( 'NONE',  ( 49.87543019189810423, -5.291415217122920289, -3.055000000000001492 ) ) ;
#142359=CARTESIAN_POINT ( 'NONE',  ( 79.47959685856477563, 6.109999999999999432, 1.637169565754164280 ) ) ;
#142368=CARTESIAN_POINT ( 'NONE',  ( 62.76626352523144448, 4.472830434245839371, -4.472830434245838482 ) ) ;
#142378=ORIENTED_EDGE ( 'NONE', *, *, #61238, .F. ) ;
#142403=CARTESIAN_POINT ( 'NONE',  ( 80.26626352523145158, 4.472830434245838482, -4.472830434245837594 ) ) ;
#142425=CARTESIAN_POINT ( 'NONE',  ( 34.27126352523143993, 4.472830434245838482, 4.472830434245842035 ) ) ;
#142459=VERTEX_POINT ( 'NONE', #95794 ) ;
#142467=LINE ( 'NONE', #31556, #42078 ) ;
#142475=CARTESIAN_POINT ( 'NONE',  ( 70.05793019189812298, 6.110000000000001208, -1.637169565754156286 ) ) ;
#142497=ORIENTED_EDGE ( 'NONE', *, *, #63442, .F. ) ;
#142503=CARTESIAN_POINT ( 'NONE',  ( 82.32919371712955581, -3.975000000000001865, 6.884901960086284411 ) ) ;
#142508=CARTESIAN_POINT ( 'NONE',  ( 85.58333333333332860, 6.884901960086290629, -3.974999999999994316 ) ) ;
#142511=CARTESIAN_POINT ( 'NONE',  ( 0.000000000000000000, 0.000000000000000000, 0.000000000000000000 ) ) ;
#142519=CARTESIAN_POINT ( 'NONE',  ( 79.04209685856477563, 5.291415217122923842, -3.054999999999996163 ) ) ;
#142527=CARTESIAN_POINT ( 'NONE',  ( 125.5000000000000000, 0.000000000000000000, 0.000000000000000000 ) ) ;
#142530=EDGE_LOOP ( 'NONE', ( #27306, #132931, #77989, #36193 ) ) ;
#142538=CARTESIAN_POINT ( 'NONE',  ( 64.02126352523144703, -4.472830434245839371, -4.472830434245840259 ) ) ;
#142568=EDGE_LOOP ( 'NONE', ( #74427, #124909, #11062, #26809 ) ) ;
#142569=CARTESIAN_POINT ( 'NONE',  ( 108.4120968585647944, 5.291415217122921177, -3.054999999999994831 ) ) ;
#142590=CARTESIAN_POINT ( 'NONE',  ( 65.47959685856477563, 6.109999999999999432, 1.637169565754164280 ) ) ;
#142597=CARTESIAN_POINT ( 'NONE',  ( 104.1254301918981184, 5.291415217122919401, 3.055000000000002824 ) ) ;
#142613=CARTESIAN_POINT ( 'NONE',  ( 125.6204301918981088, 3.055000000000001936, -5.291415217122916737 ) ) ;
#142632=CARTESIAN_POINT ( 'NONE',  ( 27.00000000000000355, 6.349999999999999645, 0.000000000000000000 ) ) ;
#142633=CARTESIAN_POINT ( 'NONE',  ( 34.12543019189810423, 5.291415217122919401, 3.055000000000002824 ) ) ;
#142639=DIRECTION ( 'NONE',  ( 0.000000000000000000, 0.000000000000000000, 1.000000000000000000 ) ) ;
#142655=CARTESIAN_POINT ( 'NONE',  ( 112.5166937171295700, 7.950000000000001066, -2.130196079827421318 ) ) ;
#142677=ADVANCED_FACE ( 'NONE', ( #102945 ), #3590, .T. ) ;
#142695=CARTESIAN_POINT ( 'NONE',  ( 91.00043019189810423, -3.055000000000002380, 5.291415217122920289 ) ) ;
#142706=CARTESIAN_POINT ( 'NONE',  ( 86.97459685856479439, 1.637169565754164058, -6.109999999999996767 ) ) ;
#142730=( BOUNDED_CURVE ( )  B_SPLINE_CURVE ( 2, ( #13304, #114754, #36513, #57577, #15429, #69898, #2421, #59034, #103186, #46735, #48116, #81476, #59717 ),
 .UNSPECIFIED., .F., .F. ) 
 B_SPLINE_CURVE_WITH_KNOTS ( ( 3, 2, 2, 2, 2, 2, 3 ),
 ( 0.08333333333332175463, 0.08611111111109912009, 0.08888888888887649942, 0.09166666666665385099, 0.09444444444443121645, 0.09722222222220859578, 0.09999999999998596123 ),
 .UNSPECIFIED. ) 
 CURVE ( )  GEOMETRIC_REPRESENTATION_ITEM ( )  RATIONAL_B_SPLINE_CURVE ( ( 1.000000000000141887, 0.9659258262889263147, 1.000000000000000000, 0.9659258262890683122, 1.000000000000000000, 0.9659258262890683122, 1.000000000000000000, 0.9659258262890683122, 1.000000000000000000, 0.9659258262890683122, 1.000000000000000000, 0.9659258262892406188, 0.9999999999998276934 ) ) 
 REPRESENTATION_ITEM ( '' )  );
#142733=CARTESIAN_POINT ( 'NONE',  ( 55.24999999999999289, -9.735942053221458872E-16, 7.950000000000000178 ) ) ;
#142757=CARTESIAN_POINT ( 'NONE',  ( 123.8129301918981042, -1.637169565754159617, -6.110000000000001208 ) ) ;
#142770=ORIENTED_EDGE ( 'NONE', *, *, #92935, .F. ) ;
#142787=CARTESIAN_POINT ( 'NONE',  ( 89.74543019189812298, -5.291415217122919401, -3.055000000000000604 ) ) ;
#142792=DIRECTION ( 'NONE',  ( 0.000000000000000000, 0.000000000000000000, 1.000000000000000000 ) ) ;
#142840=CARTESIAN_POINT ( 'NONE',  ( 97.10416666666665719, 2.130196079827422206, 7.950000000000001954 ) ) ;
#142841=ADVANCED_FACE ( 'NONE', ( #44874, #107894 ), #54996, .F. ) ;
#142860=CARTESIAN_POINT ( 'NONE',  ( 28.51669371712955225, 7.950000000000001066, -2.130196079827421318 ) ) ;
#142864=CARTESIAN_POINT ( 'NONE',  ( 116.3754301918981042, -5.291415217122920289, -3.055000000000001492 ) ) ;
#142874=CARTESIAN_POINT ( 'NONE',  ( 111.3287635252314516, 0.000000000000000000, -6.109999999999998543 ) ) ;
#142878=CARTESIAN_POINT ( 'NONE',  ( 70.80836038379624142, 7.949999999999996625, 2.130196079827431088 ) ) ;
#142884=CARTESIAN_POINT ( 'NONE',  ( 36.60459685856475431, 1.637169565754164946, -6.109999999999999432 ) ) ;
#142893=CARTESIAN_POINT ( 'NONE',  ( 38.84959685856477307, 6.109999999999996767, 1.637169565754163836 ) ) ;
#142907=EDGE_CURVE ( 'NONE', #55557, #92449, #84715, .T. ) ;
#142921=CARTESIAN_POINT ( 'NONE',  ( 46.87043019189811588, -3.055000000000001492, 5.291415217122917625 ) ) ;
#142953=CARTESIAN_POINT ( 'NONE',  ( 116.7245968585647660, -1.637169565754161171, 6.109999999999998543 ) ) ;
#142989=LINE ( 'NONE', #87184, #92357 ) ;
#143000=CARTESIAN_POINT ( 'NONE',  ( 40.89126352523144448, -4.472830434245839371, -4.472830434245839371 ) ) ;
#143004=CARTESIAN_POINT ( 'NONE',  ( 126.2708333333333286, -7.949999999999999289, -2.130196079827426203 ) ) ;
#143017=CARTESIAN_POINT ( 'NONE',  ( 120.8962635252314186, 4.472830434245840259, -4.472830434245839371 ) ) ;
#143028=CARTESIAN_POINT ( 'NONE',  ( 53.16252705046288440, 7.949999999999998401, 1.460391307983218338E-15 ) ) ;
#143034=CARTESIAN_POINT ( 'NONE',  ( 43.14583333333332860, 2.130196079827431976, -7.949999999999999289 ) ) ;
#143040=CARTESIAN_POINT ( 'NONE',  ( 46.22959685856476852, -6.110000000000000320, -1.637169565754161393 ) ) ;
#143053=CARTESIAN_POINT ( 'NONE',  ( 78.16709685856476142, -3.055000000000000160, -5.291415217122921177 ) ) ;
#143062=CARTESIAN_POINT ( 'NONE',  ( 88.01669371712955581, 7.950000000000000178, -2.130196079827421318 ) ) ;
#143063=CARTESIAN_POINT ( 'NONE',  ( 69.47459685856475176, 1.637169565754164058, -6.109999999999996767 ) ) ;
#143095=CARTESIAN_POINT ( 'NONE',  ( 73.70376352523145158, 6.109999999999998543, 1.122388791418548911E-15 ) ) ;
#143125=VERTEX_POINT ( 'NONE', #26632 ) ;
#143139=CARTESIAN_POINT ( 'NONE',  ( 109.7458603837962272, 3.974999999999996980, 6.884901960086287964 ) ) ;
#143171=CARTESIAN_POINT ( 'NONE',  ( 66.41209685856478018, 5.291415217122922066, -3.054999999999995275 ) ) ;
#143172=CARTESIAN_POINT ( 'NONE',  ( 0.000000000000000000, 0.000000000000000000, 7.950000000000000178 ) ) ;
#143175=CARTESIAN_POINT ( 'NONE',  ( 84.70833333333332860, -3.974999999999999201, -6.884901960086287964 ) ) ;
#143193=DIRECTION ( 'NONE',  ( -1.000000000000000000, -0.000000000000000000, -0.000000000000000000 ) ) ;
#143195=AXIS2_PLACEMENT_3D ( 'NONE', #25708, #60518, #71374 ) ;
#143199=CARTESIAN_POINT ( 'NONE',  ( 88.30836038379622721, 7.949999999999997513, 2.130196079827431088 ) ) ;
#143203=CARTESIAN_POINT ( 'NONE',  ( 80.33333333333334281, -6.884901960086287964, 3.974999999999998312 ) ) ;
#143213=CARTESIAN_POINT ( 'NONE',  ( 73.06293019189811844, 1.637169565754157174, 6.110000000000002984 ) ) ;
#143224=CARTESIAN_POINT ( 'NONE',  ( 127.0000000000000000, 1.564650039245123914, 6.154215649023822010 ) ) ;
#143234=CARTESIAN_POINT ( 'NONE',  ( 60.22959685856476142, -6.110000000000000320, -1.637169565754161393 ) ) ;
#143238=CARTESIAN_POINT ( 'NONE',  ( 125.0583603837962272, -7.949999999999996625, -2.130196079827426203 ) ) ;
#143261=CARTESIAN_POINT ( 'NONE',  ( 113.2245968585647802, -1.637169565754160949, 6.109999999999997655 ) ) ;
#143268=CARTESIAN_POINT ( 'NONE',  ( 68.18336038379621300, -2.130196079827426203, 7.949999999999996625 ) ) ;
#143282=VERTEX_POINT ( 'NONE', #51967 ) ;
#143288=CARTESIAN_POINT ( 'NONE',  ( 62.12543019189810423, 5.291415217122919401, 3.055000000000002824 ) ) ;
#143293=CARTESIAN_POINT ( 'NONE',  ( 98.87543019189810423, -5.291415217122920289, -3.055000000000001492 ) ) ;
#143308=CARTESIAN_POINT ( 'NONE',  ( 124.4537635252314516, -6.109999999999998543, -3.741295971395162543E-16 ) ) ;
#143329=CARTESIAN_POINT ( 'NONE',  ( 57.58333333333333570, 6.884901960086290629, -3.974999999999994316 ) ) ;
#143357=CARTESIAN_POINT ( 'NONE',  ( 116.0166937171295416, 7.950000000000001066, -2.130196079827421318 ) ) ;
#143358=DIRECTION ( 'NONE',  ( 0.000000000000000000, 0.000000000000000000, 1.000000000000000000 ) ) ;
#143400=CARTESIAN_POINT ( 'NONE',  ( 89.25043019189810423, 3.055000000000002824, -5.291415217122919401 ) ) ;
#143408=CARTESIAN_POINT ( 'NONE',  ( 150.3000000000000114, 6.349999999999997868, 0.000000000000000000 ) ) ;
#143410=CARTESIAN_POINT ( 'NONE',  ( 90.32876352523145158, 0.000000000000000000, -6.109999999999998543 ) ) ;
#143413=CARTESIAN_POINT ( 'NONE',  ( 114.7500000000000000, -9.735942053221458872E-16, 7.950000000000000178 ) ) ;
#143427=VERTEX_POINT ( 'NONE', #127189 ) ;
#143438=CARTESIAN_POINT ( 'NONE',  ( 118.8333333333333286, -6.884901960086287964, 3.974999999999998312 ) ) ;
#143442=ADVANCED_FACE ( 'NONE', ( #37346 ), #127935, .T. ) ;
#143454=CARTESIAN_POINT ( 'NONE',  ( 0.000000000000000000, 9.735942053221458872E-16, -7.950000000000000178 ) ) ;
#143456=CARTESIAN_POINT ( 'NONE',  ( 123.2295968585647756, -6.110000000000000320, -1.637169565754161393 ) ) ;
#143478=CARTESIAN_POINT ( 'NONE',  ( 127.0000000000000000, 7.950000000000000178, 0.000000000000000000 ) ) ;
#143491=CARTESIAN_POINT ( 'NONE',  ( 87.41209685856478018, 5.291415217122922066, -3.054999999999995275 ) ) ;
#143492=CARTESIAN_POINT ( 'NONE',  ( 6.404891093144800429, -9.299077053091121314, -1.947765254981038696 ) ) ;
#143543=CARTESIAN_POINT ( 'NONE',  ( 111.1041666666666714, 2.130196079827422206, 7.950000000000001954 ) ) ;
#143547=CARTESIAN_POINT ( 'NONE',  ( 101.0416666666666714, -3.975000000000002753, 6.884901960086286188 ) ) ;
ENDSEC;
END-ISO-10303-21;
